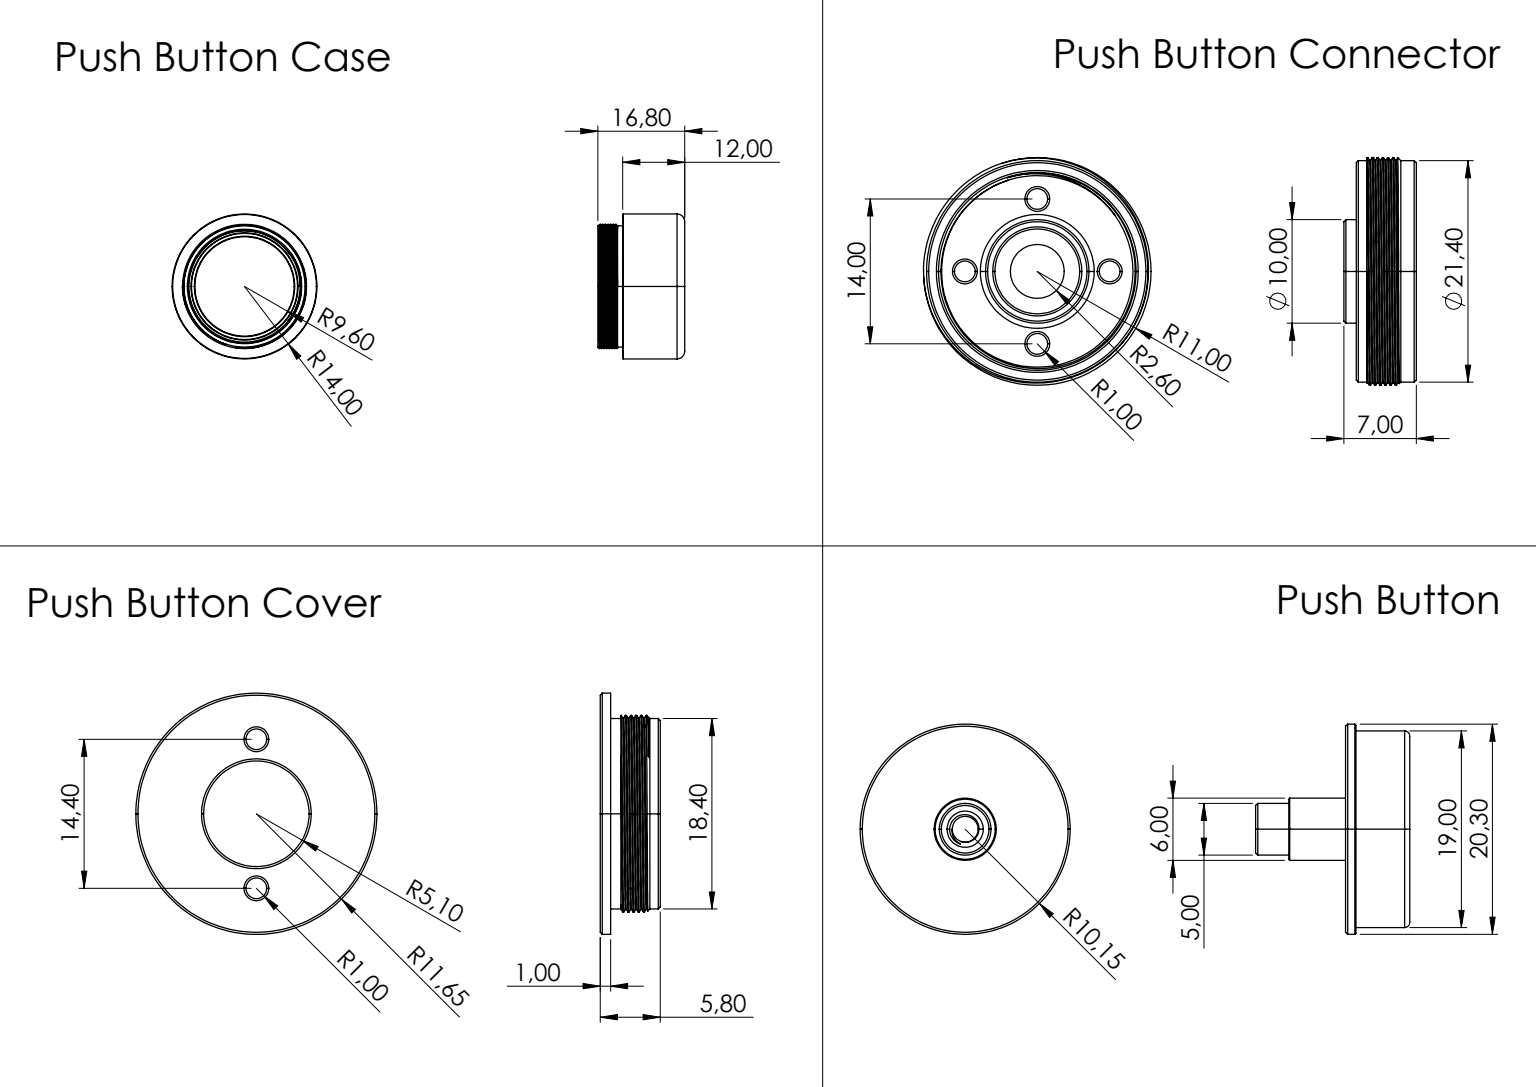
ISO-10303-21;
HEADER;
FILE_DESCRIPTION (('STEP AP214'),
    '1' );
FILE_NAME ('Push Button.step',
    '2026-10-07T19:06:49',
    ( '' ),
    ( '' ),
    'SwSTEP 2.0',
    'SolidWorks 2020',
    '' );
FILE_SCHEMA (( 'AUTOMOTIVE_DESIGN' ));
ENDSEC;

DATA;
#4=CARTESIAN_POINT ( 'NONE',  ( 1.472546342128999930, -80.60010221862999913, -0.7790162248558000213 ) ) ;
#18=CARTESIAN_POINT ( 'NONE',  ( -1.435687946562000272, -77.69186995290999675, 0.2750228405014999988 ) ) ;
#21=CARTESIAN_POINT ( 'NONE',  ( 0.06046471609518229429, -80.22932665438294464, -1.248482646815343600 ) ) ;
#44=CARTESIAN_POINT ( 'NONE',  ( -0.9806565569677715422, -83.04738115356282435, 0.7753017405169410070 ) ) ;
#48=CARTESIAN_POINT ( 'NONE',  ( 1.362316189135000188, -81.60059162671998934, -0.8114345006153000917 ) ) ;
#49=CARTESIAN_POINT ( 'NONE',  ( -1.300896064473999969, -80.54177512065000144, -0.3655689422679000433 ) ) ;
#54=CARTESIAN_POINT ( 'NONE',  ( -1.508789225394999933, -82.23555239048998544, 0.7062677124845000431 ) ) ;
#73=CARTESIAN_POINT ( 'NONE',  ( 0.8787695232493443198, -79.91340179010917666, 0.8885763300944270471 ) ) ;
#78=CARTESIAN_POINT ( 'NONE',  ( -0.5731630996927263855, -81.51327970983244597, 1.110821756836525287 ) ) ;
#88=CARTESIAN_POINT ( 'NONE',  ( -1.250000000000000000, -80.00000000000000000, 0.000000000000000000 ) ) ;
#115=CARTESIAN_POINT ( 'NONE',  ( -1.249999999999999778, -78.01041666666664298, -0.1636246173744686228 ) ) ;
#146=CARTESIAN_POINT ( 'NONE',  ( 0.000000000000000000, -86.20000000000000284, 0.000000000000000000 ) ) ;
#149=B_SPLINE_CURVE_WITH_KNOTS ( 'NONE', 3,
 ( #55404, #38266, #46279, #42423, #24107, #37685, #55701, #15248, #52939, #7198, #42935, #33761, #52652, #47672, #2489, #16927, #57077, #43805 ),
 .UNSPECIFIED., .F., .F.,
 ( 4, 2, 2, 2, 2, 2, 2, 2, 4 ),
 ( 0.000000000000000000, 0.1250000000000000833, 0.2500000000000001110, 0.3750000000000000000, 0.4999999999999999445, 0.6249999999999998890, 0.7499999999999997780, 0.8749999999999998890, 1.000000000000000000 ),
 .UNSPECIFIED. ) ;
#152=CARTESIAN_POINT ( 'NONE',  ( -0.8033051684372000123, -80.29613481679999154, -1.459438184619000101 ) ) ;
#153=CARTESIAN_POINT ( 'NONE',  ( -1.297701781740999927, -78.99170572834999859, -0.6115961818822999163 ) ) ;
#157=DIRECTION ( 'NONE',  ( 0.000000000000000000, -1.000000000000000000, 0.000000000000000000 ) ) ;
#176=CARTESIAN_POINT ( 'NONE',  ( 1.250000000000000000, -78.75000000000000000, 0.000000000000000000 ) ) ;
#186=ORIENTED_EDGE ( 'NONE', *, *, #27821, .T. ) ;
#194=B_SPLINE_CURVE_WITH_KNOTS ( 'NONE', 3,
 ( #52120, #52408, #39679, #34947 ),
 .UNSPECIFIED., .F., .F.,
 ( 4, 4 ),
 ( 0.000000000000000000, 1.000000000000000000 ),
 .UNSPECIFIED. ) ;
#195=CARTESIAN_POINT ( 'NONE',  ( -0.6515920321739999688, -80.16498426945000233, -1.183807013712999900 ) ) ;
#201=LINE ( 'NONE', #48879, #40279 ) ;
#232=DIRECTION ( 'NONE',  ( 0.000000000000000000, -1.000000000000000000, 0.000000000000000000 ) ) ;
#248=CARTESIAN_POINT ( 'NONE',  ( 0.000000000000000000, -80.69999999999998863, -2.899999999999999911 ) ) ;
#273=CARTESIAN_POINT ( 'NONE',  ( 0.1201880509156493942, -80.71773650514016651, 1.541718551563904693 ) ) ;
#282=CARTESIAN_POINT ( 'NONE',  ( 0.000000000000000000, -86.20000000000000284, 0.000000000000000000 ) ) ;
#290=CARTESIAN_POINT ( 'NONE',  ( 0.000000000000000000, -76.75499999999999545, 0.000000000000000000 ) ) ;
#316=CARTESIAN_POINT ( 'NONE',  ( 1.009608792702000102, -77.94743573086999788, -1.302912760256000224 ) ) ;
#319=CARTESIAN_POINT ( 'NONE',  ( 1.156290009273217123, -80.31913236748124518, -0.4746485085928086600 ) ) ;
#320=CARTESIAN_POINT ( 'NONE',  ( 0.3695519436384570033, -77.84114583351794181, -1.371859334843410050 ) ) ;
#333=LINE ( 'NONE', #13274, #40446 ) ;
#342=CARTESIAN_POINT ( 'NONE',  ( 1.349879140156000190, -82.67445575724998719, -0.5781647238538999423 ) ) ;
#345=CARTESIAN_POINT ( 'NONE',  ( -1.217465845835396188, -78.97916666666668561, 0.3271848554490955907 ) ) ;
#362=CARTESIAN_POINT ( 'NONE',  ( -0.2019459281704069076, -77.99218750000888178, 1.256926119276726483 ) ) ;
#368=CARTESIAN_POINT ( 'NONE',  ( -0.5212558242701900157, -81.50950461384270795, 1.136067814103569606 ) ) ;
#370=CYLINDRICAL_SURFACE ( 'NONE', #8132, 1.250000000000000000 ) ;
#371=CARTESIAN_POINT ( 'NONE',  ( -0.9788204679455345669, -81.78049098935534289, 1.151159408688467778 ) ) ;
#388=LINE ( 'NONE', #31625, #21184 ) ;
#402=CARTESIAN_POINT ( 'NONE',  ( -0.9347040216968000026, -78.69407608247999519, 1.332288049216000081 ) ) ;
#442=CARTESIAN_POINT ( 'NONE',  ( 1.520902128651999918, -80.92772696789998577, -0.6797894616744000196 ) ) ;
#443=CARTESIAN_POINT ( 'NONE',  ( 1.082149117140000172, -79.20679688847999955, 1.108446078784000033 ) ) ;
#445=CARTESIAN_POINT ( 'NONE',  ( 0.01073940206318611812, -82.87549824373742524, -1.509945108508129907 ) ) ;
#450=CARTESIAN_POINT ( 'NONE',  ( 0.8593825103163911239, -81.78595333969393266, -0.9078339653130700349 ) ) ;
#478=CARTESIAN_POINT ( 'NONE',  ( -0.5035993198763999423, -79.23880658815998856, -1.271638408173999979 ) ) ;
#513=CARTESIAN_POINT ( 'NONE',  ( -0.7681833999686477066, -82.42708333333332860, 0.9995835529977223910 ) ) ;
#515=VERTEX_POINT ( 'NONE', #57244 ) ;
#555=DIRECTION ( 'NONE',  ( 0.000000000000000000, -1.000000000000000000, 0.000000000000000000 ) ) ;
#565=CARTESIAN_POINT ( 'NONE',  ( -1.511461402894981321, -79.84725243224966107, 0.03864653979242833881 ) ) ;
#573=CARTESIAN_POINT ( 'NONE',  ( -0.5918520097389999846, -82.86672773667999081, -1.596724312065999962 ) ) ;
#595=ORIENTED_EDGE ( 'NONE', *, *, #38393, .T. ) ;
#607=CARTESIAN_POINT ( 'NONE',  ( -1.485771955761999941, -77.72682433276000324, -0.3846555688014000052 ) ) ;
#611=CARTESIAN_POINT ( 'NONE',  ( 0.8048611780553004413, -80.28119307227865420, -0.9591988868156666737 ) ) ;
#613=LINE ( 'NONE', #54606, #57976 ) ;
#632=CARTESIAN_POINT ( 'NONE',  ( 0.6959559787155999988, -82.23218377781998356, 1.424795421937999906 ) ) ;
#634=CARTESIAN_POINT ( 'NONE',  ( -0.1636246173744726473, -79.38541666666664298, 1.249999999999999112 ) ) ;
#663=DIRECTION ( 'NONE',  ( -2.716802477432000171E-13, 0.000000000000000000, 1.000000000000000000 ) ) ;
#673=CIRCLE ( 'NONE', #41223, 10.14999999999999858 ) ;
#686=ORIENTED_EDGE ( 'NONE', *, *, #25485, .T. ) ;
#693=CARTESIAN_POINT ( 'NONE',  ( -0.9347040216968000026, -78.63485975860999133, 1.332288049216000081 ) ) ;
#715=ORIENTED_EDGE ( 'NONE', *, *, #40383, .T. ) ;
#716=DIRECTION ( 'NONE',  ( -1.000000000000000000, 0.000000000000000000, 0.000000000000000000 ) ) ;
#729=CARTESIAN_POINT ( 'NONE',  ( 0.7545134501129999727, -80.60798800110998741, 1.485250302772000097 ) ) ;
#730=CARTESIAN_POINT ( 'NONE',  ( 1.315513048017999953, -78.77661456821999764, 0.1100150488083000005 ) ) ;
#732=CARTESIAN_POINT ( 'NONE',  ( 1.328728262137743421, -81.53943792409916114, 0.7184295318478360892 ) ) ;
#733=CARTESIAN_POINT ( 'NONE',  ( -1.321725462025712616, -83.30889907083121670, 0.7346322590915946860 ) ) ;
#737=CARTESIAN_POINT ( 'NONE',  ( 1.250000000000000000, -81.84999999999999432, 0.000000000000000000 ) ) ;
#741=CARTESIAN_POINT ( 'NONE',  ( 0.9995835529977264988, -80.19791666666665719, -0.7681833999686417114 ) ) ;
#768=CARTESIAN_POINT ( 'NONE',  ( -1.436931233250000162, -79.65986802222998620, -0.3027821832741999786 ) ) ;
#791=DIRECTION ( 'NONE',  ( 0.000000000000000000, -1.000000000000000000, 0.000000000000000000 ) ) ;
#794=DIRECTION ( 'NONE',  ( 0.000000000000000000, -1.000000000000000000, 0.000000000000000000 ) ) ;
#798=CARTESIAN_POINT ( 'NONE',  ( 0.3271848554490964789, -82.35416666666665719, 1.217465845835395521 ) ) ;
#818=B_SPLINE_SURFACE_WITH_KNOTS ( 'NONE', 3, 3, ( 
 ( #39006, #21856, #17146, #8578, #52308, #11864, #12432, #20715, #44020, #25714, #16866, #29841, #57878, #34561, #43740, #3858, #35133, #7424, #26565, #12713, #26288, #8000, #30425, #3572, #34847, #53164, #52878, #25428, #57304, #38715, #52593, #12143, #30131, #48180, #48457 ),
 ( #25997, #21576, #30706, #39581, #48743, #13881, #36609, #54631, #14168, #5322, #4446, #27154, #41337, #4151, #58171, #36896, #22447, #54909, #54, #17737, #18029, #36021, #25219, #43239, #9841, #26576, #58184, #12725, #44610, #35735, #21870, #22164, #35433, #39306, #30717 ),
 ( #4165, #39878, #26008, #34574, #8299, #3305, #53462, #16880, #30437, #40171, #57891, #17447, #48468, #44034, #34861, #39593, #31005, #47909, #8588, #52607, #7441, #25440, #43458, #21013, #39018, #16589, #12157, #30144, #48193, #7726, #32983, #11453, #2595, #25012, #20022 ),
 ( #15871, #33280, #10282, #55444, #14986, #46316, #32692, #6427, #6135, #51320, #15580, #24442, #10878, #38299, #29432, #11170, #29145, #47485, #47191, #51029, #5841, #56605, #42456, #20593, #33575, #43033, #38006, #42162, #24142, #23847, #51614, #19432, #10578, #2024, #56031 ) ),
 .UNSPECIFIED., .F., .F., .F.,
 ( 4, 4 ),
 ( 4, 1, 1, 1, 1, 1, 1, 1, 1, 1, 1, 1, 1, 1, 1, 1, 1, 1, 1, 1, 1, 1, 1, 1, 1, 1, 1, 1, 1, 1, 1, 1, 4 ),
 ( -0.3882448580381000491, 1.388244858038000018 ),
 ( -0.02000000000000000042, 0.01250000000000000069, 0.04499999999999999833, 0.07749999999999999944, 0.1100000000000000006, 0.1424999999999999878, 0.1749999999999999889, 0.2074999999999999900, 0.2399999999999999911, 0.2725000000000000200, 0.3049999999999999933, 0.3375000000000000222, 0.3699999999999999956, 0.4025000000000000244, 0.4349999999999999978, 0.4675000000000000266, 0.5000000000000000000, 0.5324999999999999734, 0.5649999999999999467, 0.5975000000000000311, 0.6300000000000000044, 0.6624999999999999778, 0.6949999999999999512, 0.7275000000000000355, 0.7600000000000000089, 0.7924999999999999822, 0.8249999999999999556, 0.8575000000000000400, 0.8900000000000000133, 0.9224999999999999867, 0.9549999999999999600, 0.9875000000000000444, 1.020000000000000018 ),
 .UNSPECIFIED. ) ;
#820=CARTESIAN_POINT ( 'NONE',  ( 0.8847132563061232968, -82.78824692404089092, -0.8824945250560863874 ) ) ;
#840=CARTESIAN_POINT ( 'NONE',  ( 0.1762382865323051384, -79.63606589178333195, -1.250387681160788134 ) ) ;
#848=CARTESIAN_POINT ( 'NONE',  ( -0.4056890888208716794, -79.74603335400661308, 1.458054600993641259 ) ) ;
#856=CARTESIAN_POINT ( 'NONE',  ( 1.606311393998999915, -82.99304616690000103, -0.5653197666394998988 ) ) ;
#874=CARTESIAN_POINT ( 'NONE',  ( 1.249565383984963862, -80.84028809121133463, -0.1639645281534745924 ) ) ;
#889=CARTESIAN_POINT ( 'NONE',  ( -1.113811846534999983, -78.14627689099999941, 1.056031667973999832 ) ) ;
#894=CARTESIAN_POINT ( 'NONE',  ( -0.8733059116898821417, -80.16394694085556694, -0.8939094887366128006 ) ) ;
#898=CARTESIAN_POINT ( 'NONE',  ( 0.4567011726104230895, -78.99889090922864909, -1.468873967789304125 ) ) ;
#916=CARTESIAN_POINT ( 'NONE',  ( -0.3643839585117999991, -81.91670264959000747, 1.301227969886000091 ) ) ;
#917=CARTESIAN_POINT ( 'NONE',  ( -1.322249586278000155, -80.03650139976998901, -0.2786171024073000324 ) ) ;
#935=CARTESIAN_POINT ( 'NONE',  ( 0.1759108568145950069, -79.23653620316339641, -1.251611073654840034 ) ) ;
#945=CARTESIAN_POINT ( 'NONE',  ( -1.173001147021014212, -81.57218295784426232, 0.4318201719082435108 ) ) ;
#949=CARTESIAN_POINT ( 'NONE',  ( -0.9491653955992001013, -78.01964351345999660, 0.8999264274451000967 ) ) ;
#950=B_SPLINE_CURVE_WITH_KNOTS ( 'NONE', 3,
 ( #46073, #45780, #6184, #14456, #37471, #23607, #15041, #51080, #28612, #20350, #48379, #16211, #43654, #11783, #39207, #57222, #25631, #7630, #34479, #15919, #48098, #25060, #3214, #20919, #33904, #38920, #7060, #47535, #51946, #16787, #56655, #51666, #56938, #38638, #29756, #11503, #30047, #21202, #38060, #29476, #43084, #11213, #3492, #47813, #25918, #16498, #7917, #43358, #2642, #34770, #52510, #12066, #52794, #12349, #38347, #29191, #56081, #7344, #43941, #30336, #15627, #24778, #33622, #47239, #6769, #20635, #42791, #2354, #56368, #34188, #2919, #52226, #25343, #16064, #11355, #29621, #10475, #10775, #29051, #25203, #37617, #46509, #2778, #51511, #28753, #33474, #15186, #38778, #43222, #42644, #2210, #55634, #42058, #47090, #19919, #42356, #15484, #32884, #1924, #29333, #37909, #20777, #14886, #11643, #6034, #55933, #33176 ),
 .UNSPECIFIED., .F., .F.,
 ( 4, 2, 2, 2, 2, 2, 1, 2, 2, 2, 2, 2, 2, 2, 2, 2, 2, 2, 2, 2, 2, 2, 2, 2, 2, 2, 2, 1, 2, 2, 2, 2, 2, 2, 2, 2, 2, 2, 2, 2, 2, 2, 2, 2, 2, 2, 2, 2, 1, 2, 2, 2, 2, 2, 4 ),
 ( 0.000000000000000000, 0.01562500000000001388, 0.03125000000000003469, 0.04687500000000005551, 0.06250000000000008327, 0.07812500000000009714, 0.09375000000000011102, 0.1093750000000001249, 0.1250000000000001388, 0.1406250000000001110, 0.1562500000000001110, 0.1718750000000000833, 0.1875000000000000833, 0.2031250000000000833, 0.2187500000000001110, 0.2343750000000001110, 0.2500000000000001110, 0.2656250000000001110, 0.2812500000000001110, 0.2968750000000001665, 0.3125000000000001665, 0.3281250000000001665, 0.3437500000000001665, 0.3750000000000001665, 0.4062500000000001110, 0.4375000000000001110, 0.4687500000000000555, 0.5000000000000000000, 0.5312500000000000000, 0.5624999999999998890, 0.5937499999999998890, 0.6249999999999997780, 0.6562499999999997780, 0.6718749999999997780, 0.6874999999999997780, 0.7031249999999998890, 0.7187499999999998890, 0.7343749999999998890, 0.7499999999999998890, 0.7656249999999998890, 0.7812499999999998890, 0.7968749999999998890, 0.8124999999999998890, 0.8281250000000000000, 0.8437500000000000000, 0.8593750000000000000, 0.8750000000000000000, 0.8906250000000000000, 0.9062500000000000000, 0.9218750000000000000, 0.9375000000000000000, 0.9531250000000001110, 0.9687500000000001110, 0.9843750000000001110, 1.000000000000000000 ),
 .UNSPECIFIED. ) ;
#959=ORIENTED_EDGE ( 'NONE', *, *, #25485, .F. ) ;
#978=CARTESIAN_POINT ( 'NONE',  ( 0.4326115402657000342, -78.91680236158998696, -1.568920109259999807 ) ) ;
#1016=ADVANCED_FACE ( 'NONE', ( #23425 ), #43407, .T. ) ;
#1018=CARTESIAN_POINT ( 'NONE',  ( -0.8981901762082999952, -79.79086109591999332, -1.403037214508999986 ) ) ;
#1019=CARTESIAN_POINT ( 'NONE',  ( 0.06763567127574998672, -79.64895916143998988, -1.247532485737999908 ) ) ;
#1021=CARTESIAN_POINT ( 'NONE',  ( 0.6046126565052558632, -81.40785622595326743, -1.385375599882785025 ) ) ;
#1026=CARTESIAN_POINT ( 'NONE',  ( -0.8193159871064622513, -81.66856760969551488, -0.9439107478074511004 ) ) ;
#1027=( NAMED_UNIT ( * ) SI_UNIT ( $, .STERADIAN. ) SOLID_ANGLE_UNIT ( ) );
#1048=AXIS2_PLACEMENT_3D ( 'NONE', #52317, #57594, #33995 ) ;
#1053=CARTESIAN_POINT ( 'NONE',  ( 0.6229729438976999711, -81.04952822830999537, 1.458184003450999855 ) ) ;
#1064=CARTESIAN_POINT ( 'NONE',  ( -1.250000000000000000, -79.00000000000000000, 0.000000000000000000 ) ) ;
#1087=CARTESIAN_POINT ( 'NONE',  ( -1.092232985442822102, -82.54166666666664298, -0.6295237254636245616 ) ) ;
#1093=ORIENTED_EDGE ( 'NONE', *, *, #15590, .T. ) ;
#1107=CARTESIAN_POINT ( 'NONE',  ( 1.228744581380641687, -82.83562427784806914, -0.2287525698557267839 ) ) ;
#1126=CARTESIAN_POINT ( 'NONE',  ( -0.4851089960429650905, -83.00678479282305489, 1.152015161174709146 ) ) ;
#1133=CARTESIAN_POINT ( 'NONE',  ( 0.1624548541070857943, -79.48286375057362818, -1.504788102669172734 ) ) ;
#1180=CARTESIAN_POINT ( 'NONE',  ( -1.190204951956445267, -80.12538959866201083, -0.3913796594779095916 ) ) ;
#1184=CARTESIAN_POINT ( 'NONE',  ( -0.7887420553019258707, -78.26716755245251989, 1.320791577295096442 ) ) ;
#1194=DIRECTION ( 'NONE',  ( -1.000000000000000000, 0.000000000000000000, 0.000000000000000000 ) ) ;
#1199=CARTESIAN_POINT ( 'NONE',  ( 0.4274279416557000277, -83.36936459712099179, 1.281884980902999960 ) ) ;
#1209=CARTESIAN_POINT ( 'NONE',  ( -1.288646058034000008, -83.05573296103600001, 0.4058063692239000098 ) ) ;
#1212=CARTESIAN_POINT ( 'NONE',  ( 1.343749999883000035, -77.90625000011999646, 3.156563468101999814E-09 ) ) ;
#1220=CARTESIAN_POINT ( 'NONE',  ( 1.062167859419960614, -79.30478719906479057, -0.6841706396682687430 ) ) ;
#1225=CARTESIAN_POINT ( 'NONE',  ( -2.299999999264999762, -77.49999999927000260, -2.080610052828999912E-10 ) ) ;
#1229=CARTESIAN_POINT ( 'NONE',  ( -1.143190144809757669, -81.56692634864619151, 0.5063306831769307514 ) ) ;
#1234=CARTESIAN_POINT ( 'NONE',  ( -1.280405559996000031, -78.59639078104000021, -0.2671032044805999872 ) ) ;
#1263=CARTESIAN_POINT ( 'NONE',  ( 1.341343219651000229, -78.97248393136999312, -0.9216622887798999741 ) ) ;
#1271=CARTESIAN_POINT ( 'NONE',  ( -0.9334586162929999764, -81.40447863951000329, -1.282259494539000011 ) ) ;
#1298=CARTESIAN_POINT ( 'NONE',  ( 1.640574411872000038, -79.59349766811000393, 0.2893137654249999802 ) ) ;
#1301=CARTESIAN_POINT ( 'NONE',  ( -0.1061383120418225301, -81.63053294589249731, 1.507463295298500761 ) ) ;
#1309=CARTESIAN_POINT ( 'NONE',  ( -0.5392730711932351984, -81.68971611294774959, -1.130938875651418929 ) ) ;
#1319=CARTESIAN_POINT ( 'NONE',  ( -1.447950951198242908, -77.76302083339091098, -0.3900009942188623069 ) ) ;
#1335=CARTESIAN_POINT ( 'NONE',  ( -1.125831293927000099, -79.53339211834999389, 0.7473110439769999891 ) ) ;
#1390=CARTESIAN_POINT ( 'NONE',  ( 1.179782483562120010, -82.82318035081991070, -0.4135125750267664158 ) ) ;
#1410=DIRECTION ( 'NONE',  ( 0.000000000000000000, -1.000000000000000000, 0.000000000000000000 ) ) ;
#1415=CARTESIAN_POINT ( 'NONE',  ( 1.136635571591867233, -82.88416972722252751, 0.5202534302794125098 ) ) ;
#1417=DIRECTION ( 'NONE',  ( -1.000000000000000000, 0.000000000000000000, 0.000000000000000000 ) ) ;
#1421=CONICAL_SURFACE ( 'NONE', #16485, 1.546875000130000011, 0.7853981633972997312 ) ;
#1450=CARTESIAN_POINT ( 'NONE',  ( -0.2327570447753271599, -80.71078059628793255, -1.249194938801351462 ) ) ;
#1469=CARTESIAN_POINT ( 'NONE',  ( -0.4548846362379543873, -80.19556477582571574, -1.164187075856578879 ) ) ;
#1473=CARTESIAN_POINT ( 'NONE',  ( 0.7757320150892573762, -78.51702430842580327, -1.327015570253983867 ) ) ;
#1475=VERTEX_POINT ( 'NONE', #10794 ) ;
#1491=CARTESIAN_POINT ( 'NONE',  ( -0.3271848554491046945, -78.89583333333328596, 1.217465845835393301 ) ) ;
#1515=CARTESIAN_POINT ( 'NONE',  ( 1.137232763453390971, -81.38436038258944905, 0.5186267222472648042 ) ) ;
#1547=CARTESIAN_POINT ( 'NONE',  ( -0.6580604922749000441, -79.48068756757000131, -1.488334326434000099 ) ) ;
#1555=CARTESIAN_POINT ( 'NONE',  ( -1.478021081765000133, -80.28866583923000633, 0.8457367421919999018 ) ) ;
#1586=CARTESIAN_POINT ( 'NONE',  ( 1.520902128651999918, -81.04615961563999349, -0.6797894616744000196 ) ) ;
#1587=CARTESIAN_POINT ( 'NONE',  ( -0.7899273271878000102, -77.87807433275999358, 1.197381041534999913 ) ) ;
#1592=CARTESIAN_POINT ( 'NONE',  ( 1.008924559857650838, -79.79982627189708921, -0.7395781483535016632 ) ) ;
#1595=CARTESIAN_POINT ( 'NONE',  ( -0.6881529071261847097, -81.67893781361996730, -1.045368128735210345 ) ) ;
#1598=EDGE_LOOP ( 'NONE', ( #30301, #26182, #32852, #20081 ) ) ;
#1605=DIRECTION ( 'NONE',  ( 0.000000000000000000, 1.000000000000000000, 0.000000000000000000 ) ) ;
#1625=CARTESIAN_POINT ( 'NONE',  ( -0.4634070002434999558, -79.17548989939000137, -1.170148800580000037 ) ) ;
#1646=CARTESIAN_POINT ( 'NONE',  ( 0.1128515190273495367, -78.46792679642489077, 1.249931857778512345 ) ) ;
#1651=ADVANCED_FACE ( 'NONE', ( #6935 ), #57395, .F. ) ;
#1668=CARTESIAN_POINT ( 'NONE',  ( 0.7677661701836960839, -78.27713689064573543, -0.9989898656190768778 ) ) ;
#1669=CARTESIAN_POINT ( 'NONE',  ( 0.000000000000000000, -87.15000000002500258, 0.000000000000000000 ) ) ;
#1683=ORIENTED_EDGE ( 'NONE', *, *, #42399, .F. ) ;
#1684=CARTESIAN_POINT ( 'NONE',  ( -1.249681228189473803, -79.59559394467255800, 0.07758196913156252539 ) ) ;
#1685=CARTESIAN_POINT ( 'NONE',  ( -0.6712347860653230525, -78.16172226271685020, 1.350201467282728274 ) ) ;
#1703=CARTESIAN_POINT ( 'NONE',  ( 0.4639973262319513347, -82.94477574862143854, 1.160677889351085623 ) ) ;
#1715=CARTESIAN_POINT ( 'NONE',  ( 1.092232985442823212, -80.70833333333331439, -0.6295237254636224522 ) ) ;
#1745=CARTESIAN_POINT ( 'NONE',  ( -1.009397235748368260, -81.20718188826208461, -0.8706472256294847112 ) ) ;
#1760=CARTESIAN_POINT ( 'NONE',  ( -0.5573453952815472512, -80.18842898730592594, -1.122125656035228625 ) ) ;
#1764=CARTESIAN_POINT ( 'NONE',  ( 1.505383061368419151, -79.10597237606836529, 0.1212336400873940262 ) ) ;
#1779=CARTESIAN_POINT ( 'NONE',  ( -0.6142531002814000107, -83.43252381223099690, 1.203711489715000305 ) ) ;
#1789=CARTESIAN_POINT ( 'NONE',  ( -0.5525270872808000222, -82.17150394948998837, -1.233160589678000019 ) ) ;
#1791=ADVANCED_FACE ( 'NONE', ( #35516 ), #44242, .T. ) ;
#1808=CARTESIAN_POINT ( 'NONE',  ( 0.9748194815771379362, -81.40464457030101642, 0.7859197306878139555 ) ) ;
#1813=CARTESIAN_POINT ( 'NONE',  ( 0.05227849266716000365, -79.20809242846999609, -1.244609249457999889 ) ) ;
#1843=CARTESIAN_POINT ( 'NONE',  ( -0.06603165175717734536, -81.62109302337999850, -1.273657571949194489 ) ) ;
#1844=CARTESIAN_POINT ( 'NONE',  ( 0.1660104325307999729, -78.25569303241999819, 1.618982269915999916 ) ) ;
#1852=FACE_OUTER_BOUND ( 'NONE', #12679, .T. ) ;
#1864=ORIENTED_EDGE ( 'NONE', *, *, #30051, .T. ) ;
#1877=CARTESIAN_POINT ( 'NONE',  ( -0.4900037880837543325, -80.00730615406503432, 1.149793150307434342 ) ) ;
#1881=EDGE_CURVE ( 'NONE', #7116, #37205, #34789, .T. ) ;
#1883=CARTESIAN_POINT ( 'NONE',  ( 1.417725061834000044, -79.97639585000999318, -0.8748226493128999914 ) ) ;
#1884=CARTESIAN_POINT ( 'NONE',  ( -1.375650254229000113, -77.93375590253999974, 0.4072090767667999600 ) ) ;
#1886=CARTESIAN_POINT ( 'NONE',  ( 1.076979181859827106, -81.43822123321770334, -1.059161443897362664 ) ) ;
#1888=LINE ( 'NONE', #10740, #54428 ) ;
#1893=CARTESIAN_POINT ( 'NONE',  ( -0.4068589336182526495, -81.69886620421327450, -1.181800740598763166 ) ) ;
#1896=CARTESIAN_POINT ( 'NONE',  ( -1.249999999999999778, -80.01041666666664298, -0.1636246173744686228 ) ) ;
#1903=CARTESIAN_POINT ( 'NONE',  ( 1.250000000000000000, -80.74999999999998579, 0.000000000000000000 ) ) ;
#1908=CARTESIAN_POINT ( 'NONE',  ( 1.343749999883000035, -77.90625000011999646, 3.156563468101999814E-09 ) ) ;
#1920=CARTESIAN_POINT ( 'NONE',  ( 1.676986109946000170, -79.53386453932999700, 0.2957349343760000138 ) ) ;
#1924=CARTESIAN_POINT ( 'NONE',  ( 1.434073767539737476, -79.47461743011145074, -0.4734074842604066302 ) ) ;
#1940=CARTESIAN_POINT ( 'NONE',  ( 0.7924526256690966886, -78.42054099154100300, 0.9668092435737775103 ) ) ;
#1966=DIRECTION ( 'NONE',  ( 1.040437577282999923E-11, 1.000000000000000000, -2.038011343141999906E-09 ) ) ;
#1978=CARTESIAN_POINT ( 'NONE',  ( -0.6292794791536331367, -82.68371027185608568, -1.092639821175960479 ) ) ;
#1979=ORIENTED_EDGE ( 'NONE', *, *, #58164, .T. ) ;
#1983=CARTESIAN_POINT ( 'NONE',  ( 0.7149329466314869874, -78.08609980630498626, 1.354438294650810892 ) ) ;
#2002=CARTESIAN_POINT ( 'NONE',  ( 0.9590251478797268136, -82.90587166377093808, 0.8014916951292889724 ) ) ;
#2024=CARTESIAN_POINT ( 'NONE',  ( -1.374853770045000090, -81.42764988327999731, -0.7192078502473999713 ) ) ;
#2041=CARTESIAN_POINT ( 'NONE',  ( -0.04600636030614828342, -80.47847291610720788, 1.248880407862982711 ) ) ;
#2058=CARTESIAN_POINT ( 'NONE',  ( -1.279096942007310611, -78.80257488668075894, 0.8515545081673395744 ) ) ;
#2071=CARTESIAN_POINT ( 'NONE',  ( -0.6329778402533998705, -82.10618029491999437, -1.193863583722999833 ) ) ;
#2099=CARTESIAN_POINT ( 'NONE',  ( -0.003982218678106667215, -81.47577399763491712, 1.249684034757714279 ) ) ;
#2101=CARTESIAN_POINT ( 'NONE',  ( 1.093387357835452933, -82.30899171049304641, -0.6298603018139183884 ) ) ;
#2103=CARTESIAN_POINT ( 'NONE',  ( 0.0004826309679763999953, -77.70505409477999592, -1.307959744758000031 ) ) ;
#2107=ORIENTED_EDGE ( 'NONE', *, *, #50023, .T. ) ;
#2108=ORIENTED_EDGE ( 'NONE', *, *, #13353, .T. ) ;
#2130=CARTESIAN_POINT ( 'NONE',  ( 0.08338359222296000406, -79.51780861409000067, -1.538001148114999994 ) ) ;
#2139=CARTESIAN_POINT ( 'NONE',  ( 1.653747448240000084, -80.09918819389999101, 0.4061235413877000155 ) ) ;
#2166=CARTESIAN_POINT ( 'NONE',  ( -0.9620943986040956242, -80.04521171774420907, 0.7983770923343646020 ) ) ;
#2172=FACE_OUTER_BOUND ( 'NONE', #45792, .T. ) ;
#2174=CARTESIAN_POINT ( 'NONE',  ( 1.052209778380920779, -83.03560755957414585, -1.084595603600321256 ) ) ;
#2175=CARTESIAN_POINT ( 'NONE',  ( -1.249989095222701962, -79.61143095040115725, -0.1792705600110044706 ) ) ;
#2178=CARTESIAN_POINT ( 'NONE',  ( -0.7575910999740240737, -81.67355912156841669, -0.9946733871216205669 ) ) ;
#2180=( LENGTH_UNIT ( ) NAMED_UNIT ( * ) SI_UNIT ( .MILLI., .METRE. ) );
#2195=DIRECTION ( 'NONE',  ( 0.7071067811865474617, 0.7071067811865474617, -7.240421654463485624E-10 ) ) ;
#2198=ORIENTED_EDGE ( 'NONE', *, *, #38015, .F. ) ;
#2204=CARTESIAN_POINT ( 'NONE',  ( 1.217465845835393967, -79.77083333333330017, 0.3271848554491025851 ) ) ;
#2206=CARTESIAN_POINT ( 'NONE',  ( 0.8102226603197999477, -80.03898078654999892, 1.363061245571999924 ) ) ;
#2210=CARTESIAN_POINT ( 'NONE',  ( 0.1655257079421880717, -79.61632079734550871, 1.501053824981346763 ) ) ;
#2214=LINE ( 'NONE', #38204, #7077 ) ;
#2224=CARTESIAN_POINT ( 'NONE',  ( 0.8397211166896187962, -78.41649201275657788, 0.9258721447709178376 ) ) ;
#2245=CARTESIAN_POINT ( 'NONE',  ( 0.000000000000000000, -77.69999999999998863, 0.000000000000000000 ) ) ;
#2259=CARTESIAN_POINT ( 'NONE',  ( 0.4467594448287516284, -82.75414052523781550, -1.167571400202662035 ) ) ;
#2264=CARTESIAN_POINT ( 'NONE',  ( 0.6359740846337066378, -79.43277818229616116, 1.079437290100915048 ) ) ;
#2265=CARTESIAN_POINT ( 'NONE',  ( -1.002309790681787716, -78.81711688494529255, -1.125562765835532497 ) ) ;
#2274=CARTESIAN_POINT ( 'NONE',  ( 0.9062719787061290777, -81.17322235724128632, 1.209793186763744366 ) ) ;
#2285=CARTESIAN_POINT ( 'NONE',  ( 0.2266372662724759901, -82.96071876721104843, 1.229146615866300696 ) ) ;
#2293=DIRECTION ( 'NONE',  ( 0.000000000000000000, 1.000000000000000000, 0.000000000000000000 ) ) ;
#2319=FACE_OUTER_BOUND ( 'NONE', #35834, .T. ) ;
#2325=CARTESIAN_POINT ( 'NONE',  ( -0.02507988100666198525, -80.47717407346517859, 1.249410415426445153 ) ) ;
#2328=CIRCLE ( 'NONE', #34322, 9.500000000000000000 ) ;
#2332=ORIENTED_EDGE ( 'NONE', *, *, #19355, .T. ) ;
#2341=CARTESIAN_POINT ( 'NONE',  ( -1.478853428237032475, -77.86561205178121270, -0.3007429780463568014 ) ) ;
#2342=ADVANCED_FACE ( 'NONE', ( #58194 ), #8600, .F. ) ;
#2354=CARTESIAN_POINT ( 'NONE',  ( 1.329440977735876661, -79.96045754634249647, -0.7203538468090995295 ) ) ;
#2384=CARTESIAN_POINT ( 'NONE',  ( 1.146081193082048033, -81.38292660934976652, 0.4986479518160068514 ) ) ;
#2392=ORIENTED_EDGE ( 'NONE', *, *, #3092, .T. ) ;
#2406=ORIENTED_EDGE ( 'NONE', *, *, #22775, .F. ) ;
#2415=CARTESIAN_POINT ( 'NONE',  ( 0.1742577344548000007, -77.75455890439999962, 1.489843697164999980 ) ) ;
#2422=CARTESIAN_POINT ( 'NONE',  ( -1.586699731716999962, -82.80045924015399805, 0.6182239771991999699 ) ) ;
#2423=CARTESIAN_POINT ( 'NONE',  ( -1.639384890095999969, -80.35182505433999722, -0.4606887641594999971 ) ) ;
#2431=CARTESIAN_POINT ( 'NONE',  ( -0.8302729325563608098, -81.16825566421603355, -0.9509483969845207163 ) ) ;
#2458=CARTESIAN_POINT ( 'NONE',  ( -0.1835247799291997717, -82.96475420480349783, -1.500792295550013478 ) ) ;
#2488=CARTESIAN_POINT ( 'NONE',  ( -0.9334586162929999764, -81.34442870581999330, -1.282259494539000011 ) ) ;
#2489=CARTESIAN_POINT ( 'NONE',  ( -1.092232985442822102, -81.04166666666664298, -0.6295237254636245616 ) ) ;
#2528=FACE_BOUND ( 'NONE', #24499, .T. ) ;
#2530=CARTESIAN_POINT ( 'NONE',  ( -0.3271848554491046945, -81.89583333333330017, 1.217465845835393301 ) ) ;
#2544=CARTESIAN_POINT ( 'NONE',  ( 0.7945685312060931649, -82.78032265392057809, -0.9647621081858361869 ) ) ;
#2548=CARTESIAN_POINT ( 'NONE',  ( 0.8360307752442982521, -79.41690561761365075, 0.9295092197899607056 ) ) ;
#2549=CARTESIAN_POINT ( 'NONE',  ( -0.9591330678447479441, -78.32136967069745026, -1.194087134926961946 ) ) ;
#2558=CARTESIAN_POINT ( 'NONE',  ( -1.480668258985768482, -81.36553860590423426, -0.3070248522480592546 ) ) ;
#2595=CARTESIAN_POINT ( 'NONE',  ( -0.8762103189736000219, -81.41053970282000307, -1.416501064863000092 ) ) ;
#2607=ORIENTED_EDGE ( 'NONE', *, *, #55721, .F. ) ;
#2611=EDGE_LOOP ( 'NONE', ( #45072, #3068, #21608, #2789, #31112, #29819 ) ) ;
#2612=CARTESIAN_POINT ( 'NONE',  ( -0.06320921880059908460, -80.47953876087936465, 1.248225759446036864 ) ) ;
#2629=CARTESIAN_POINT ( 'NONE',  ( -1.250000000000000000, -83.09999999999999432, 0.000000000000000000 ) ) ;
#2642=CARTESIAN_POINT ( 'NONE',  ( 1.545086291967713299, -80.49690600801427820, -0.05127199417640600221 ) ) ;
#2652=CARTESIAN_POINT ( 'NONE',  ( 0.6735630312197999903, -82.86657026302199824, -1.435516540950999786 ) ) ;
#2670=CARTESIAN_POINT ( 'NONE',  ( 0.6793202165550557003, -81.42948271688828754, 1.050371840538202539 ) ) ;
#2673=CARTESIAN_POINT ( 'NONE',  ( 0.000000000000000000, -87.15000000002500258, 0.000000000000000000 ) ) ;
#2706=DIRECTION ( 'NONE',  ( -1.000000000000000000, 0.000000000000000000, 0.000000000000000000 ) ) ;
#2707=CARTESIAN_POINT ( 'NONE',  ( -1.566959183383000109, -78.36705617198001050, 0.4396611996733000294 ) ) ;
#2713=CARTESIAN_POINT ( 'NONE',  ( 0.4046438523804999909, -81.47411572283999703, -1.654233492563000008 ) ) ;
#2714=CARTESIAN_POINT ( 'NONE',  ( -0.7407245532275998912, -81.59442870581999330, -1.017507444502999903 ) ) ;
#2733=CARTESIAN_POINT ( 'NONE',  ( -1.440962122118119471, -79.37367604318139058, -0.4505052090234867301 ) ) ;
#2739=CARTESIAN_POINT ( 'NONE',  ( -1.250000000000000000, -80.09999999999999432, 0.000000000000000000 ) ) ;
#2745=CARTESIAN_POINT ( 'NONE',  ( 0.4264742922811849413, -82.70158460137095346, 1.451405935591948637 ) ) ;
#2746=CARTESIAN_POINT ( 'NONE',  ( -0.9383909286133819139, -79.65811737660978054, -0.8288992896692728429 ) ) ;
#2754=ORIENTED_EDGE ( 'NONE', *, *, #48627, .T. ) ;
#2755=VERTEX_POINT ( 'NONE', #44119 ) ;
#2776=CARTESIAN_POINT ( 'NONE',  ( -1.526555281555000088, -80.22845843187998582, -0.4289821568622999570 ) ) ;
#2778=CARTESIAN_POINT ( 'NONE',  ( -1.492020074518721318, -79.73778082640328080, 0.2322189972777134459 ) ) ;
#2789=ORIENTED_EDGE ( 'NONE', *, *, #23705, .F. ) ;
#2798=AXIS2_PLACEMENT_3D ( 'NONE', #33784, #43246, #16954 ) ;
#2810=CARTESIAN_POINT ( 'NONE',  ( 1.357547920874000003, -78.53098293213999170, -0.9615626969474000418 ) ) ;
#2818=CARTESIAN_POINT ( 'NONE',  ( 0.9995835529977233902, -81.80208333333332860, 0.7681833999686461523 ) ) ;
#2834=CARTESIAN_POINT ( 'NONE',  ( -0.2254326743809463296, -78.13651477724624783, 1.514863696781568736 ) ) ;
#2891=CARTESIAN_POINT ( 'NONE',  ( -0.01891664938484899361, -80.47679111333721380, 1.249509389969930773 ) ) ;
#2911=VECTOR ( 'NONE', #51281, 1000.000000000000000 ) ;
#2919=CARTESIAN_POINT ( 'NONE',  ( 0.8074256036998892494, -79.91997086998991051, -1.276157013251583150 ) ) ;
#2928=CARTESIAN_POINT ( 'NONE',  ( 1.420454834158999979, -81.41375084182999444, 0.3724989704330000095 ) ) ;
#2947=CARTESIAN_POINT ( 'NONE',  ( -0.8033051684372000123, -80.41456746453999926, -1.459438184619000101 ) ) ;
#2951=CARTESIAN_POINT ( 'NONE',  ( -0.6299849389810197042, -82.18398283962009998, -1.093434970869878287 ) ) ;
#2988=DIRECTION ( 'NONE',  ( 1.000000000000000000, 0.000000000000000000, 2.719057617949999588E-13 ) ) ;
#2991=CARTESIAN_POINT ( 'NONE',  ( 9.500000000000000000, -91.89999999999999147, 0.000000000000000000 ) ) ;
#2997=CARTESIAN_POINT ( 'NONE',  ( -1.544355253863999966, -83.34783910444198796, -0.3612495668209000366 ) ) ;
#2999=CARTESIAN_POINT ( 'NONE',  ( 1.446151133417000079, -79.72054785055999560, 0.2550274018384999786 ) ) ;
#3008=CARTESIAN_POINT ( 'NONE',  ( -0.2863152943028942077, -81.20653045236295497, -1.221378511987871951 ) ) ;
#3013=DIRECTION ( 'NONE',  ( 0.000000000000000000, -1.000000000000000000, 0.000000000000000000 ) ) ;
#3025=CARTESIAN_POINT ( 'NONE',  ( -1.190683053189752982, -80.07578141901581148, 0.3803500925840294089 ) ) ;
#3033=CARTESIAN_POINT ( 'NONE',  ( 1.270967135966797112, -82.05378250061171741, -0.8204115018237847501 ) ) ;
#3034=CARTESIAN_POINT ( 'NONE',  ( 0.4820167300484242690, -79.75682355617291819, -1.153123235814610181 ) ) ;
#3050=SHAPE_DEFINITION_REPRESENTATION ( #24909, #33899 ) ;
#3065=CARTESIAN_POINT ( 'NONE',  ( 1.291435174072999903, -79.40738863544999049, -0.9202965842325999679 ) ) ;
#3068=ORIENTED_EDGE ( 'NONE', *, *, #54755, .F. ) ;
#3092=EDGE_CURVE ( 'NONE', #26509, #39544, #52050, .T. ) ;
#3100=CARTESIAN_POINT ( 'NONE',  ( 1.249653476780883121, -81.85243642884611859, 0.02917368571513033818 ) ) ;
#3127=CARTESIAN_POINT ( 'NONE',  ( 0.3860122406418020624, -82.75015049869273298, -1.188808172101050165 ) ) ;
#3138=CARTESIAN_POINT ( 'NONE',  ( -1.260603054430202263, -81.39590432937541209, -0.8352852932649793560 ) ) ;
#3148=CARTESIAN_POINT ( 'NONE',  ( 1.251003419626117052, -82.85390030615222656, 0.05208032629560303828 ) ) ;
#3154=DIRECTION ( 'NONE',  ( 0.000000000000000000, 1.000000000000000000, 0.000000000000000000 ) ) ;
#3188=CARTESIAN_POINT ( 'NONE',  ( 0.3239878837106308085, -80.45445633517968531, 1.207198879959141102 ) ) ;
#3207=CARTESIAN_POINT ( 'NONE',  ( -1.092232985442824100, -83.45833333333328596, 0.6295237254636200097 ) ) ;
#3214=CARTESIAN_POINT ( 'NONE',  ( 1.348353453518538192, -80.96250278606902384, -0.6851815357594489564 ) ) ;
#3224=CARTESIAN_POINT ( 'NONE',  ( -0.6256353049379000941, -82.61393340258099727, 1.457043991488000012 ) ) ;
#3227=CARTESIAN_POINT ( 'NONE',  ( -1.249999999999999778, -82.01041666666662877, -0.1636246173744686228 ) ) ;
#3237=CARTESIAN_POINT ( 'NONE',  ( 0.000000000000000000, -87.20000000000000284, 0.000000000000000000 ) ) ;
#3243=CARTESIAN_POINT ( 'NONE',  ( 0.8512149552595998925, -80.16193060409999305, 1.432023780608000063 ) ) ;
#3274=CARTESIAN_POINT ( 'NONE',  ( 1.092232985442823212, -83.20833333333330017, -0.6295237254636224522 ) ) ;
#3280=CARTESIAN_POINT ( 'NONE',  ( -1.250000000000000000, -79.10000000000000853, 0.000000000000000000 ) ) ;
#3282=CARTESIAN_POINT ( 'NONE',  ( 0.000000000000000000, -91.89999999999999147, 0.000000000000000000 ) ) ;
#3287=CARTESIAN_POINT ( 'NONE',  ( -1.438065998794000100, -83.41115579321099460, -0.3363867981957999742 ) ) ;
#3288=CARTESIAN_POINT ( 'NONE',  ( 0.4542139134408000323, -80.54146017332999463, -1.519238769708999959 ) ) ;
#3305=CARTESIAN_POINT ( 'NONE',  ( 1.496210884224999926, -83.11583851079198837, 0.7325374182646999799 ) ) ;
#3313=CARTESIAN_POINT ( 'NONE',  ( 1.105138191744446718, -79.88914713198865059, 0.5837908578609295462 ) ) ;
#3316=ADVANCED_FACE ( 'NONE', ( #53478 ), #370, .F. ) ;
#3318=CARTESIAN_POINT ( 'NONE',  ( -0.3273215601811345077, -78.99604344152334079, 1.250887209240275633 ) ) ;
#3319=CARTESIAN_POINT ( 'NONE',  ( 1.520202006809699524, -82.11451394755752631, 0.3017852963696689428 ) ) ;
#3320=CARTESIAN_POINT ( 'NONE',  ( 0.01229450786555221289, -79.72617763684984027, -1.249719495759485710 ) ) ;
#3366=DIRECTION ( 'NONE',  ( 0.000000000000000000, 1.000000000000000000, 0.000000000000000000 ) ) ;
#3385=CARTESIAN_POINT ( 'NONE',  ( 1.181146588278086940, -81.87666702745578107, 0.4112698556210559464 ) ) ;
#3409=EDGE_LOOP ( 'NONE', ( #34555, #30308, #2392, #27625 ) ) ;
#3421=CARTESIAN_POINT ( 'NONE',  ( 0.3870708775265000456, -80.22814348455999323, -1.294661097694999929 ) ) ;
#3466=EDGE_LOOP ( 'NONE', ( #43905, #24684, #12476, #4857, #49366, #30018, #49439 ) ) ;
#3490=CARTESIAN_POINT ( 'NONE',  ( 0.7681833999686451531, -78.67708333333332860, -0.9995835529977240563 ) ) ;
#3492=CARTESIAN_POINT ( 'NONE',  ( -0.6245939647354400437, -80.65885271342463625, 1.376621695022554936 ) ) ;
#3502=CARTESIAN_POINT ( 'NONE',  ( 0.3489451476548999787, -81.28743241160998423, -1.426530384489999914 ) ) ;
#3563=CARTESIAN_POINT ( 'NONE',  ( -0.8845133210371012300, -83.03823067849943129, 0.8826922710338861444 ) ) ;
#3567=CARTESIAN_POINT ( 'NONE',  ( -0.5667803598935999831, -82.23202630415998726, 1.605794812195000087 ) ) ;
#3568=CARTESIAN_POINT ( 'NONE',  ( -1.413725673013999984, -80.47845843187998582, -0.3972755495651000279 ) ) ;
#3572=CARTESIAN_POINT ( 'NONE',  ( 0.5021253177900999454, -81.86053999106999868, -1.588436081161999969 ) ) ;
#3589=CARTESIAN_POINT ( 'NONE',  ( 0.0004189892803136687979, -77.98437500001877254, 1.281334813302893005 ) ) ;
#3592=CARTESIAN_POINT ( 'NONE',  ( 1.072822471686033063, -79.89348443873119265, 0.6422160631042705958 ) ) ;
#3610=EDGE_CURVE ( 'NONE', #7212, #44932, #20964, .T. ) ;
#3615=B_SPLINE_CURVE_WITH_KNOTS ( 'NONE', 3,
 ( #7457, #38161, #25167, #16893, #3318, #25455, #34875, #57046, #20173, #56184, #56471, #56763, #11315, #6872 ),
 .UNSPECIFIED., .F., .F.,
 ( 4, 2, 2, 2, 2, 2, 4 ),
 ( 0.000000000000000000, 0.2500000000000000000, 0.5000000000000000000, 0.6250000000000000000, 0.7500000000000000000, 0.8750000000000000000, 1.000000000000000000 ),
 .UNSPECIFIED. ) ;
#3626=CARTESIAN_POINT ( 'NONE',  ( 0.4326115402657000342, -78.85758603771999731, -1.568920109259999807 ) ) ;
#3666=CARTESIAN_POINT ( 'NONE',  ( 1.036471533130701506, -81.89769297308482976, 0.7000341817469545314 ) ) ;
#3667=CARTESIAN_POINT ( 'NONE',  ( 1.541711259781999743, -79.15111531869999340, 0.1510856428486999914 ) ) ;
#3675=CARTESIAN_POINT ( 'NONE',  ( -1.250000000000001332, -81.98958333333334281, 0.1636246173744632659 ) ) ;
#3682=VERTEX_POINT ( 'NONE', #6800 ) ;
#3691=ORIENTED_EDGE ( 'NONE', *, *, #16360, .F. ) ;
#3695=DIRECTION ( 'NONE',  ( 1.000000000000000000, 0.000000000000000000, 0.000000000000000000 ) ) ;
#3726=ORIENTED_EDGE ( 'NONE', *, *, #52233, .F. ) ;
#3748=EDGE_LOOP ( 'NONE', ( #37219, #7609 ) ) ;
#3769=CARTESIAN_POINT ( 'NONE',  ( 0.9995835529977233902, -83.30208333333332860, 0.7681833999686461523 ) ) ;
#3774=CARTESIAN_POINT ( 'NONE',  ( 1.082313248930284022, -80.53554216430265456, -1.106039928096046898 ) ) ;
#3787=CARTESIAN_POINT ( 'NONE',  ( 1.392666586335999934, -81.91902456270999267, 0.4657552147452999614 ) ) ;
#3801=DIRECTION ( 'NONE',  ( 0.000000000000000000, 0.000000000000000000, -1.000000000000000000 ) ) ;
#3806=CARTESIAN_POINT ( 'NONE',  ( -1.445929428138999828, -80.34746535818999291, 0.8273736140038000508 ) ) ;
#3811=PLANE ( 'NONE',  #19518 ) ;
#3812=B_SPLINE_CURVE_WITH_KNOTS ( 'NONE', 3,
 ( #14647, #1684, #50694, #19674, #37674, #55692, #38255, #57926, #24688, #11699, #4201, #49075, #7547, #52140, #53498, #25547, #56278, #31039, #21903, #17483, #16411, #34100, #56561, #29675, #47148, #16122, #43565, #47725, #52426, #2264, #29963, #58220, #11985, #2548, #35470, #17783, #48013, #3899, #22199, #13041, #44647, #40210, #38837, #8625, #35773, #39912, #53801, #26611, #20551 ),
 .UNSPECIFIED., .F., .F.,
 ( 4, 2, 2, 2, 2, 2, 2, 2, 2, 2, 2, 2, 1, 2, 2, 2, 2, 1, 2, 2, 2, 2, 1, 2, 2, 4 ),
 ( 0.000000000000000000, 0.06250000000000033307, 0.09375000000000018041, 0.1093750000000004441, 0.1250000000000006939, 0.1875000000000002498, 0.2499999999999998057, 0.3124999999999993894, 0.3749999999999989453, 0.4374999999999985012, 0.4999999999999981126, 0.5624999999999976685, 0.5937499999999973355, 0.6093749999999968914, 0.6249999999999964473, 0.6874999999999957812, 0.7187499999999953371, 0.7343749999999952260, 0.7421874999999952260, 0.7499999999999951150, 0.8124999999999962252, 0.8437499999999966693, 0.8593749999999966693, 0.8671874999999966693, 0.8749999999999965583, 1.000000000000000000 ),
 .UNSPECIFIED. ) ;
#3848=CARTESIAN_POINT ( 'NONE',  ( -0.8853410819279036170, -83.03830652476008822, 0.8818642663556593986 ) ) ;
#3852=CARTESIAN_POINT ( 'NONE',  ( -1.388458563311000038, -81.85322848715999555, 0.7658850185041000680 ) ) ;
#3853=CARTESIAN_POINT ( 'NONE',  ( -0.7917463127232000630, -80.03634392611000692, -1.236764296276999797 ) ) ;
#3856=EDGE_CURVE ( 'NONE', #55505, #22441, #47773, .T. ) ;
#3858=CARTESIAN_POINT ( 'NONE',  ( 0.6062141276560999437, -82.36581371194999690, -1.551696954864999922 ) ) ;
#3870=AXIS2_PLACEMENT_3D ( 'NONE', #39423, #57710, #3695 ) ;
#3874=CARTESIAN_POINT ( 'NONE',  ( -0.1834469635243000107, -79.61327907013999550, -1.236465612773999911 ) ) ;
#3889=ORIENTED_EDGE ( 'NONE', *, *, #43305, .T. ) ;
#3899=CARTESIAN_POINT ( 'NONE',  ( 0.9450683339454785115, -79.40746036129796437, 0.8222713226707200063 ) ) ;
#3946=CARTESIAN_POINT ( 'NONE',  ( 0.8682910081118865309, -81.91446363364094907, 0.8987380763722911947 ) ) ;
#3947=CARTESIAN_POINT ( 'NONE',  ( 0.07350186345039000368, -79.58564247267000269, -1.355733752427000116 ) ) ;
#3949=CARTESIAN_POINT ( 'NONE',  ( 0.6752050339386822531, -83.08805329458888878, 1.352705552778453502 ) ) ;
#3978=ORIENTED_EDGE ( 'NONE', *, *, #53175, .F. ) ;
#4037=ORIENTED_EDGE ( 'NONE', *, *, #20942, .F. ) ;
#4055=CARTESIAN_POINT ( 'NONE',  ( -1.250000000000000000, -83.49999999999998579, 0.000000000000000000 ) ) ;
#4062=CARTESIAN_POINT ( 'NONE',  ( 1.330394425097165323, -80.05981249656014143, -0.7208325465702845047 ) ) ;
#4063=CARTESIAN_POINT ( 'NONE',  ( -0.9441204537501906024, -78.54342336913121869, 0.8192162103976715626 ) ) ;
#4073=CARTESIAN_POINT ( 'NONE',  ( 1.614964347157999747, -82.04565794024999548, 0.5400991692461000193 ) ) ;
#4075=ORIENTED_EDGE ( 'NONE', *, *, #32990, .T. ) ;
#4077=CARTESIAN_POINT ( 'NONE',  ( -1.092232985442822102, -82.04166666666664298, -0.6295237254636245616 ) ) ;
#4090=ORIENTED_EDGE ( 'NONE', *, *, #42289, .T. ) ;
#4112=CARTESIAN_POINT ( 'NONE',  ( 0.3277382951148000156, -78.62904613799999254, 1.615386606358000243 ) ) ;
#4117=CARTESIAN_POINT ( 'NONE',  ( 1.249621755023126113, -80.34836072372822002, -0.03568039317074558903 ) ) ;
#4131=B_SPLINE_CURVE_WITH_KNOTS ( 'NONE', 3,
 ( #47897, #47029, #25140, #56159, #7429, #6559, #34565, #47615, #11581, #7139, #25432, #56740, #12148, #20434, #43166, #7717, #43447, #24567, #3008, #21004, #20719, #2431, #15420 ),
 .UNSPECIFIED., .F., .F.,
 ( 4, 2, 2, 2, 1, 1, 1, 2, 2, 2, 2, 2, 4 ),
 ( 0.000000000000000000, 0.2499999999999713007, 0.3749999999999568678, 0.4374999999999500955, 0.4687499999999468758, 0.4843749999999452105, 0.4921874999999448219, 0.4960937499999449884, 0.4999999999999451550, 0.6249999999999588107, 0.7499999999999724665, 0.8749999999999862332, 1.000000000000000000 ),
 .UNSPECIFIED. ) ;
#4146=CARTESIAN_POINT ( 'NONE',  ( 1.420454834158999979, -81.72706753059999585, 0.3724989704330000095 ) ) ;
#4147=CARTESIAN_POINT ( 'NONE',  ( 0.9992737233374668904, -78.79819669903726265, -0.7680393074100418938 ) ) ;
#4151=CARTESIAN_POINT ( 'NONE',  ( 1.541440768196999933, -82.55134846604198628, 0.6318380856084999664 ) ) ;
#4158=ORIENTED_EDGE ( 'NONE', *, *, #55225, .T. ) ;
#4165=CARTESIAN_POINT ( 'NONE',  ( -1.324613189995999862, -83.36847537123300356, -0.7038465009425000085 ) ) ;
#4175=CARTESIAN_POINT ( 'NONE',  ( 0.8822134339024870764, -79.91310085715470279, 0.8851451072459763925 ) ) ;
#4178=VECTOR ( 'NONE', #50468, 1000.000000000000000 ) ;
#4181=CARTESIAN_POINT ( 'NONE',  ( -0.1062458101858989590, -81.72988145023380469, 1.508520553443295942 ) ) ;
#4201=CARTESIAN_POINT ( 'NONE',  ( -1.086186157952083509, -79.55861393801417591, 0.6243850812737060663 ) ) ;
#4202=AXIS2_PLACEMENT_3D ( 'NONE', #17965, #9105, #35955 ) ;
#4250=CARTESIAN_POINT ( 'NONE',  ( 0.07675521435781498814, -81.97078358942633258, 1.247900519352959092 ) ) ;
#4251=CARTESIAN_POINT ( 'NONE',  ( 0.1580158025359000018, -78.26021020222999880, 1.541016301036999936 ) ) ;
#4253=CARTESIAN_POINT ( 'NONE',  ( 0.3159905065672543589, -83.10829663276524570, 1.478797643683121166 ) ) ;
#4258=CARTESIAN_POINT ( 'NONE',  ( 0.4912582738047306941, -81.75727386977339961, -1.149340960687430968 ) ) ;
#4264=ORIENTED_EDGE ( 'NONE', *, *, #10969, .T. ) ;
#4287=CARTESIAN_POINT ( 'NONE',  ( -1.240843214692000096, -81.11237249610999811, -0.5344114414419000036 ) ) ;
#4290=CARTESIAN_POINT ( 'NONE',  ( 0.000000000000000000, -86.39999999999999147, 0.000000000000000000 ) ) ;
#4318=B_SPLINE_CURVE_WITH_KNOTS ( 'NONE', 3,
 ( #12250, #1745, #47999, #52696 ),
 .UNSPECIFIED., .F., .F.,
 ( 4, 4 ),
 ( 0.000000000000000000, 1.000000000000000000 ),
 .UNSPECIFIED. ) ;
#4327=COLOUR_RGB ( '', 0.72549020, 0.75294118, 0.79215686) ;
#4329=ORIENTED_EDGE ( 'NONE', *, *, #45187, .T. ) ;
#4359=FACE_OUTER_BOUND ( 'NONE', #8727, .T. ) ;
#4366=CARTESIAN_POINT ( 'NONE',  ( 1.448902839066656512, -81.12261281811970548, 0.4373190867481531185 ) ) ;
#4377=CARTESIAN_POINT ( 'NONE',  ( -0.6718767921597000869, -82.67725009134899494, 1.564735933714000105 ) ) ;
#4381=FACE_OUTER_BOUND ( 'NONE', #53864, .T. ) ;
#4403=ORIENTED_EDGE ( 'NONE', *, *, #1881, .F. ) ;
#4410=CARTESIAN_POINT ( 'NONE',  ( -0.1834469635243000107, -79.21327907014000402, -1.236465612773999911 ) ) ;
#4411=CARTESIAN_POINT ( 'NONE',  ( -1.069737409789999871, -78.83877241711999773, -1.254012819428000247 ) ) ;
#4412=ORIENTED_EDGE ( 'NONE', *, *, #54106, .F. ) ;
#4416=CARTESIAN_POINT ( 'NONE',  ( 0.9762155229984909033, -80.29668698289697204, -0.7812602609263914477 ) ) ;
#4440=CARTESIAN_POINT ( 'NONE',  ( -0.5511181765943999888, -82.99009435914298649, -1.486830790314999984 ) ) ;
#4442=CARTESIAN_POINT ( 'NONE',  ( -0.7285569484545000307, -80.09966061487999411, -1.138057995564000002 ) ) ;
#4446=CARTESIAN_POINT ( 'NONE',  ( -1.552248384014999871, -82.74082611137200161, 0.6048007385293000526 ) ) ;
#4454=ORIENTED_EDGE ( 'NONE', *, *, #25310, .T. ) ;
#4546=CARTESIAN_POINT ( 'NONE',  ( 1.520902128651999918, -80.98694329177000384, -0.6797894616744000196 ) ) ;
#4547=CARTESIAN_POINT ( 'NONE',  ( 1.182381611807000077, -79.15875043768998864, -0.8124367623325000620 ) ) ;
#4549=CARTESIAN_POINT ( 'NONE',  ( 0.6083220426053820296, -82.59209150926855614, 1.384507690863692408 ) ) ;
#4556=CARTESIAN_POINT ( 'NONE',  ( 1.155696476636351555, -81.81899358315281745, -0.4761507332103875889 ) ) ;
#4560=DIRECTION ( 'NONE',  ( -1.000000000000000000, 0.000000000000000000, 0.000000000000000000 ) ) ;
#4561=ORIENTED_EDGE ( 'NONE', *, *, #44622, .F. ) ;
#4563=FACE_OUTER_BOUND ( 'NONE', #9355, .T. ) ;
#4586=CARTESIAN_POINT ( 'NONE',  ( 1.288070761429999989, -80.35446191477998923, 0.4084665662698999666 ) ) ;
#4590=CARTESIAN_POINT ( 'NONE',  ( -0.8333782921101757779, -79.16723044587702418, -0.9320641449025461878 ) ) ;
#4627=ORIENTED_EDGE ( 'NONE', *, *, #21672, .T. ) ;
#4643=B_SPLINE_CURVE_WITH_KNOTS ( 'NONE', 3,
 ( #58141, #35695, #320, #18297, #14432, #18877, #23878, #55178, #19170, #50769 ),
 .UNSPECIFIED., .F., .F.,
 ( 4, 2, 2, 2, 4 ),
 ( 0.5000000007922399403, 0.6250000005941799275, 0.7500000003961200257, 0.8750000001980600128, 1.000000000000000000 ),
 .UNSPECIFIED. ) ;
#4662=CARTESIAN_POINT ( 'NONE',  ( 0.6809358820633165665, -79.67024612424833663, -1.063416950850958331 ) ) ;
#4670=CARTESIAN_POINT ( 'NONE',  ( 1.385745491928287665, -80.63676124254567412, 0.6939760826984652242 ) ) ;
#4671=CARTESIAN_POINT ( 'NONE',  ( -0.9326541099288512271, -78.54231991824191539, 0.8322237885996108808 ) ) ;
#4713=CARTESIAN_POINT ( 'NONE',  ( 0.3051819181680999749, -78.56572944923000534, 1.504208664230000103 ) ) ;
#4716=CARTESIAN_POINT ( 'NONE',  ( 0.08493805541549671878, -80.23085499046800351, -1.247011083204105919 ) ) ;
#4731=FACE_OUTER_BOUND ( 'NONE', #55790, .T. ) ;
#4738=CARTESIAN_POINT ( 'NONE',  ( -0.7208041749482999583, -83.30589043469399257, 1.412512638229999951 ) ) ;
#4739=CARTESIAN_POINT ( 'NONE',  ( 0.3269278782881216983, -78.74609622332656045, -1.249941949099096172 ) ) ;
#4741=CARTESIAN_POINT ( 'NONE',  ( -1.250000000000000000, -79.00000000000000000, 0.000000000000000000 ) ) ;
#4743=CARTESIAN_POINT ( 'NONE',  ( 0.000000000000000000, -87.20000000000000284, -10.05000000000000071 ) ) ;
#4749=FACE_OUTER_BOUND ( 'NONE', #15583, .T. ) ;
#4764=CARTESIAN_POINT ( 'NONE',  ( -1.156132896548696776, -81.56914977956330404, 0.4749676188561988144 ) ) ;
#4768=CARTESIAN_POINT ( 'NONE',  ( 1.077757070171020848, -81.53756520157187992, -1.059880615153325989 ) ) ;
#4778=ORIENTED_EDGE ( 'NONE', *, *, #43702, .T. ) ;
#4779=DIRECTION ( 'NONE',  ( 0.000000000000000000, 1.000000000000000000, 0.000000000000000000 ) ) ;
#4789=ORIENTED_EDGE ( 'NONE', *, *, #26674, .T. ) ;
#4800=CARTESIAN_POINT ( 'NONE',  ( 0.1429208184976999974, -78.63839451269998904, 1.621183732314999792 ) ) ;
#4841=CARTESIAN_POINT ( 'NONE',  ( 0.3704480504712000521, -79.85402031102998421, -1.624200486671999899 ) ) ;
#4842=CARTESIAN_POINT ( 'NONE',  ( -0.6865653500940999132, -77.98180235332999644, -1.388644167491000170 ) ) ;
#4844=CARTESIAN_POINT ( 'NONE',  ( 1.475387890451711925, -83.01720161097178163, 0.3238678118364496927 ) ) ;
#4851=B_SPLINE_CURVE_WITH_KNOTS ( 'NONE', 3,
 ( #4741, #22740, #345, #36316, #55495, #33037, #10632, #1491, #19481, #41335, #33336, #24200, #19777, #37474, #23900, #15045, #28315, #46953 ),
 .UNSPECIFIED., .F., .F.,
 ( 4, 2, 2, 2, 2, 2, 2, 2, 4 ),
 ( 0.000000000000000000, 0.1249999999999999722, 0.2500000000000000000, 0.3750000000000000000, 0.5000000000000001110, 0.6250000000000001110, 0.7500000000000000000, 0.8750000000000000000, 1.000000000000000000 ),
 .UNSPECIFIED. ) ;
#4857=ORIENTED_EDGE ( 'NONE', *, *, #33179, .T. ) ;
#4862=CARTESIAN_POINT ( 'NONE',  ( 1.151665787602303759, -80.38188276058083659, 0.4857789717937905372 ) ) ;
#4873=LINE ( 'NONE', #18451, #19696 ) ;
#4880=CARTESIAN_POINT ( 'NONE',  ( -1.348464306027999937, -81.17568918487999952, -0.5807621341562000383 ) ) ;
#4895=DIRECTION ( 'NONE',  ( 0.000000000000000000, -1.000000000000000000, 0.000000000000000000 ) ) ;
#4904=ORIENTED_EDGE ( 'NONE', *, *, #32931, .T. ) ;
#4954=B_SPLINE_CURVE_WITH_KNOTS ( 'NONE', 3,
 ( #46086, #56096, #11227, #24501 ),
 .UNSPECIFIED., .F., .F.,
 ( 4, 4 ),
 ( 0.000000000000000000, 1.000000000000000000 ),
 .UNSPECIFIED. ) ;
#4992=CARTESIAN_POINT ( 'NONE',  ( -1.207620444084886113, -80.57949090611919019, 0.3245627370427532354 ) ) ;
#4999=CARTESIAN_POINT ( 'NONE',  ( -1.312001604499999807, -77.67439276297999129, 0.5631709907292000716 ) ) ;
#5001=EDGE_CURVE ( 'NONE', #50285, #32332, #39206, .T. ) ;
#5004=CARTESIAN_POINT ( 'NONE',  ( 1.154865739624113985, -80.31888759917194420, -0.4781106390998191014 ) ) ;
#5017=DIRECTION ( 'NONE',  ( -1.000000000000000000, 0.000000000000000000, 0.000000000000000000 ) ) ;
#5026=CARTESIAN_POINT ( 'NONE',  ( 1.392666586335999934, -82.23234125147999407, 0.4657552147452999614 ) ) ;
#5041=B_SPLINE_CURVE_WITH_KNOTS ( 'NONE', 3,
 ( #14025, #14895, #9610, #32307, #46519, #32893, #10195, #27597, #45932, #10485, #5178, #54194, #5465, #45639, #23184, #13732, #23468, #1064 ),
 .UNSPECIFIED., .F., .F.,
 ( 4, 2, 2, 2, 2, 2, 2, 2, 4 ),
 ( 0.000000000000000000, 0.1250000000000000833, 0.2500000000000001110, 0.3750000000000000000, 0.4999999999999999445, 0.6249999999999998890, 0.7499999999999997780, 0.8749999999999998890, 1.000000000000000000 ),
 .UNSPECIFIED. ) ;
#5092=CARTESIAN_POINT ( 'NONE',  ( -1.481905647302000029, -78.24508877014999086, -0.6727694308694001091 ) ) ;
#5132=CARTESIAN_POINT ( 'NONE',  ( 0.5818457612699999837, -80.92378407665999873, -1.560998038830999857 ) ) ;
#5133=CARTESIAN_POINT ( 'NONE',  ( -1.275974813924000140, -78.99934084733999384, 0.3384762398118000282 ) ) ;
#5135=CARTESIAN_POINT ( 'NONE',  ( 0.1237032920003742348, -83.11841830185345259, 1.505458275059794460 ) ) ;
#5140=CARTESIAN_POINT ( 'NONE',  ( 1.184538586134731508, -81.82436935641939613, -0.3988734786993729520 ) ) ;
#5146=DIRECTION ( 'NONE',  ( 0.000000000000000000, 0.000000000000000000, -1.000000000000000000 ) ) ;
#5167=CARTESIAN_POINT ( 'NONE',  ( 0.5128916439544000117, -80.79673389420999285, -1.376005298375999830 ) ) ;
#5178=CARTESIAN_POINT ( 'NONE',  ( -0.3271848554490991434, -79.10416666666665719, -1.217465845835395299 ) ) ;
#5192=VECTOR ( 'NONE', #25207, 1000.000000000000000 ) ;
#5220=ORIENTED_EDGE ( 'NONE', *, *, #39281, .F. ) ;
#5221=CARTESIAN_POINT ( 'NONE',  ( 0.8840402821807384903, -82.78818478153729643, -0.8831652403929096673 ) ) ;
#5222=ORIENTED_EDGE ( 'NONE', *, *, #6014, .T. ) ;
#5231=CARTESIAN_POINT ( 'NONE',  ( 0.000000000000000000, -77.50000000000000000, 0.000000000000000000 ) ) ;
#5243=CARTESIAN_POINT ( 'NONE',  ( -9.500000000000000000, -91.89999999999999147, 0.000000000000000000 ) ) ;
#5246=CARTESIAN_POINT ( 'NONE',  ( 1.250000000000000000, -80.74999999999998579, 0.000000000000000000 ) ) ;
#5249=CARTESIAN_POINT ( 'NONE',  ( 0.5327588397318764324, -79.50310756622292274, -1.415177852321873209 ) ) ;
#5256=CARTESIAN_POINT ( 'NONE',  ( -1.623947472758999977, -83.24568302734098779, 0.5113958356693000251 ) ) ;
#5282=CARTESIAN_POINT ( 'NONE',  ( -1.189861610678828008, -80.57546913605862926, 0.3832792502281296421 ) ) ;
#5287=LINE ( 'NONE', #23295, #4178 ) ;
#5288=CARTESIAN_POINT ( 'NONE',  ( -0.6796159160043999670, -78.61816101900998888, 1.376191089724000172 ) ) ;
#5306=ADVANCED_FACE ( 'NONE', ( #14288 ), #10280, .T. ) ;
#5307=DIRECTION ( 'NONE',  ( 0.000000000000000000, -1.000000000000000000, 0.000000000000000000 ) ) ;
#5310=CIRCLE ( 'NONE', #27966, 2.299999999999999822 ) ;
#5317=CARTESIAN_POINT ( 'NONE',  ( -0.5331523304941999664, -82.92725009134899494, 1.241660107034999960 ) ) ;
#5318=CARTESIAN_POINT ( 'NONE',  ( -1.091933803201964315, -78.64189527190625029, -0.6291797731469532806 ) ) ;
#5320=CARTESIAN_POINT ( 'NONE',  ( 1.092232985442820992, -82.79166666666665719, 0.6295237254636267821 ) ) ;
#5322=CARTESIAN_POINT ( 'NONE',  ( -1.519662023741000123, -82.80398532648199250, -0.6825586799200999977 ) ) ;
#5342=CARTESIAN_POINT ( 'NONE',  ( -0.5388325380043634816, -81.51077761135140065, 1.127735728752304656 ) ) ;
#5348=CARTESIAN_POINT ( 'NONE',  ( -9.000000000000000000, -91.89999999999999147, -2.445120494964999949E-12 ) ) ;
#5349=AXIS2_PLACEMENT_3D ( 'NONE', #5818, #32664, #50717 ) ;
#5354=ORIENTED_EDGE ( 'NONE', *, *, #9210, .T. ) ;
#5362=DIRECTION ( 'NONE',  ( 0.000000000000000000, 1.000000000000000000, 0.000000000000000000 ) ) ;
#5369=ORIENTED_EDGE ( 'NONE', *, *, #6783, .T. ) ;
#5376=CARTESIAN_POINT ( 'NONE',  ( 0.4102083068199999794, -78.35645190970998897, -1.574926093281000083 ) ) ;
#5399=FACE_OUTER_BOUND ( 'NONE', #18724, .T. ) ;
#5412=CARTESIAN_POINT ( 'NONE',  ( 1.551146335801999898, -80.99088618300999087, 0.6076261867840000441 ) ) ;
#5413=CARTESIAN_POINT ( 'NONE',  ( -0.7268831363637999754, -77.94139102152999499, 1.101817922911999981 ) ) ;
#5415=CARTESIAN_POINT ( 'NONE',  ( -1.549803789708370738, -82.27831976753381582, -0.5760661418227226438 ) ) ;
#5421=CARTESIAN_POINT ( 'NONE',  ( -1.249786646214342989, -81.60930685382331262, -0.1405899892054735811 ) ) ;
#5428=DIRECTION ( 'NONE',  ( 0.000000000000000000, -1.000000000000000000, 0.000000000000000000 ) ) ;
#5436=DIRECTION ( 'NONE',  ( 0.000000000000000000, -1.000000000000000000, 0.000000000000000000 ) ) ;
#5443=CARTESIAN_POINT ( 'NONE',  ( -0.1636246173744726473, -81.38541666666664298, 1.249999999999999112 ) ) ;
#5444=VECTOR ( 'NONE', #10860, 1000.000000000000000 ) ;
#5452=CARTESIAN_POINT ( 'NONE',  ( -0.2789364955927000067, -79.53354959200999019, 1.441751320050999929 ) ) ;
#5465=CARTESIAN_POINT ( 'NONE',  ( -0.7681833999686432657, -79.07291666666668561, -0.9995835529977258327 ) ) ;
#5485=EDGE_CURVE ( 'NONE', #7824, #41164, #27858, .T. ) ;
#5513=EDGE_CURVE ( 'NONE', #40202, #31102, #11338, .T. ) ;
#5518=FACE_OUTER_BOUND ( 'NONE', #22852, .T. ) ;
#5523=CARTESIAN_POINT ( 'NONE',  ( -1.156432516341094896, -83.06912217221712069, 0.4743574928646153710 ) ) ;
#5528=CARTESIAN_POINT ( 'NONE',  ( 1.510215997576003222, -79.60432664446625495, 0.09564393186081109055 ) ) ;
#5566=CARTESIAN_POINT ( 'NONE',  ( -1.242201279478839959, -80.59188204877600015, 0.1373445331278350945 ) ) ;
#5575=CARTESIAN_POINT ( 'NONE',  ( -0.7905733931407377124, -80.17088946056077248, -0.9685879666675529798 ) ) ;
#5579=CARTESIAN_POINT ( 'NONE',  ( 1.343421608112092658, -78.06192807433161818, -0.6881263894564929595 ) ) ;
#5594=CARTESIAN_POINT ( 'NONE',  ( 0.4072933538588000002, -82.16933951002999947, -1.288442219433000080 ) ) ;
#5620=VERTEX_POINT ( 'NONE', #48717 ) ;
#5630=CARTESIAN_POINT ( 'NONE',  ( -1.266141431829999942, -77.60019095522000043, -0.3277948212408000050 ) ) ;
#5660=CARTESIAN_POINT ( 'NONE',  ( -1.560595261880000084, -77.68827307234998614, 0.4619550309703999713 ) ) ;
#5699=CARTESIAN_POINT ( 'NONE',  ( -1.529754383668999962, -81.24352304346000153, -0.6588408878327000062 ) ) ;
#5700=CARTESIAN_POINT ( 'NONE',  ( -0.5850755440913000260, -78.10843573086999925, -1.183371315974999893 ) ) ;
#5702=CARTESIAN_POINT ( 'NONE',  ( 1.518408311387865917, -81.48882957865839671, -0.2150362242269064084 ) ) ;
#5703=CARTESIAN_POINT ( 'NONE',  ( 0.1237567301189053115, -83.21780190041201308, 1.506540253472085755 ) ) ;
#5706=CARTESIAN_POINT ( 'NONE',  ( -1.218468010184407202, -81.07986474255089604, 0.3279021448883003842 ) ) ;
#5739=CARTESIAN_POINT ( 'NONE',  ( 0.7658660592953000501, -79.40707368812999789, 1.113292320107999833 ) ) ;
#5777=CONICAL_SURFACE ( 'NONE', #38770, 10.09999999997999964, 0.7853981633972997312 ) ;
#5784=DIRECTION ( 'NONE',  ( 0.000000000000000000, 1.000000000000000000, 0.000000000000000000 ) ) ;
#5809=CYLINDRICAL_SURFACE ( 'NONE', #31753, 1.250000000000000000 ) ;
#5816=CARTESIAN_POINT ( 'NONE',  ( 1.115776411654021860, -82.88725312741937046, 0.5639269211292178285 ) ) ;
#5818=CARTESIAN_POINT ( 'NONE',  ( 0.000000000000000000, -87.09999999999999432, 0.000000000000000000 ) ) ;
#5841=CARTESIAN_POINT ( 'NONE',  ( 0.7311670807272000472, -82.22766660800999716, 1.496881327486000002 ) ) ;
#5844=EDGE_LOOP ( 'NONE', ( #47249, #20049, #54096, #24145 ) ) ;
#5856=AXIS2_PLACEMENT_3D ( 'NONE', #50630, #41171, #9887 ) ;
#5873=CARTESIAN_POINT ( 'NONE',  ( 1.210448961617198282, -79.15058965391948220, 0.9017437205617973017 ) ) ;
#5878=CARTESIAN_POINT ( 'NONE',  ( 0.000000000000000000, -76.75499999999999545, 0.000000000000000000 ) ) ;
#5906=CARTESIAN_POINT ( 'NONE',  ( -0.3070260000256299082, -79.20550685558696102, -1.218020810600508153 ) ) ;
#5919=CARTESIAN_POINT ( 'NONE',  ( -0.8842298993840882471, -81.53809034327093741, 0.8830699700463247037 ) ) ;
#5952=CARTESIAN_POINT ( 'NONE',  ( 2.500000000000000000, -80.69999999999998863, 0.000000000000000000 ) ) ;
#5954=CARTESIAN_POINT ( 'NONE',  ( -0.1732310466989999687, -77.59547045605000903, 1.530487294790999986 ) ) ;
#5957=( GEOMETRIC_REPRESENTATION_CONTEXT ( 3 ) GLOBAL_UNCERTAINTY_ASSIGNED_CONTEXT ( ( #37827 ) ) GLOBAL_UNIT_ASSIGNED_CONTEXT ( ( #56019, #10567, #24720 ) ) REPRESENTATION_CONTEXT ( 'NONE', 'WORKASPACE' ) );
#5964=CARTESIAN_POINT ( 'NONE',  ( -1.494795747725999879, -80.92041546398999685, -0.5291335979940999801 ) ) ;
#5992=CARTESIAN_POINT ( 'NONE',  ( -1.542698325316999908, -81.29879647607999971, 0.6290719308543000210 ) ) ;
#5993=CARTESIAN_POINT ( 'NONE',  ( 1.031014977102000074, -78.26784532121999405, 0.9975409193212999570 ) ) ;
#5996=CARTESIAN_POINT ( 'NONE',  ( -1.500000000000000000, -83.34999999999999432, 0.000000000000000000 ) ) ;
#5997=EDGE_LOOP ( 'NONE', ( #1864, #4904, #21685, #10220, #28201, #44556, #40343, #37595, #14059, #25029, #29160 ) ) ;
#5998=CARTESIAN_POINT ( 'NONE',  ( 1.249651984936067439, -79.84628556922963583, -0.06748478051193507188 ) ) ;
#6003=CARTESIAN_POINT ( 'NONE',  ( 0.3134647746052411921, -81.74538725804720229, -1.211105577459558269 ) ) ;
#6014=EDGE_CURVE ( 'NONE', #16529, #515, #54870, .T. ) ;
#6018=CARTESIAN_POINT ( 'NONE',  ( 0.000000000000000000, -86.29999999996098836, 0.000000000000000000 ) ) ;
#6030=CARTESIAN_POINT ( 'NONE',  ( -0.3737996561424999920, -80.03882331289000263, 1.420113360969999849 ) ) ;
#6034=CARTESIAN_POINT ( 'NONE',  ( 0.1623090455760520801, -79.38352240831720508, -1.503739187786481191 ) ) ;
#6043=CARTESIAN_POINT ( 'NONE',  ( -1.135826688880000157, -81.30663953507000485, -0.9797437077257000748 ) ) ;
#6075=CARTESIAN_POINT ( 'NONE',  ( 1.249471583050132839, -78.32919795546139596, -0.3269302217491961149 ) ) ;
#6086=CARTESIAN_POINT ( 'NONE',  ( 1.186068794074434996, -82.82441975421146196, -0.3952336422712977027 ) ) ;
#6090=CARTESIAN_POINT ( 'NONE',  ( -1.521427883520144686, -78.25414970944238746, -0.07951690128473563879 ) ) ;
#6110=CARTESIAN_POINT ( 'NONE',  ( 0.8734639515568026757, -82.91404585606140643, 0.8936271339499843869 ) ) ;
#6119=CARTESIAN_POINT ( 'NONE',  ( -1.493074398910679834, -79.83713052442533353, 0.2323495900538211922 ) ) ;
#6135=CARTESIAN_POINT ( 'NONE',  ( -0.5790013745696001024, -82.98557718933099636, -1.562055304842999925 ) ) ;
#6147=CARTESIAN_POINT ( 'NONE',  ( 0.6294848425788325263, -80.76745373571634445, -1.093351163505755341 ) ) ;
#6148=ORIENTED_EDGE ( 'NONE', *, *, #38393, .F. ) ;
#6155=CARTESIAN_POINT ( 'NONE',  ( -1.055666910258088231, -80.55513841626326155, 0.6698640694703560383 ) ) ;
#6159=EDGE_LOOP ( 'NONE', ( #19027, #42909, #14269, #13943, #41729, #1093, #49408, #56851, #13957, #46261, #3889, #27054 ) ) ;
#6165=CARTESIAN_POINT ( 'NONE',  ( -0.3490198212478526907, -80.20286839885675079, -1.200175596027631908 ) ) ;
#6170=CARTESIAN_POINT ( 'NONE',  ( 0.5445062389433608097, -78.69549341983497470, 1.437445382695913487 ) ) ;
#6184=CARTESIAN_POINT ( 'NONE',  ( -1.357301787716079788, -81.28639619689411688, -0.6673137404722703225 ) ) ;
#6187=CARTESIAN_POINT ( 'NONE',  ( 0.000000000000000000, -77.69999999999998863, 0.000000000000000000 ) ) ;
#6193=CARTESIAN_POINT ( 'NONE',  ( -0.5331523304941999664, -82.48730002504399295, 1.241660107034999960 ) ) ;
#6210=CARTESIAN_POINT ( 'NONE',  ( 0.9272193457273129047, -81.40918307165384249, 0.8400180975224862401 ) ) ;
#6215=CARTESIAN_POINT ( 'NONE',  ( -1.140778876102999995, -79.12070647882998742, -0.6399209788899999918 ) ) ;
#6243=CARTESIAN_POINT ( 'NONE',  ( 0.4326115402657000342, -78.97601868546000503, -1.568920109259999807 ) ) ;
#6244=CARTESIAN_POINT ( 'NONE',  ( -0.9428654619097610601, -79.15721871088541661, -0.8204702594945776362 ) ) ;
#6278=CARTESIAN_POINT ( 'NONE',  ( -0.6492849177312852715, -80.01898409060812867, 1.068617496498147856 ) ) ;
#6286=CARTESIAN_POINT ( 'NONE',  ( 0.2617232932829000047, -79.40796291402000406, -1.644907507304999905 ) ) ;
#6287=CARTESIAN_POINT ( 'NONE',  ( -0.7581747471680000405, -78.94365927756000190, 1.080670598843999963 ) ) ;
#6289=CARTESIAN_POINT ( 'NONE',  ( 1.205168758126570427, -81.44834290230591023, -0.9133787470919593199 ) ) ;
#6295=CARTESIAN_POINT ( 'NONE',  ( 0.9994933351473022087, -80.90274815551298104, 0.7676091254557989574 ) ) ;
#6296=ORIENTED_EDGE ( 'NONE', *, *, #38342, .T. ) ;
#6298=CARTESIAN_POINT ( 'NONE',  ( 0.1446683541241534920, -81.73463977978825312, -1.242005837416781056 ) ) ;
#6317=CARTESIAN_POINT ( 'NONE',  ( 1.217465845835393967, -81.27083333333332860, 0.3271848554491025851 ) ) ;
#6322=CARTESIAN_POINT ( 'NONE',  ( -0.6295237254636286695, -79.91666666666665719, 1.092232985442819881 ) ) ;
#6325=CARTESIAN_POINT ( 'NONE',  ( -1.321122997307999869, -79.66002549588999671, 0.8769429413327000100 ) ) ;
#6344=CARTESIAN_POINT ( 'NONE',  ( -0.004472651058881748666, -78.47550862917535142, 1.249857563130390981 ) ) ;
#6380=ORIENTED_EDGE ( 'NONE', *, *, #48957, .F. ) ;
#6385=CARTESIAN_POINT ( 'NONE',  ( 0.9916361112363957231, -78.06929481599125609, 1.169919221591249503 ) ) ;
#6402=CARTESIAN_POINT ( 'NONE',  ( 0.9188661267636154539, -82.90988150905879195, 0.8478900103341754368 ) ) ;
#6404=DIRECTION ( 'NONE',  ( 0.000000000000000000, -1.000000000000000000, 0.000000000000000000 ) ) ;
#6405=CARTESIAN_POINT ( 'NONE',  ( 0.6295237254636211199, -80.33333333333334281, 1.092232985442824322 ) ) ;
#6416=SURFACE_STYLE_FILL_AREA ( #10867 ) ;
#6423=DIRECTION ( 'NONE',  ( 0.000000000000000000, -1.000000000000000000, 0.000000000000000000 ) ) ;
#6427=CARTESIAN_POINT ( 'NONE',  ( 0.7076411874954000591, -83.04873640444098726, -1.508144869335000138 ) ) ;
#6435=ADVANCED_FACE ( 'NONE', ( #25413 ), #48164, .F. ) ;
#6444=CARTESIAN_POINT ( 'NONE',  ( -0.6282371225189693487, -80.51721610571219401, 1.080583994657213998 ) ) ;
#6461=CARTESIAN_POINT ( 'NONE',  ( 0.7804427332109117321, -79.01673782036979787, -1.323298261115681385 ) ) ;
#6476=CARTESIAN_POINT ( 'NONE',  ( 0.5739952604901000788, -83.17988695178998171, -1.223314898041000021 ) ) ;
#6479=DIRECTION ( 'NONE',  ( 0.000000000000000000, 1.000000000000000000, 0.000000000000000000 ) ) ;
#6489=CARTESIAN_POINT ( 'NONE',  ( 1.250000000000000222, -82.23958333333330017, -0.1636246173744659582 ) ) ;
#6505=EDGE_CURVE ( 'NONE', #45641, #50158, #44530, .T. ) ;
#6506=CARTESIAN_POINT ( 'NONE',  ( 1.250000000000000000, -81.34999999999999432, 0.000000000000000000 ) ) ;
#6507=EDGE_CURVE ( 'NONE', #31243, #50285, #34448, .T. ) ;
#6509=CARTESIAN_POINT ( 'NONE',  ( 0.6295189948058200757, -82.26732208686871672, -1.093239786954644410 ) ) ;
#6525=CARTESIAN_POINT ( 'NONE',  ( 0.000000000000000000, -91.89999999999999147, 0.000000000000000000 ) ) ;
#6541=CARTESIAN_POINT ( 'NONE',  ( 0.4102083068199999794, -78.53410088132000055, -1.574926093281000083 ) ) ;
#6550=CARTESIAN_POINT ( 'NONE',  ( 0.9651418585498000580, -79.65707368812999789, 1.402967275931999769 ) ) ;
#6559=CARTESIAN_POINT ( 'NONE',  ( 0.7369231997792153877, -81.27577443587277628, -1.011343237770755632 ) ) ;
#6583=CARTESIAN_POINT ( 'NONE',  ( -1.192863218486718724, -81.80260132039094856, -0.9258880463762395596 ) ) ;
#6585=CARTESIAN_POINT ( 'NONE',  ( -0.02827822798232390578, -81.97280723801726765, -1.511008595699627532 ) ) ;
#6586=CARTESIAN_POINT ( 'NONE',  ( -0.8768947901867296668, -79.66348982473350304, -0.8905431139892215908 ) ) ;
#6590=CARTESIAN_POINT ( 'NONE',  ( -1.151942055393958553, -81.63187234693144489, -0.4850639606811199545 ) ) ;
#6617=CARTESIAN_POINT ( 'NONE',  ( 0.4877854313978999268, -80.41809355086999744, -1.631527605715999973 ) ) ;
#6628=CARTESIAN_POINT ( 'NONE',  ( -1.250000000000000000, -80.99999999999998579, 0.000000000000000000 ) ) ;
#6639=CARTESIAN_POINT ( 'NONE',  ( 0.3401359493934584810, -78.45311654837766469, 1.203085218402039525 ) ) ;
#6648=CARTESIAN_POINT ( 'NONE',  ( -1.249549403371825740, -82.09031365513524747, 0.1639824843638148233 ) ) ;
#6680=CARTESIAN_POINT ( 'NONE',  ( -1.499313493251033913, -78.74149442853628500, 0.1614851097358912524 ) ) ;
#6688=CARTESIAN_POINT ( 'NONE',  ( 0.3918244861196526485, -81.20358808071422629, 1.461319962763056868 ) ) ;
#6699=CARTESIAN_POINT ( 'NONE',  ( 0.8515782275871298657, -82.91596154203972446, 0.9145198330317436675 ) ) ;
#6701=CARTESIAN_POINT ( 'NONE',  ( -1.217465845835396188, -80.47916666666668561, 0.3271848554490955907 ) ) ;
#6726=ORIENTED_EDGE ( 'NONE', *, *, #50366, .T. ) ;
#6739=CARTESIAN_POINT ( 'NONE',  ( 0.6898300185143996233, -80.42861775785651446, 1.042310243182293483 ) ) ;
#6745=EDGE_LOOP ( 'NONE', ( #49802, #49662, #36189, #42813, #40102 ) ) ;
#6766=CARTESIAN_POINT ( 'NONE',  ( 0.1636246173744697330, -78.63541666666665719, -1.249999999999999778 ) ) ;
#6769=CARTESIAN_POINT ( 'NONE',  ( 1.497208609717835648, -80.01106589178321826, 0.2087373732156078132 ) ) ;
#6779=CARTESIAN_POINT ( 'NONE',  ( 1.250322495222000008, -82.36098159482000369, 0.5125084194436000384 ) ) ;
#6783=EDGE_CURVE ( 'NONE', #24608, #29213, #47398, .T. ) ;
#6798=CARTESIAN_POINT ( 'NONE',  ( -0.2725461282999930845, -81.49265652800838211, 1.220870497201928639 ) ) ;
#6800=CARTESIAN_POINT ( 'NONE',  ( -1.250000000000000000, -80.99999999999998579, 0.000000000000000000 ) ) ;
#6803=CARTESIAN_POINT ( 'NONE',  ( -1.118058248199999882, -77.54775938543998848, 0.4799216473306999742 ) ) ;
#6829=CARTESIAN_POINT ( 'NONE',  ( -1.491326706514000122, -77.92160361373998967, -0.6515838025032999470 ) ) ;
#6838=CARTESIAN_POINT ( 'NONE',  ( 1.529418508686999800, -83.11625531570498993, 0.7487957062819000642 ) ) ;
#6839=CARTESIAN_POINT ( 'NONE',  ( -0.6027184710183000060, -81.29937075464998486, 1.466649853462000053 ) ) ;
#6867=CARTESIAN_POINT ( 'NONE',  ( -0.8943305861287761394, -80.03894847689588232, 0.8728967361965981331 ) ) ;
#6870=CARTESIAN_POINT ( 'NONE',  ( 0.000000000000000000, -77.69999999999998863, -2.500000000003963496 ) ) ;
#6872=CARTESIAN_POINT ( 'NONE',  ( 1.250000000000000000, -78.85000000000000853, 0.000000000000000000 ) ) ;
#6874=CARTESIAN_POINT ( 'NONE',  ( 0.8231928634769288822, -82.51939026053260307, -1.312852273108907397 ) ) ;
#6875=CARTESIAN_POINT ( 'NONE',  ( -1.211605918170402196, -79.62183856433064477, -0.3412175572405004020 ) ) ;
#6907=CARTESIAN_POINT ( 'NONE',  ( 1.505228744355000092, -80.48125276597998834, -0.7963060858757999849 ) ) ;
#6927=CARTESIAN_POINT ( 'NONE',  ( 0.3711240750354344864, -78.45108290871590384, 1.193600970463786881 ) ) ;
#6935=FACE_OUTER_BOUND ( 'NONE', #35276, .T. ) ;
#6936=VECTOR ( 'NONE', #15509, 1000.000000000000000 ) ;
#6950=CARTESIAN_POINT ( 'NONE',  ( -1.250013176831791695, -78.10006463709670754, 4.053087819277079897E-06 ) ) ;
#6951=DIRECTION ( 'NONE',  ( 0.000000000000000000, 0.000000000000000000, -1.000000000000000000 ) ) ;
#6956=EDGE_CURVE ( 'NONE', #22441, #17800, #49325, .T. ) ;
#6968=CARTESIAN_POINT ( 'NONE',  ( 1.520089283902537947, -78.48941957383496515, -0.1979304151590696170 ) ) ;
#6986=CARTESIAN_POINT ( 'NONE',  ( 0.6995068289773208603, -82.92824216472010335, 1.038481775461846057 ) ) ;
#6988=CARTESIAN_POINT ( 'NONE',  ( 0.1636246173744642929, -80.36458333333335702, 1.250000000000000888 ) ) ;
#6996=EDGE_CURVE ( 'NONE', #12208, #22441, #26713, .T. ) ;
#7021=CARTESIAN_POINT ( 'NONE',  ( -0.9211504236885831309, -80.66021725436883116, -0.8591334638782682775 ) ) ;
#7029=CARTESIAN_POINT ( 'NONE',  ( -0.2496591548053319620, -80.49116606994940071, 1.224717197152575654 ) ) ;
#7048=CARTESIAN_POINT ( 'NONE',  ( -0.7748888817652298533, -77.76745404050591048, 1.296322661737231874 ) ) ;
#7060=CARTESIAN_POINT ( 'NONE',  ( 0.5006249160878237792, -80.90177277154016622, -1.427178972532155088 ) ) ;
#7069=CARTESIAN_POINT ( 'NONE',  ( 1.495758047513000122, -82.92972947813200335, -0.5264119980271999566 ) ) ;
#7077=VECTOR ( 'NONE', #32887, 1000.000000000000000 ) ;
#7089=CARTESIAN_POINT ( 'NONE',  ( 0.3808713525295242541, -81.45074787893075552, 1.190513909683055926 ) ) ;
#7090=EDGE_CURVE ( 'NONE', #42991, #2755, #15447, .T. ) ;
#7095=CARTESIAN_POINT ( 'NONE',  ( 0.1636246173744642929, -78.36458333333330017, 1.250000000000000888 ) ) ;
#7116=VERTEX_POINT ( 'NONE', #10254 ) ;
#7124=CARTESIAN_POINT ( 'NONE',  ( -1.472167250137000005, -78.86465554589999272, -0.6938203229310999642 ) ) ;
#7131=CARTESIAN_POINT ( 'NONE',  ( 0.8322913257134999521, -79.78370706566998649, 1.209850638715999960 ) ) ;
#7139=CARTESIAN_POINT ( 'NONE',  ( 0.4919046592935741868, -81.25746093831025973, -1.149158243204877472 ) ) ;
#7164=CARTESIAN_POINT ( 'NONE',  ( -1.506971685459099097, -82.84329131091146792, 0.1165168607353958691 ) ) ;
#7165=CARTESIAN_POINT ( 'NONE',  ( -0.2710612067321039320, -79.70821832930488426, -1.220449725728272705 ) ) ;
#7198=CARTESIAN_POINT ( 'NONE',  ( -0.1636246173744673738, -81.11458333333331439, -1.249999999999999778 ) ) ;
#7212=VERTEX_POINT ( 'NONE', #47742 ) ;
#7216=CARTESIAN_POINT ( 'NONE',  ( 1.228871970593624852, -78.36477678297961802, 0.2288398227139316898 ) ) ;
#7230=CARTESIAN_POINT ( 'NONE',  ( -1.607979213109999916, -78.80939078103999407, 0.4265466307092000142 ) ) ;
#7260=CARTESIAN_POINT ( 'NONE',  ( -1.215794352730352079, -78.80031189463259977, -0.8913456688967522634 ) ) ;
#7261=CIRCLE ( 'NONE', #42119, 2.500000000000000000 ) ;
#7291=ORIENTED_EDGE ( 'NONE', *, *, #48227, .F. ) ;
#7306=B_SPLINE_CURVE_WITH_KNOTS ( 'NONE', 3,
 ( #45237, #26607, #44644, #54386, #13923, #53798, #31918, #13332, #57922, #31326, #8919, #26041, #22494, #32494, #24247, #10681, #49963 ),
 .UNSPECIFIED., .F., .F.,
 ( 4, 2, 2, 2, 2, 2, 1, 2, 4 ),
 ( 0.000000000000000000, 0.1250000000000000555, 0.2500000000000001110, 0.3750000000000001665, 0.5000000000000002220, 0.6250000000000002220, 0.7500000000000003331, 0.8750000000000001110, 1.000000000000000000 ),
 .UNSPECIFIED. ) ;
#7314=CARTESIAN_POINT ( 'NONE',  ( 0.4619589256644854869, -80.44498959896617407, 1.161429065943083039 ) ) ;
#7328=CYLINDRICAL_SURFACE ( 'NONE', #47812, 9.500000000000000000 ) ;
#7342=CARTESIAN_POINT ( 'NONE',  ( 0.9995835529977264988, -78.69791666666664298, -0.7681833999686417114 ) ) ;
#7343=B_SPLINE_CURVE_WITH_KNOTS ( 'NONE', 3,
 ( #46269, #41523, #32640, #18512, #50692, #37670, #32067, #19385, #1107, #9361, #23799, #41815, #6086, #1390, #46562, #54532, #37376, #45389, #55689, #55391, #24095, #14937, #36506, #14069, #50978, #28512, #50107, #49815, #45681, #5221, #23226, #41230, #820, #25543, #42987, #2544, #37959, #42408, #47433, #20259, #42695, #11695, #11406, #19973, #2259, #20827, #43561, #3127, #11980, #46851, #56273, #55983, #39124, #15533, #51564, #51274, #48009, #52137, #52423, #21117, #24967, #15235, #29385, #33228, #20547, #24394, #38251, #1978, #43276, #10828, #15824, #7544, #34391, #29671 ),
 .UNSPECIFIED., .F., .F.,
 ( 4, 2, 2, 1, 2, 2, 2, 2, 1, 1, 1, 2, 2, 2, 2, 2, 1, 1, 2, 2, 2, 2, 2, 2, 2, 2, 1, 2, 2, 2, 2, 1, 2, 2, 2, 2, 2, 2, 2, 2, 4 ),
 ( 0.000000000000000000, 0.03125000000000469763, 0.04687500000000669603, 0.05468750000000768829, 0.05859375000000816708, 0.06250000000000864586, 0.09375000000000832667, 0.1093750000000081740, 0.1171875000000081185, 0.1210937500000085210, 0.1230468750000082712, 0.1240234375000081324, 0.1250000000000079936, 0.1875000000000035805, 0.2187500000000010270, 0.2343749999999996669, 0.2421874999999990286, 0.2460937499999984734, 0.2480468749999981681, 0.2499999999999978906, 0.2812499999999959477, 0.2968749999999949485, 0.3046874999999941158, 0.3124999999999932832, 0.3749999999999866218, 0.3906249999999853451, 0.3984374999999846789, 0.4023437499999846234, 0.4062499999999845124, 0.4218749999999843459, 0.4296874999999840128, 0.4335937499999837907, 0.4355468749999836797, 0.4374999999999836242, 0.4687499999999834577, 0.4843749999999837352, 0.4999999999999839573, 0.6249999999999878986, 0.7499999999999918954, 0.8749999999999960032, 1.000000000000000000 ),
 .UNSPECIFIED. ) ;
#7344=CARTESIAN_POINT ( 'NONE',  ( -1.177014466106575785, -80.19325593536987640, 1.006209693435321739 ) ) ;
#7346=CARTESIAN_POINT ( 'NONE',  ( 1.250000000000000000, -79.25000000000000000, 0.000000000000000000 ) ) ;
#7354=CARTESIAN_POINT ( 'NONE',  ( -0.6878774159238000285, -81.72954691737999156, -1.297410027194999982 ) ) ;
#7373=CARTESIAN_POINT ( 'NONE',  ( -1.570423240223999928, -80.91589829417999624, -0.5559045111934000083 ) ) ;
#7379=CARTESIAN_POINT ( 'NONE',  ( -1.250000000000001332, -78.48958333333332860, 0.1636246173744632659 ) ) ;
#7403=CARTESIAN_POINT ( 'NONE',  ( -1.217465845835394411, -83.02083333333330017, -0.3271848554491003647 ) ) ;
#7407=CIRCLE ( 'NONE', #56429, 9.500000000000000000 ) ;
#7410=CARTESIAN_POINT ( 'NONE',  ( -0.7213013439201000354, -77.91806885964999196, -1.458901041394999876 ) ) ;
#7411=DIRECTION ( 'NONE',  ( 0.000000000000000000, 1.000000000000000000, 0.000000000000000000 ) ) ;
#7420=CARTESIAN_POINT ( 'NONE',  ( -0.2789364955927000067, -79.84686628078000581, 1.441751320050999929 ) ) ;
#7424=CARTESIAN_POINT ( 'NONE',  ( -1.561527218546999940, -82.23949528173000090, -0.5804237711334999661 ) ) ;
#7429=CARTESIAN_POINT ( 'NONE',  ( 0.8922764163254073289, -81.28868091437070120, -0.8857686078441138200 ) ) ;
#7441=CARTESIAN_POINT ( 'NONE',  ( 0.7311670807272000472, -82.16845028413999330, 1.496881327486000002 ) ) ;
#7450=CARTESIAN_POINT ( 'NONE',  ( -1.226019641078067490, -80.08489572786606914, 0.2445129742201496981 ) ) ;
#7457=CARTESIAN_POINT ( 'NONE',  ( -1.250000000000000000, -79.10000000000000853, 0.000000000000000000 ) ) ;
#7458=CARTESIAN_POINT ( 'NONE',  ( 0.6087236336976633577, -82.69146269354659751, 1.385507257417856186 ) ) ;
#7459=CARTESIAN_POINT ( 'NONE',  ( -0.4678443571040080129, -79.69481927908104524, -1.158927088315063969 ) ) ;
#7477=VERTEX_POINT ( 'NONE', #40458 ) ;
#7486=CARTESIAN_POINT ( 'NONE',  ( -1.250000000000000000, -80.00000000000000000, 0.000000000000000000 ) ) ;
#7488=CARTESIAN_POINT ( 'NONE',  ( 1.561568621681000080, -79.47054785055999560, 0.2753811681071999806 ) ) ;
#7508=CARTESIAN_POINT ( 'NONE',  ( 1.240145984052934303, -78.36013412040074400, 0.1580125328906592519 ) ) ;
#7520=B_SPLINE_CURVE_WITH_KNOTS ( 'NONE', 3,
 ( #10438, #5998, #18715, #19582, #55600, #14561, #28129, #36710, #23426, #32555, #23716, #41727, #15147, #33142, #1592, #51186, #29017, #16029, #7744, #52623, #33441, #34595, #29298, #42900, #38458, #25744, #11894, #20747, #51477, #12175, #3034, #52053, #38745, #21314, #21032, #38163, #39037, #57048, #16326, #3320, #11611, #29585, #16608, #7165, #30162, #48211, #43770, #39326, #24884, #7459, #56187, #15735, #56765, #57333, #33731, #11035, #47056, #56473, #34307, #6586, #2746, #52339, #24597, #29873, #47641, #51766, #25458, #43477, #42611, #6875, #2175, #11318 ),
 .UNSPECIFIED., .F., .F.,
 ( 4, 2, 2, 1, 1, 2, 2, 2, 2, 1, 1, 2, 2, 2, 2, 1, 1, 2, 2, 2, 2, 1, 1, 2, 2, 2, 2, 1, 1, 2, 2, 2, 2, 1, 2, 2, 2, 2, 1, 2, 2, 4 ),
 ( 0.000000000000000000, 0.06249999999999798772, 0.09374999999999730771, 0.1093749999999972800, 0.1171874999999975714, 0.1210937499999977102, 0.1249999999999978628, 0.1875000000000006661, 0.2187500000000024425, 0.2343750000000035805, 0.2421875000000041911, 0.2460937500000048017, 0.2500000000000053846, 0.3125000000000109357, 0.3437500000000133782, 0.3593750000000145994, 0.3671875000000155431, 0.3710937500000163203, 0.3750000000000170419, 0.4375000000000226485, 0.4687500000000254241, 0.4843750000000268119, 0.4921875000000275335, 0.4960937500000278666, 0.5000000000000281997, 0.5625000000000229816, 0.5937500000000199840, 0.6093750000000184297, 0.6171875000000176525, 0.6210937500000173195, 0.6250000000000169864, 0.6875000000000148770, 0.7187500000000138778, 0.7343750000000133227, 0.7421875000000127676, 0.7500000000000121014, 0.8125000000000074385, 0.8437500000000047740, 0.8593750000000034417, 0.8671875000000031086, 0.8750000000000026645, 1.000000000000000000 ),
 .UNSPECIFIED. ) ;
#7523=CARTESIAN_POINT ( 'NONE',  ( 0.1585695142483192488, -81.96550636862359340, 1.239693765617767340 ) ) ;
#7528=LINE ( 'NONE', #29368, #47622 ) ;
#7544=CARTESIAN_POINT ( 'NONE',  ( -1.217816995976848338, -82.62131526224676747, -0.3277238727207466007 ) ) ;
#7547=CARTESIAN_POINT ( 'NONE',  ( -0.9418125538657827756, -79.54291035859898784, 0.8257868174826785701 ) ) ;
#7574=EDGE_CURVE ( 'NONE', #16529, #20818, #12606, .T. ) ;
#7603=CARTESIAN_POINT ( 'NONE',  ( 0.6623344797569685749, -80.43065007664468169, 1.060132421565134431 ) ) ;
#7609=ORIENTED_EDGE ( 'NONE', *, *, #55721, .T. ) ;
#7618=CARTESIAN_POINT ( 'NONE',  ( -0.5337295926248202260, -77.94592315191539456, -1.412633301426811760 ) ) ;
#7630=CARTESIAN_POINT ( 'NONE',  ( 1.292068742513557078, -81.04347613877415313, 0.7843776082647708758 ) ) ;
#7640=CARTESIAN_POINT ( 'NONE',  ( -0.7723712723579999606, -81.22427319649999333, -1.248632555533999877 ) ) ;
#7656=FACE_OUTER_BOUND ( 'NONE', #36559, .T. ) ;
#7659=CARTESIAN_POINT ( 'NONE',  ( 1.587978134902999994, -80.60404510987000037, 0.5035716945827000135 ) ) ;
#7663=CARTESIAN_POINT ( 'NONE',  ( -1.218691819105022001, -82.12147840418360545, -0.3276751685990938467 ) ) ;
#7670=VERTEX_POINT ( 'NONE', #46075 ) ;
#7695=CARTESIAN_POINT ( 'NONE',  ( 1.250000000000000888, -81.73388662792250159, -0.2531082567149807172 ) ) ;
#7706=CARTESIAN_POINT ( 'NONE',  ( -1.542276019614999827, -82.29518551926999237, 0.7219429580085000575 ) ) ;
#7708=CARTESIAN_POINT ( 'NONE',  ( 0.7503380909894999951, -80.28898078654999892, 1.262315685543000221 ) ) ;
#7717=CARTESIAN_POINT ( 'NONE',  ( 0.2796250015563770397, -81.24281920464285633, -1.222472053442152484 ) ) ;
#7726=CARTESIAN_POINT ( 'NONE',  ( 1.611423453808999984, -81.60001734814998997, 0.4225784326546000447 ) ) ;
#7743=CARTESIAN_POINT ( 'NONE',  ( 1.348211372310171408, -82.64085315442503088, 0.7644857786683515455 ) ) ;
#7744=CARTESIAN_POINT ( 'NONE',  ( 0.9013968416950485230, -79.78949536163368350, -0.8657002453825515254 ) ) ;
#7809=CARTESIAN_POINT ( 'NONE',  ( 1.199399675185978564, -81.87278530070058480, 0.3527059046770779083 ) ) ;
#7817=EDGE_CURVE ( 'NONE', #12936, #8817, #35053, .T. ) ;
#7820=CARTESIAN_POINT ( 'NONE',  ( -1.250000000000000000, -81.99999999999998579, 0.000000000000000000 ) ) ;
#7824=VERTEX_POINT ( 'NONE', #47815 ) ;
#7852=CARTESIAN_POINT ( 'NONE',  ( 1.214377479881415978, -82.87154625297898747, 0.3342415832218785243 ) ) ;
#7859=CARTESIAN_POINT ( 'NONE',  ( 0.000000000000000000, -83.49999999999998579, 0.000000000000000000 ) ) ;
#7917=CARTESIAN_POINT ( 'NONE',  ( 1.151817246788077176, -80.55763602254313582, 1.030585181417483565 ) ) ;
#7920=DIRECTION ( 'NONE',  ( 1.000000000000000000, 0.000000000000000000, 0.000000000000000000 ) ) ;
#7927=CARTESIAN_POINT ( 'NONE',  ( 0.5770204343780001022, -82.36129654213999629, -1.476971271490000071 ) ) ;
#7941=DIRECTION ( 'NONE',  ( 0.000000000000000000, 1.000000000000000000, 0.000000000000000000 ) ) ;
#7945=CARTESIAN_POINT ( 'NONE',  ( -0.7048934085577001074, -80.91984118541999749, -1.509431780672999990 ) ) ;
#7962=CARTESIAN_POINT ( 'NONE',  ( -0.8698315184489000540, -77.71593921376999958, -1.124239518549000172 ) ) ;
#7976=ORIENTED_EDGE ( 'NONE', *, *, #13476, .F. ) ;
#7984=DIRECTION ( 'NONE',  ( 2.719057617950000092E-13, 0.000000000000000000, -1.000000000000000000 ) ) ;
#7987=DIRECTION ( 'NONE',  ( -0.9999873237594404385, 0.000000000000000000, -0.005035108780571202237 ) ) ;
#7988=CARTESIAN_POINT ( 'NONE',  ( -0.8854615841765430817, -83.03831763565791846, 0.8817396644130072181 ) ) ;
#7995=CARTESIAN_POINT ( 'NONE',  ( -1.274573384913999963, -80.41529921676999493, 0.7293221697183999153 ) ) ;
#8000=CARTESIAN_POINT ( 'NONE',  ( 1.579899301681999990, -81.98685842128999468, 0.5283722218587000308 ) ) ;
#8015=DIRECTION ( 'NONE',  ( -1.000000000000000000, 0.000000000000000000, 0.000000000000000000 ) ) ;
#8020=CARTESIAN_POINT ( 'NONE',  ( 0.2548808781567560300, -79.95924185380276583, 1.223919185308683266 ) ) ;
#8025=PLANE ( 'NONE',  #47314 ) ;
#8026=CARTESIAN_POINT ( 'NONE',  ( 0.4639995417680284895, -81.69951572676090734, 1.438848120810740872 ) ) ;
#8052=ADVANCED_FACE ( 'NONE', ( #4359 ), #17945, .F. ) ;
#8057=CARTESIAN_POINT ( 'NONE',  ( -1.578837173282999995, -79.19167545639999162, 0.3948290484592000271 ) ) ;
#8060=CARTESIAN_POINT ( 'NONE',  ( -1.217465845835394411, -78.02083333333332860, -0.3271848554491003647 ) ) ;
#8096=CARTESIAN_POINT ( 'NONE',  ( 1.129777590424469569, -81.88536348647744489, 0.5350541287706942484 ) ) ;
#8132=AXIS2_PLACEMENT_3D ( 'NONE', #18351, #13906, #8900 ) ;
#8200=CARTESIAN_POINT ( 'NONE',  ( -0.1636246173744726473, -83.38541666666664298, 1.249999999999999112 ) ) ;
#8207=CARTESIAN_POINT ( 'NONE',  ( -0.8298952231115165334, -79.92822769484411083, -1.265560781775035171 ) ) ;
#8216=CARTESIAN_POINT ( 'NONE',  ( -0.4887637738901999818, -82.04534299292998867, 1.384759226041999858 ) ) ;
#8220=CARTESIAN_POINT ( 'NONE',  ( 0.3271848554491016414, -82.14583333333331439, -1.217465845835393967 ) ) ;
#8230=CARTESIAN_POINT ( 'NONE',  ( 0.000000000000000000, -77.50000000000000000, 0.000000000000000000 ) ) ;
#8241=ORIENTED_EDGE ( 'NONE', *, *, #6996, .T. ) ;
#8250=CARTESIAN_POINT ( 'NONE',  ( 0.06134695251390999415, -79.33472580599999446, -1.460504705271000070 ) ) ;
#8257=CARTESIAN_POINT ( 'NONE',  ( 0.8515566320460936645, -80.28524471423844489, -0.9156626745943138301 ) ) ;
#8272=DIRECTION ( 'NONE',  ( 1.000000000000000000, 0.000000000000000000, 0.000000000000000000 ) ) ;
#8276=CARTESIAN_POINT ( 'NONE',  ( -1.155509423026611415, -83.06897101105678871, 0.4765901429544092682 ) ) ;
#8281=CARTESIAN_POINT ( 'NONE',  ( -1.400413196275999805, -83.43236633857299012, 0.4410028580390000230 ) ) ;
#8282=CARTESIAN_POINT ( 'NONE',  ( 0.5769282351073999893, -81.29952822830999537, 1.350407801515999928 ) ) ;
#8293=CARTESIAN_POINT ( 'NONE',  ( -0.7528178228308939346, -79.57551938009331138, -1.041016560679725478 ) ) ;
#8299=CARTESIAN_POINT ( 'NONE',  ( 0.5269479332349999989, -83.17899772590298824, 1.580352090963000000 ) ) ;
#8304=CARTESIAN_POINT ( 'NONE',  ( -0.2078146149822125144, -79.51265551170533286, -1.400962704543201154 ) ) ;
#8308=CARTESIAN_POINT ( 'NONE',  ( 1.249963906870020347, -79.86378459473635871, 0.2155801268755469513 ) ) ;
#8320=VERTEX_POINT ( 'NONE', #49699 ) ;
#8346=CARTESIAN_POINT ( 'NONE',  ( 1.250000000000000000, -78.25000000000000000, 0.000000000000000000 ) ) ;
#8363=CARTESIAN_POINT ( 'NONE',  ( 0.000000000000000000, -80.74999999950000529, 0.000000000000000000 ) ) ;
#8377=CARTESIAN_POINT ( 'NONE',  ( 0.4690275182270805532, -81.94447212118758728, 1.158641618440934051 ) ) ;
#8378=CARTESIAN_POINT ( 'NONE',  ( 1.195585824879000114, -78.14121194367999124, 1.156768630296999945 ) ) ;
#8391=CARTESIAN_POINT ( 'NONE',  ( 0.1636246173744697330, -80.13541666666665719, -1.249999999999999778 ) ) ;
#8462=ORIENTED_EDGE ( 'NONE', *, *, #11446, .T. ) ;
#8491=CARTESIAN_POINT ( 'NONE',  ( 0.3271848554490964789, -80.85416666666665719, 1.217465845835395521 ) ) ;
#8492=CARTESIAN_POINT ( 'NONE',  ( 0.9540091777473798107, -80.17115348262751695, 1.221456096381576151 ) ) ;
#8503=CARTESIAN_POINT ( 'NONE',  ( -0.6962927961685000389, -82.36145401580000680, -1.554024870232999955 ) ) ;
#8517=DIRECTION ( 'NONE',  ( 0.000000000000000000, 1.000000000000000000, 0.000000000000000000 ) ) ;
#8522=B_SPLINE_CURVE_WITH_KNOTS ( 'NONE', 3,
 ( #40925, #36197, #54215, #31156, #53621, #513, #17906, #49194, #50087, #8746, #798, #58343, #14332, #31750, #40030, #9341, #36772, #27330 ),
 .UNSPECIFIED., .F., .F.,
 ( 4, 2, 2, 2, 2, 2, 2, 2, 4 ),
 ( 0.000000000000000000, 0.1249999999999999722, 0.2500000000000000000, 0.3750000000000000000, 0.5000000000000001110, 0.6250000000000001110, 0.7500000000000000000, 0.8750000000000000000, 1.000000000000000000 ),
 .UNSPECIFIED. ) ;
#8539=CARTESIAN_POINT ( 'NONE',  ( 0.8664330213526999502, -79.10093026602000066, 1.402205237644999825 ) ) ;
#8543=CARTESIAN_POINT ( 'NONE',  ( -1.407266007596761570, -79.27925411857121674, -0.5431331937064914905 ) ) ;
#8544=CARTESIAN_POINT ( 'NONE',  ( -0.04676854649727409108, -80.22264845957727175, -1.249623885083431807 ) ) ;
#8548=EDGE_CURVE ( 'NONE', #30955, #32917, #4131, .T. ) ;
#8561=CYLINDRICAL_SURFACE ( 'NONE', #35708, 1.250000000000000000 ) ;
#8573=CARTESIAN_POINT ( 'NONE',  ( -0.6675286376147999690, -83.36920712346199025, 1.308112063971999861 ) ) ;
#8578=CARTESIAN_POINT ( 'NONE',  ( -0.7572724432162000197, -83.12372429327399459, 1.483977110291999857 ) ) ;
#8588=CARTESIAN_POINT ( 'NONE',  ( -1.508789225394999933, -82.29476871435998930, 0.7062677124845000431 ) ) ;
#8595=CARTESIAN_POINT ( 'NONE',  ( 1.277523036634464537, -77.92187500009777068, 0.4181665473888493412 ) ) ;
#8596=ORIENTED_EDGE ( 'NONE', *, *, #30941, .F. ) ;
#8599=CARTESIAN_POINT ( 'NONE',  ( 0.7287571107289755323, -79.92570316464997404, 1.016895782456411323 ) ) ;
#8600=CYLINDRICAL_SURFACE ( 'NONE', #22591, 1.250000000000000000 ) ;
#8625=CARTESIAN_POINT ( 'NONE',  ( 1.139330238168773324, -79.38420227355845782, 0.5135602714818040537 ) ) ;
#8673=CARTESIAN_POINT ( 'NONE',  ( 0.4455676568320503517, -81.94613279277081119, 1.167930216820072920 ) ) ;
#8674=CARTESIAN_POINT ( 'NONE',  ( -0.1648886907344999930, -77.77763659747000702, 1.456783013396000248 ) ) ;
#8686=CYLINDRICAL_SURFACE ( 'NONE', #33710, 2.500000000000000000 ) ;
#8727=EDGE_LOOP ( 'NONE', ( #26003, #36730, #31571, #43402 ) ) ;
#8746=CARTESIAN_POINT ( 'NONE',  ( 0.1636246173744642929, -82.36458333333334281, 1.250000000000000888 ) ) ;
#8755=FACE_OUTER_BOUND ( 'NONE', #52488, .T. ) ;
#8785=CARTESIAN_POINT ( 'NONE',  ( -1.217465845835396188, -83.47916666666668561, 0.3271848554490955907 ) ) ;
#8792=CARTESIAN_POINT ( 'NONE',  ( -0.1058354079650530299, -79.96871532614137834, -1.507746398707539681 ) ) ;
#8802=CARTESIAN_POINT ( 'NONE',  ( -1.631971144587999856, -81.79302107981000347, -0.4862994432698999892 ) ) ;
#8803=ORIENTED_EDGE ( 'NONE', *, *, #34070, .T. ) ;
#8817=VERTEX_POINT ( 'NONE', #28181 ) ;
#8826=CARTESIAN_POINT ( 'NONE',  ( -0.3164372427141999844, -79.77903242220000379, 1.635583079321000000 ) ) ;
#8836=ORIENTED_EDGE ( 'NONE', *, *, #22873, .F. ) ;
#8840=CARTESIAN_POINT ( 'NONE',  ( -0.9392528719664000603, -77.77925590253998678, -1.213965203811000038 ) ) ;
#8844=CARTESIAN_POINT ( 'NONE',  ( 1.165063941761719013, -80.32067678519440790, -0.4527090129185701306 ) ) ;
#8868=CARTESIAN_POINT ( 'NONE',  ( -0.5103843434498001042, -83.05341104791099838, -1.376937268564000005 ) ) ;
#8869=CARTESIAN_POINT ( 'NONE',  ( 1.330733645151999989, -79.78386453932999700, 0.2346736355698000043 ) ) ;
#8876=EDGE_CURVE ( 'NONE', #25256, #10113, #7407, .T. ) ;
#8894=CARTESIAN_POINT ( 'NONE',  ( 0.5875992245590921925, -79.93626096961999394, 1.106550443725125232 ) ) ;
#8900=DIRECTION ( 'NONE',  ( -1.000000000000000000, 0.000000000000000000, 0.000000000000000000 ) ) ;
#8909=LINE ( 'NONE', #88, #12954 ) ;
#8919=CARTESIAN_POINT ( 'NONE',  ( 0.3278620359192580547, -82.45482759320131549, 1.218429155783411044 ) ) ;
#8936=VECTOR ( 'NONE', #52119, 1000.000000000000000 ) ;
#8958=DIRECTION ( 'NONE',  ( 0.000000000000000000, 1.000000000000000000, -1.561587422443000175E-14 ) ) ;
#8974=CARTESIAN_POINT ( 'NONE',  ( 0.6544915521845998674, -81.11326172198998563, 1.531959166345999934 ) ) ;
#8975=CARTESIAN_POINT ( 'NONE',  ( -1.497311080048000065, -78.87270746980999547, 0.3971898337434000004 ) ) ;
#8978=CARTESIAN_POINT ( 'NONE',  ( 1.501514506084554723, -82.48075314929823776, -0.3793901851540854020 ) ) ;
#8983=CARTESIAN_POINT ( 'NONE',  ( 1.079681942422447305, -81.80797850944155414, -0.6305161809801804740 ) ) ;
#8992=CARTESIAN_POINT ( 'NONE',  ( -1.391457981517000064, -78.65970746980998740, -0.2902696593763000044 ) ) ;
#9014=CARTESIAN_POINT ( 'NONE',  ( -1.273831304311999979, -80.60709877522999989, -0.4509157470602000450 ) ) ;
#9051=CARTESIAN_POINT ( 'NONE',  ( 0.000000000000000000, -76.75499999999999545, 0.000000000000000000 ) ) ;
#9091=CARTESIAN_POINT ( 'NONE',  ( 0.5010153433495700970, -81.00114992422807347, -1.428186821674153117 ) ) ;
#9092=CARTESIAN_POINT ( 'NONE',  ( -1.249848728141158993, -78.59781426991139597, 0.03830777415639201322 ) ) ;
#9101=CARTESIAN_POINT ( 'NONE',  ( -0.5277720668919000380, -82.10865968170000428, 1.495277019118000039 ) ) ;
#9105=DIRECTION ( 'NONE',  ( 0.000000000000000000, -1.000000000000000000, 0.000000000000000000 ) ) ;
#9124=CARTESIAN_POINT ( 'NONE',  ( 0.8512149552595998925, -80.22114692796999691, 1.432023780608000063 ) ) ;
#9138=CARTESIAN_POINT ( 'NONE',  ( -1.062134069330999964, -79.14247671680999474, 1.107996173502999948 ) ) ;
#9143=CARTESIAN_POINT ( 'NONE',  ( 1.174637156278667494, -80.32243980880512879, -0.4274726629302632586 ) ) ;
#9167=CARTESIAN_POINT ( 'NONE',  ( 1.467208996055999748, -82.67429828359199462, 0.6014104092625999209 ) ) ;
#9168=CARTESIAN_POINT ( 'NONE',  ( 0.3004848064042999756, -80.16281982998998501, -1.317452118262000038 ) ) ;
#9202=ORIENTED_EDGE ( 'NONE', *, *, #6956, .F. ) ;
#9210=EDGE_CURVE ( 'NONE', #48909, #20818, #41364, .T. ) ;
#9227=CARTESIAN_POINT ( 'NONE',  ( -0.8961266428360998848, -77.69180782643999805, 1.358359200922999888 ) ) ;
#9264=B_SPLINE_SURFACE_WITH_KNOTS ( 'NONE', 3, 3, ( 
 ( #57936, #30484, #31049, #48510, #8057, #35781, #12767, #44077, #49084, #53810, #3626, #30763, #39922, #40810, #693, #31639, #28379, #14224, #46425, #5376, #27213, #5092, #45251, #46137, #13644, #18675, #50847, #37245, #54966, #13937, #32222, #5660, #27506, #5954, #36666 ),
 ( #54682, #50264, #23088, #9812, #23384, #23956, #23670, #22801, #41683, #1263, #978, #41976, #27797, #32799, #402, #4800, #36083, #19250, #18380, #55257, #18090, #10393, #41395, #41101, #45841, #14806, #18961, #36955, #54102, #49682, #14517, #31932, #9227, #32509, #36373 ),
 ( #54399, #49976, #10106, #9519, #50554, #28086, #45547, #56143, #56431, #15690, #6243, #47011, #7124, #11849, #29828, #56721, #33098, #42564, #24260, #25414, #42276, #37831, #37534, #34258, #38411, #38700, #47879, #11276, #16278, #7410, #33972, #52290, #47597, #51434, #47303 ),
 ( #55551, #2130, #1547, #20702, #15982, #55851, #33686, #25124, #10988, #19539, #20131, #15403, #28673, #43148, #38119, #33396, #15101, #52010, #51142, #6541, #19836, #29542, #2707, #28969, #1844, #10696, #51724, #46727, #29254, #24550, #6829, #24841, #42855, #11564, #2415 ) ),
 .UNSPECIFIED., .F., .F., .F.,
 ( 4, 4 ),
 ( 4, 1, 1, 1, 1, 1, 1, 1, 1, 1, 1, 1, 1, 1, 1, 1, 1, 1, 1, 1, 1, 1, 1, 1, 1, 1, 1, 1, 1, 1, 1, 1, 4 ),
 ( -0.3882448580381000491, 1.388244858038000018 ),
 ( -0.01763212848115999765, 0.01102008030072000079, 0.03967228908261000164, 0.06832449786448999141, 0.09697670664638000093, 0.1256289154283000142, 0.1542811242101000124, 0.1829333329919999862, 0.2115855417738999877, 0.2402377505557999893, 0.2688899593376999908, 0.2975421681195999923, 0.3261943769014999939, 0.3548465856833000198, 0.3834987944651999658, 0.4121510032471000229, 0.4408032120290000244, 0.4694554208109000260, 0.4981076295927999720, 0.5267598383746000534, 0.5554120471565000550, 0.5840642559384000565, 0.6127164647203000580, 0.6413686735021999485, 0.6700208822840999501, 0.6986730910659999516, 0.7273252998478000331, 0.7559775086296999236, 0.7846297174115999251, 0.8132819261935000377, 0.8419341349753999282, 0.8705863437573000407, 0.8992385525391000112 ),
 .UNSPECIFIED. ) ;
#9266=CARTESIAN_POINT ( 'NONE',  ( -0.5298108134926000634, -80.67114721621999252, 1.579417458585999912 ) ) ;
#9267=CARTESIAN_POINT ( 'NONE',  ( -1.391730330000000126, -79.43715828658999101, 0.3480381455443000149 ) ) ;
#9269=CARTESIAN_POINT ( 'NONE',  ( 0.8225791642732954712, -82.42002313476852748, -1.311939220806510153 ) ) ;
#9275=CARTESIAN_POINT ( 'NONE',  ( 1.001278227489189598, -81.79905685887599986, -0.7511161502827685688 ) ) ;
#9285=CARTESIAN_POINT ( 'NONE',  ( 1.249765501161204995, -80.36036749726001460, 0.1566955736949024458 ) ) ;
#9304=CARTESIAN_POINT ( 'NONE',  ( 1.367321113498000118, -80.92305232442998886, 0.5356168500207999505 ) ) ;
#9306=CARTESIAN_POINT ( 'NONE',  ( -0.8944171124340070111, -79.16181922138737548, -0.8730969871168202667 ) ) ;
#9341=CARTESIAN_POINT ( 'NONE',  ( 1.217465845835393967, -82.27083333333331439, 0.3271848554491025851 ) ) ;
#9355=EDGE_LOOP ( 'NONE', ( #44774, #40275, #17545, #42761 ) ) ;
#9361=CARTESIAN_POINT ( 'NONE',  ( 1.227045062450840884, -82.83502415505597583, -0.2377312851286680906 ) ) ;
#9364=AXIS2_PLACEMENT_3D ( 'NONE', #146, #44690, #31081 ) ;
#9378=CARTESIAN_POINT ( 'NONE',  ( 0.000000000000000000, -86.20000000000000284, 0.000000000000000000 ) ) ;
#9386=CARTESIAN_POINT ( 'NONE',  ( -0.7681833999686477066, -80.92708333333332860, 0.9995835529977223910 ) ) ;
#9388=CYLINDRICAL_SURFACE ( 'NONE', #9534, 1.250000000000000000 ) ;
#9389=CARTESIAN_POINT ( 'NONE',  ( -1.546786622596739047, -80.35334782346511417, -0.08660658759117148553 ) ) ;
#9390=CARTESIAN_POINT ( 'NONE',  ( -0.1873428942460613755, -78.48719004869164451, 1.238278019793636942 ) ) ;
#9433=CARTESIAN_POINT ( 'NONE',  ( 1.409966096066999963, -77.98898218165999197, 0.6064444106313999772 ) ) ;
#9435=CARTESIAN_POINT ( 'NONE',  ( 0.8901331092129259881, -80.28864483123025764, -0.8771058481484877989 ) ) ;
#9460=CARTESIAN_POINT ( 'NONE',  ( -0.6256353049379000941, -82.80061671381200483, 1.457043991488000012 ) ) ;
#9462=CARTESIAN_POINT ( 'NONE',  ( -0.9995835529977281642, -79.44791666666662877, 0.7681833999686391579 ) ) ;
#9478=CARTESIAN_POINT ( 'NONE',  ( 1.209853131585020947, -79.32753753103162353, -0.3581602740580526190 ) ) ;
#9490=EDGE_CURVE ( 'NONE', #48229, #45641, #48883, .T. ) ;
#9511=EDGE_LOOP ( 'NONE', ( #57928, #47001, #26601, #18869 ) ) ;
#9512=EDGE_CURVE ( 'NONE', #10113, #25387, #43245, .T. ) ;
#9519=CARTESIAN_POINT ( 'NONE',  ( -1.462188802161999979, -79.36578967391999129, -0.7147474581103999691 ) ) ;
#9534=AXIS2_PLACEMENT_3D ( 'NONE', #46295, #32668, #23536 ) ;
#9559=CARTESIAN_POINT ( 'NONE',  ( 0.8512149552595998925, -80.04349795635999953, 1.432023780608000063 ) ) ;
#9560=CARTESIAN_POINT ( 'NONE',  ( -0.8715281638271999975, -78.31589177200999075, 1.280679076496999969 ) ) ;
#9562=CARTESIAN_POINT ( 'NONE',  ( -1.499047393880830858, -83.23987833091183575, 0.1907839512157355755 ) ) ;
#9563=DIRECTION ( 'NONE',  ( 0.000000000000000000, 1.000000000000000000, 0.000000000000000000 ) ) ;
#9566=EDGE_CURVE ( 'NONE', #16901, #45372, #14946, .T. ) ;
#9574=VERTEX_POINT ( 'NONE', #49014 ) ;
#9591=CARTESIAN_POINT ( 'NONE',  ( 1.092232985442820992, -81.29166666666665719, 0.6295237254636267821 ) ) ;
#9597=CARTESIAN_POINT ( 'NONE',  ( -1.322249586278000155, -79.59655133345999900, -0.2786171024073000324 ) ) ;
#9606=CARTESIAN_POINT ( 'NONE',  ( 1.250000000000000000, -79.25000000000000000, 0.000000000000000000 ) ) ;
#9610=CARTESIAN_POINT ( 'NONE',  ( 1.217465845835394855, -79.22916666666665719, -0.3271848554490981997 ) ) ;
#9645=ORIENTED_EDGE ( 'NONE', *, *, #38085, .F. ) ;
#9674=CARTESIAN_POINT ( 'NONE',  ( -0.3862712429687000237, -78.00000000000000000, 1.188820645369000006 ) ) ;
#9679=CARTESIAN_POINT ( 'NONE',  ( -1.474633671607979091, -79.86749624789827351, -0.3407938052334066326 ) ) ;
#9688=CARTESIAN_POINT ( 'NONE',  ( 0.3767945000176999848, -81.35074910037999985, -1.540381938526000027 ) ) ;
#9721=CARTESIAN_POINT ( 'NONE',  ( -1.250000000000000000, -78.50000000000000000, 0.000000000000000000 ) ) ;
#9722=CARTESIAN_POINT ( 'NONE',  ( 1.162219475002999935, -78.51329787945999783, 1.002509651144999792 ) ) ;
#9726=CARTESIAN_POINT ( 'NONE',  ( -1.154538933705213211, -80.13146567447462587, -0.4788082789554529706 ) ) ;
#9750=CARTESIAN_POINT ( 'NONE',  ( 0.6120151737828000149, -80.85757119619998434, 1.204744225600999918 ) ) ;
#9751=CARTESIAN_POINT ( 'NONE',  ( 0.3271848554490964789, -79.35416666666667140, 1.217465845835395521 ) ) ;
#9752=CARTESIAN_POINT ( 'NONE',  ( -0.6295237254636286695, -82.91666666666667140, 1.092232985442819881 ) ) ;
#9761=AXIS2_PLACEMENT_3D ( 'NONE', #8230, #30071, #22089 ) ;
#9775=EDGE_CURVE ( 'NONE', #32332, #13850, #333, .T. ) ;
#9776=CARTESIAN_POINT ( 'NONE',  ( -0.9682055199207542096, -81.54584953990853080, 0.7910361119925342077 ) ) ;
#9788=ADVANCED_FACE ( 'NONE', ( #4731 ), #8561, .F. ) ;
#9792=B_SPLINE_CURVE_WITH_KNOTS ( 'NONE', 3,
 ( #52262, #7379, #43395, #56972, #43695, #16824, #39243, #12101, #42538, #7095, #34807, #38382, #20104, #52831, #12387, #33658, #11247, #51699 ),
 .UNSPECIFIED., .F., .F.,
 ( 4, 2, 2, 2, 2, 2, 2, 2, 4 ),
 ( 0.000000000000000000, 0.1249999999999999722, 0.2500000000000000000, 0.3750000000000000000, 0.5000000000000001110, 0.6250000000000001110, 0.7500000000000000000, 0.8750000000000000000, 1.000000000000000000 ),
 .UNSPECIFIED. ) ;
#9794=DIRECTION ( 'NONE',  ( -1.000000000000000000, 0.000000000000000000, 0.000000000000000000 ) ) ;
#9812=CARTESIAN_POINT ( 'NONE',  ( -1.462188802161999979, -79.30657335004998743, -0.7147474581103999691 ) ) ;
#9841=CARTESIAN_POINT ( 'NONE',  ( -0.7803569495551999635, -81.85659709982999743, -1.471836271561000054 ) ) ;
#9847=CARTESIAN_POINT ( 'NONE',  ( -1.249474801850635419, -81.11011701208103375, -0.1486004900664459893 ) ) ;
#9853=CARTESIAN_POINT ( 'NONE',  ( -1.570423240223999928, -80.73824932256999887, -0.5559045111934000083 ) ) ;
#9854=CARTESIAN_POINT ( 'NONE',  ( -1.209673032756999778, -78.05275416108999309, -0.5285249375785000536 ) ) ;
#9856=CARTESIAN_POINT ( 'NONE',  ( -1.527490045409469532, -82.23783309118122986, 0.2444902829799560084 ) ) ;
#9857=CARTESIAN_POINT ( 'NONE',  ( 1.476436775452767192, -83.11658282216879456, 0.3241340806173243494 ) ) ;
#9861=CARTESIAN_POINT ( 'NONE',  ( -0.3392593397791182075, -81.70348311923245888, -1.202985507264590304 ) ) ;
#9864=LINE ( 'NONE', #19306, #35587 ) ;
#9883=CARTESIAN_POINT ( 'NONE',  ( -1.092232985442824100, -81.45833333333328596, 0.6295237254636200097 ) ) ;
#9887=DIRECTION ( 'NONE',  ( -1.000000000000000000, 0.000000000000000000, 2.817678007057000277E-14 ) ) ;
#9890=CARTESIAN_POINT ( 'NONE',  ( -1.359874270581000077, -81.11252996976000418, 0.5545210745837000355 ) ) ;
#9916=CYLINDRICAL_SURFACE ( 'NONE', #39135, 1.250000000000000000 ) ;
#9919=FACE_OUTER_BOUND ( 'NONE', #41966, .T. ) ;
#9926=ORIENTED_EDGE ( 'NONE', *, *, #23548, .F. ) ;
#9965=DIRECTION ( 'NONE',  ( -1.000000000000000000, 0.000000000000000000, 0.000000000000000000 ) ) ;
#9966=CARTESIAN_POINT ( 'NONE',  ( 0.5200116074403198230, -79.65885271342665419, -1.150702922115795612 ) ) ;
#9967=CARTESIAN_POINT ( 'NONE',  ( -1.053645312779857068, -83.05505849742939972, 0.6765476259604800147 ) ) ;
#9971=CARTESIAN_POINT ( 'NONE',  ( -1.164523129836848581, -78.06680908019323795, 0.5225932405203995712 ) ) ;
#9976=CARTESIAN_POINT ( 'NONE',  ( 1.363667439983781371, -79.56383901316905849, -0.6545495444765823123 ) ) ;
#9999=ORIENTED_EDGE ( 'NONE', *, *, #3856, .F. ) ;
#10013=VERTEX_POINT ( 'NONE', #38703 ) ;
#10024=CARTESIAN_POINT ( 'NONE',  ( -0.9677429597868729694, -80.15535212655082375, -0.7945947339589979341 ) ) ;
#10027=CARTESIAN_POINT ( 'NONE',  ( 1.495278353479605249, -78.08869844104306424, -0.2055598165236604546 ) ) ;
#10047=CARTESIAN_POINT ( 'NONE',  ( 1.160935205181999885, -81.72722500425999215, -0.6914862246935000734 ) ) ;
#10050=CARTESIAN_POINT ( 'NONE',  ( -0.9995835529977281642, -82.94791666666661456, 0.7681833999686391579 ) ) ;
#10074=CARTESIAN_POINT ( 'NONE',  ( -0.8938566341920096692, -81.53894037312349496, 0.8733612504233605467 ) ) ;
#10079=CARTESIAN_POINT ( 'NONE',  ( 1.306140625255000076, -78.33423293213999727, 0.06913166271809000063 ) ) ;
#10081=CIRCLE ( 'NONE', #5349, 10.14999999999999858 ) ;
#10106=CARTESIAN_POINT ( 'NONE',  ( -0.6580604922749000441, -79.42147124369999744, -1.488334326434000099 ) ) ;
#10113=VERTEX_POINT ( 'NONE', #2991 ) ;
#10131=CYLINDRICAL_SURFACE ( 'NONE', #13634, 3.000000000000000000 ) ;
#10146=CARTESIAN_POINT ( 'NONE',  ( -0.5432945554243000519, -81.36589858243000606, -1.398152719143000100 ) ) ;
#10147=CARTESIAN_POINT ( 'NONE',  ( 0.3509080281557999670, -79.16638555667999810, -1.272612056386999813 ) ) ;
#10149=CARTESIAN_POINT ( 'NONE',  ( -0.6588690626962807606, -81.66089795315696165, 1.359795660138139350 ) ) ;
#10156=DIRECTION ( 'NONE',  ( 0.000000000000000000, 0.000000000000000000, 1.000000000000000000 ) ) ;
#10183=CARTESIAN_POINT ( 'NONE',  ( 1.476447168807000221, -80.98636901320000447, 0.5783644924166000401 ) ) ;
#10195=CARTESIAN_POINT ( 'NONE',  ( 0.6295237254636258939, -79.16666666666665719, -1.092232985442821658 ) ) ;
#10213=CARTESIAN_POINT ( 'NONE',  ( -0.6295237254636235624, -82.58333333333332860, -1.092232985442822990 ) ) ;
#10219=ORIENTED_EDGE ( 'NONE', *, *, #51188, .F. ) ;
#10220=ORIENTED_EDGE ( 'NONE', *, *, #37768, .T. ) ;
#10228=ADVANCED_FACE ( 'NONE', ( #48446 ), #17828, .T. ) ;
#10234=ORIENTED_EDGE ( 'NONE', *, *, #40514, .T. ) ;
#10254=CARTESIAN_POINT ( 'NONE',  ( 0.000000000000000000, -86.20000000000000284, -9.950000000000001066 ) ) ;
#10256=CARTESIAN_POINT ( 'NONE',  ( 0.1216125091987902140, -82.96767066915866451, 1.244084642679034625 ) ) ;
#10273=ORIENTED_EDGE ( 'NONE', *, *, #25310, .F. ) ;
#10277=CYLINDRICAL_SURFACE ( 'NONE', #46942, 1.250000000000000000 ) ;
#10280=CONICAL_SURFACE ( 'NONE', #17820, 10.04999999996000071, 0.7853981633972997312 ) ;
#10282=CARTESIAN_POINT ( 'NONE',  ( -1.588687380433000174, -83.36453247999199334, 0.5002921117598999601 ) ) ;
#10312=CARTESIAN_POINT ( 'NONE',  ( -1.408973282649000014, -77.73770945175000691, 0.6047956624285000249 ) ) ;
#10314=CARTESIAN_POINT ( 'NONE',  ( -0.4716021410008969794, -80.19438574499905314, -1.157506175934070347 ) ) ;
#10318=CARTESIAN_POINT ( 'NONE',  ( 1.258015307303396391, -78.05300461876107931, -0.8356367902642429790 ) ) ;
#10332=CARTESIAN_POINT ( 'NONE',  ( 1.307088170492999968, -81.79038421936999725, 0.3427697847655999941 ) ) ;
#10336=DIRECTION ( 'NONE',  ( -1.000000000000000000, 0.000000000000000000, 0.000000000000000000 ) ) ;
#10353=EDGE_LOOP ( 'NONE', ( #20691, #48047, #2107, #33802, #53937 ) ) ;
#10359=CARTESIAN_POINT ( 'NONE',  ( -1.219338165725585066, -81.58269073872453703, 0.2774308609236747492 ) ) ;
#10363=CARTESIAN_POINT ( 'NONE',  ( -0.1995282058519000090, -77.96721194367999885, 1.292660429007000067 ) ) ;
#10393=CARTESIAN_POINT ( 'NONE',  ( -1.481905647302000029, -78.30430509401999473, -0.6727694308694001091 ) ) ;
#10395=CARTESIAN_POINT ( 'NONE',  ( -0.6813111686677723045, -79.17942873427989525, -1.051713183095109416 ) ) ;
#10403=CARTESIAN_POINT ( 'NONE',  ( 1.449190734180999973, -80.03602897879000011, -0.8942388842271000726 ) ) ;
#10432=CARTESIAN_POINT ( 'NONE',  ( -0.6332123272625999055, -81.23563726096999460, 1.540853336418999797 ) ) ;
#10435=CARTESIAN_POINT ( 'NONE',  ( -0.5897947633678554125, -81.84308799674356294, -1.392029655722818671 ) ) ;
#10438=CARTESIAN_POINT ( 'NONE',  ( 1.250000000000000000, -79.84999999999999432, 0.000000000000000000 ) ) ;
#10440=CARTESIAN_POINT ( 'NONE',  ( 0.1765468244193108827, -81.73664919909492710, -1.237851851414618176 ) ) ;
#10453=DIRECTION ( 'NONE',  ( 0.000000000000000000, -1.000000000000000000, -1.369275063704000118E-14 ) ) ;
#10465=CARTESIAN_POINT ( 'NONE',  ( -1.217465845835396188, -81.47916666666668561, 0.3271848554490955907 ) ) ;
#10471=CARTESIAN_POINT ( 'NONE',  ( 0.3265465218672000125, -79.78618645244999641, -1.431717670164000200 ) ) ;
#10475=CARTESIAN_POINT ( 'NONE',  ( -0.8293389441169838339, -79.82887584819658855, -1.264652115086847939 ) ) ;
#10485=CARTESIAN_POINT ( 'NONE',  ( -0.1636246173744673738, -79.11458333333331439, -1.249999999999999778 ) ) ;
#10498=DIRECTION ( 'NONE',  ( -1.000000000000000000, 0.000000000000000000, 0.000000000000000000 ) ) ;
#10553=CARTESIAN_POINT ( 'NONE',  ( 1.065041349166195195, -82.89404281940629460, 0.6558440019770916951 ) ) ;
#10561=CARTESIAN_POINT ( 'NONE',  ( -0.03126777369098861226, -79.47274184274870379, -1.511873468966818734 ) ) ;
#10567=( NAMED_UNIT ( * ) PLANE_ANGLE_UNIT ( ) SI_UNIT ( $, .RADIAN. ) );
#10578=CARTESIAN_POINT ( 'NONE',  ( -0.8762103189736000219, -81.46975602669000693, -1.416501064863000092 ) ) ;
#10596=CARTESIAN_POINT ( 'NONE',  ( -1.217612721212264049, -80.58218577482048772, 0.2845431953339345177 ) ) ;
#10605=CARTESIAN_POINT ( 'NONE',  ( -1.541801436820000148, -77.75518664167998395, 0.2953501223290999622 ) ) ;
#10612=DIRECTION ( 'NONE',  ( 0.000000000000000000, -0.7071067811866525998, -0.7071067811864425456 ) ) ;
#10614=CARTESIAN_POINT ( 'NONE',  ( 0.6984937801707818972, -79.18628347620142449, 1.337435529320990302 ) ) ;
#10632=CARTESIAN_POINT ( 'NONE',  ( -0.6295237254636286695, -78.91666666666665719, 1.092232985442819881 ) ) ;
#10639=CARTESIAN_POINT ( 'NONE',  ( 0.5739952604901000788, -82.73993688548499392, -1.223314898041000021 ) ) ;
#10642=EDGE_CURVE ( 'NONE', #55505, #22441, #11220, .T. ) ;
#10650=CARTESIAN_POINT ( 'NONE',  ( -0.5870567661726286968, -79.18616477877183968, -1.103542300118057984 ) ) ;
#10668=CARTESIAN_POINT ( 'NONE',  ( 0.7508852574861999418, -78.75368549038000765, -1.070959314402999851 ) ) ;
#10681=CARTESIAN_POINT ( 'NONE',  ( 1.249647686960656756, -82.36107796002586667, 0.1638768531599422151 ) ) ;
#10696=CARTESIAN_POINT ( 'NONE',  ( 1.169626569868999821, -78.20001146263999203, 1.131652196797999999 ) ) ;
#10736=CARTESIAN_POINT ( 'NONE',  ( 0.8512149552595998925, -80.10271428023000340, 1.432023780608000063 ) ) ;
#10737=CARTESIAN_POINT ( 'NONE',  ( 0.9221831299987999220, -79.33343026601998815, 0.9445928090476000127 ) ) ;
#10740=CARTESIAN_POINT ( 'NONE',  ( 1.250000000000000000, -82.74999999999998579, 0.000000000000000000 ) ) ;
#10746=CARTESIAN_POINT ( 'NONE',  ( 0.4716226049498870587, -81.75588184218486276, -1.157571032113124954 ) ) ;
#10764=CARTESIAN_POINT ( 'NONE',  ( 0.3271848554490964789, -81.35416666666667140, 1.217465845835395521 ) ) ;
#10770=CARTESIAN_POINT ( 'NONE',  ( -1.418768848999000021, -79.72334218465999811, 0.9417588900106000915 ) ) ;
#10775=CARTESIAN_POINT ( 'NONE',  ( -1.118026905147402328, -79.80863251002027425, -1.015872027318809101 ) ) ;
#10789=CARTESIAN_POINT ( 'NONE',  ( -0.001976671226007847143, -78.47534806730480739, 1.249865324143346168 ) ) ;
#10794=CARTESIAN_POINT ( 'NONE',  ( 1.250000000000000000, -79.34999999999999432, 0.000000000000000000 ) ) ;
#10804=DIRECTION ( 'NONE',  ( 0.000000000000000000, 1.000000000000000000, 0.000000000000000000 ) ) ;
#10813=CONICAL_SURFACE ( 'NONE', #43804, 2.949999999500999781, 0.7853981633972997312 ) ;
#10828=CARTESIAN_POINT ( 'NONE',  ( -0.9992933932515307704, -82.65243683341363123, -0.7674328717235032737 ) ) ;
#10833=CARTESIAN_POINT ( 'NONE',  ( 0.8523209396086280920, -78.42219961258000183, -1.272697597679407933 ) ) ;
#10853=CARTESIAN_POINT ( 'NONE',  ( 0.4492946238560011629, -82.94576776959728193, 1.166509796814039213 ) ) ;
#10860=DIRECTION ( 'NONE',  ( 1.996950752507999982E-10, 1.000000000000000000, -5.653827411922000189E-11 ) ) ;
#10864=DIRECTION ( 'NONE',  ( 1.000000000000000000, 0.000000000000000000, 0.000000000000000000 ) ) ;
#10867=FILL_AREA_STYLE ('',( #37993 ) ) ;
#10878=CARTESIAN_POINT ( 'NONE',  ( 0.6304340365998000184, -82.73294032889000960, 1.542015542100000136 ) ) ;
#10881=ORIENTED_EDGE ( 'NONE', *, *, #53680, .F. ) ;
#10882=DIRECTION ( 'NONE',  ( 0.000000000000000000, -1.000000000000000000, 0.000000000000000000 ) ) ;
#10896=CARTESIAN_POINT ( 'NONE',  ( 0.8387602819694093270, -80.41695080943928531, 0.9265839650083794732 ) ) ;
#10911=CARTESIAN_POINT ( 'NONE',  ( 0.2177847895985361160, -79.21305384291285634, 1.494441264229401378 ) ) ;
#10928=CARTESIAN_POINT ( 'NONE',  ( -1.250000000000000000, -82.99999999999998579, 0.000000000000000000 ) ) ;
#10934=CARTESIAN_POINT ( 'NONE',  ( 1.281517705925000028, -81.85570787394000547, 0.4285832374949000156 ) ) ;
#10953=CARTESIAN_POINT ( 'NONE',  ( 0.8649096616148368444, -81.41463932042252338, 0.9021248153222395372 ) ) ;
#10958=CARTESIAN_POINT ( 'NONE',  ( -1.108895999262000220, -78.12450665301999209, -0.6936369237491999407 ) ) ;
#10969=EDGE_CURVE ( 'NONE', #29213, #12675, #27247, .T. ) ;
#10981=VERTEX_POINT ( 'NONE', #29633 ) ;
#10988=CARTESIAN_POINT ( 'NONE',  ( 1.619712389308999967, -79.14659814888999279, 0.1587296492880999887 ) ) ;
#10995=CARTESIAN_POINT ( 'NONE',  ( -1.418768848999000021, -79.78339211834999389, 0.9417588900106000915 ) ) ;
#11021=CARTESIAN_POINT ( 'NONE',  ( -1.250000000000000000, -80.09999999999999432, 0.000000000000000000 ) ) ;
#11024=CARTESIAN_POINT ( 'NONE',  ( -0.4796072403373097814, -80.00656463011694086, 1.154180156579423189 ) ) ;
#11030=CARTESIAN_POINT ( 'NONE',  ( -1.194132053304999941, -79.05502241712000000, -0.5627846202731000558 ) ) ;
#11032=CARTESIAN_POINT ( 'NONE',  ( 0.6447284801462368486, -81.59004626953988293, 1.368070997584296844 ) ) ;
#11035=CARTESIAN_POINT ( 'NONE',  ( -0.8005651750373993236, -79.66990695520425447, -0.9602051216220701679 ) ) ;
#11039=CARTESIAN_POINT ( 'NONE',  ( -0.09604542572962751490, -81.71951835724753721, -1.248441681024932803 ) ) ;
#11040=FILL_AREA_STYLE ('',( #51482 ) ) ;
#11056=ORIENTED_EDGE ( 'NONE', *, *, #23435, .F. ) ;
#11067=CARTESIAN_POINT ( 'NONE',  ( -1.639384890095999969, -80.29177512065000144, -0.4606887641594999971 ) ) ;
#11080=CARTESIAN_POINT ( 'NONE',  ( 0.000000000000000000, -86.20000000000000284, 0.000000000000000000 ) ) ;
#11086=CARTESIAN_POINT ( 'NONE',  ( -0.0002385852177439338659, -78.47523597995287048, 1.249867994843831376 ) ) ;
#11101=CARTESIAN_POINT ( 'NONE',  ( 1.250000000000000000, -82.74999999999998579, 0.000000000000000000 ) ) ;
#11111=ORIENTED_EDGE ( 'NONE', *, *, #55225, .F. ) ;
#11124=DIRECTION ( 'NONE',  ( 1.000000000000000000, 0.000000000000000000, 0.000000000000000000 ) ) ;
#11127=CARTESIAN_POINT ( 'NONE',  ( -0.06629182480466444538, -78.37178464163872604, -1.530081213047539634 ) ) ;
#11147=CARTESIAN_POINT ( 'NONE',  ( 0.1634127036930090315, -82.96491418332730916, 1.239110987847197531 ) ) ;
#11150=CARTESIAN_POINT ( 'NONE',  ( -1.250000000000000000, -80.49999999999998579, 0.000000000000000000 ) ) ;
#11166=CARTESIAN_POINT ( 'NONE',  ( 0.000000000000000000, -76.75499999999999545, 0.000000000000000000 ) ) ;
#11170=CARTESIAN_POINT ( 'NONE',  ( 0.6062141276560999437, -82.54346268355999428, -1.551696954864999922 ) ) ;
#11179=CARTESIAN_POINT ( 'NONE',  ( 0.07163746727446854146, -80.73022344930195970, -1.248029480940866520 ) ) ;
#11180=ORIENTED_EDGE ( 'NONE', *, *, #48851, .F. ) ;
#11186=CARTESIAN_POINT ( 'NONE',  ( 0.9073035717151847201, -80.41100119561156134, 0.8599128470893483422 ) ) ;
#11202=CARTESIAN_POINT ( 'NONE',  ( -0.8490343226412601085, -78.42778975272105413, -1.282990012170490690 ) ) ;
#11213=CARTESIAN_POINT ( 'NONE',  ( -0.9485035383083301186, -80.67909605160095055, 1.175018830168555128 ) ) ;
#11220=CIRCLE ( 'NONE', #15962, 1.250000000000000000 ) ;
#11223=CARTESIAN_POINT ( 'NONE',  ( 1.204186364734999959, -81.79254865883000036, -0.6131120777826000179 ) ) ;
#11227=CARTESIAN_POINT ( 'NONE',  ( -0.2199206942898871697, -79.42994573680664416, -1.482330506908097201 ) ) ;
#11235=EDGE_CURVE ( 'NONE', #25256, #28446, #40541, .T. ) ;
#11241=CARTESIAN_POINT ( 'NONE',  ( -0.01395791329646856385, -81.47639348663375358, 1.249632885952940864 ) ) ;
#11245=CARTESIAN_POINT ( 'NONE',  ( -0.5100614604570999910, -79.17313804860999937, -1.204325901401000154 ) ) ;
#11247=CARTESIAN_POINT ( 'NONE',  ( 1.249999999999999778, -78.26041666666665719, 0.1636246173744711763 ) ) ;
#11260=LINE ( 'NONE', #51995, #29604 ) ;
#11265=LINE ( 'NONE', #47292, #42575 ) ;
#11276=CARTESIAN_POINT ( 'NONE',  ( 1.314530797355000225, -78.02943199921000428, -0.9595159925157999981 ) ) ;
#11302=CARTESIAN_POINT ( 'NONE',  ( -0.9813197044111214851, -79.41829332103382910, -1.146063690337610685 ) ) ;
#11309=CARTESIAN_POINT ( 'NONE',  ( -1.249631684896997275, -80.09712312601374151, 0.05486053264030937848 ) ) ;
#11315=CARTESIAN_POINT ( 'NONE',  ( 1.249716928680867145, -78.86070762237109477, 0.1637401775088879741 ) ) ;
#11317=CARTESIAN_POINT ( 'NONE',  ( -0.5178498375169425794, -82.75219414049253430, 1.421764397643496602 ) ) ;
#11318=CARTESIAN_POINT ( 'NONE',  ( -1.250000000000000000, -79.59999999999999432, 0.000000000000000000 ) ) ;
#11338=LINE ( 'NONE', #1908, #23766 ) ;
#11350=CARTESIAN_POINT ( 'NONE',  ( -0.7681833999686477066, -79.92708333333332860, 0.9995835529977223910 ) ) ;
#11352=CARTESIAN_POINT ( 'NONE',  ( -0.8211341099608999716, -80.35493433575999234, -1.491829658087999944 ) ) ;
#11355=CARTESIAN_POINT ( 'NONE',  ( -0.2985019281634834210, -79.85924085546105289, -1.480232390986309321 ) ) ;
#11372=CARTESIAN_POINT ( 'NONE',  ( -0.007261404845503787592, -78.47568757210336798, 1.249841100264606375 ) ) ;
#11396=ORIENTED_EDGE ( 'NONE', *, *, #9775, .F. ) ;
#11406=CARTESIAN_POINT ( 'NONE',  ( 0.5370760595369525880, -82.76026336597686850, -1.130548436120011102 ) ) ;
#11408=DIRECTION ( 'NONE',  ( 0.000000000000000000, 1.000000000000000000, 0.000000000000000000 ) ) ;
#11411=CARTESIAN_POINT ( 'NONE',  ( 1.465732314324990737, -78.97676429292373257, -0.4454333615512816591 ) ) ;
#11416=CARTESIAN_POINT ( 'NONE',  ( -1.250000000000000000, -81.49999999999998579, 0.000000000000000000 ) ) ;
#11429=CARTESIAN_POINT ( 'NONE',  ( -0.5585027192942962904, -83.01198894187744770, 1.119379558410208420 ) ) ;
#11437=VECTOR ( 'NONE', #37382, 1000.000000000000000 ) ;
#11446=EDGE_CURVE ( 'NONE', #38752, #48919, #29647, .T. ) ;
#11453=CARTESIAN_POINT ( 'NONE',  ( 0.3958579896396000608, -81.47369891792999397, -1.618315812554999900 ) ) ;
#11475=CARTESIAN_POINT ( 'NONE',  ( -0.5581268078707392055, -80.51203588205464712, 1.118380629099624546 ) ) ;
#11490=CARTESIAN_POINT ( 'NONE',  ( -1.495765920156680862, -77.83884168506972401, 0.2048668414424503481 ) ) ;
#11500=CARTESIAN_POINT ( 'NONE',  ( 0.6295237254636258939, -78.66666666666665719, -1.092232985442821658 ) ) ;
#11503=CARTESIAN_POINT ( 'NONE',  ( -1.463514287764630550, -80.77019107339425830, -0.3791178640163613833 ) ) ;
#11529=CARTESIAN_POINT ( 'NONE',  ( 0.4168712897526509753, -81.44826334302578630, 1.178261328541365893 ) ) ;
#11537=DIRECTION ( 'NONE',  ( 0.000000000000000000, -0.7071067811866525998, -0.7071067811864425456 ) ) ;
#11550=DIRECTION ( 'NONE',  ( 1.000000000000000000, 0.000000000000000000, 0.000000000000000000 ) ) ;
#11554=CARTESIAN_POINT ( 'NONE',  ( 9.949999999959999286, -86.19999999995999929, 1.488367914068999967E-09 ) ) ;
#11563=CARTESIAN_POINT ( 'NONE',  ( 1.170845731893568331, -81.71777325584498897, -0.5056521153163634485 ) ) ;
#11564=CARTESIAN_POINT ( 'NONE',  ( -0.1732310466989999687, -77.77311942765999220, 1.530487294790999986 ) ) ;
#11570=ORIENTED_EDGE ( 'NONE', *, *, #48227, .T. ) ;
#11572=CARTESIAN_POINT ( 'NONE',  ( -1.456085397364999867, -81.42568918487999952, -0.6271128268704999620 ) ) ;
#11581=CARTESIAN_POINT ( 'NONE',  ( 0.5470778622144214509, -81.26141029258948834, -1.124504696060896425 ) ) ;
#11600=ORIENTED_EDGE ( 'NONE', *, *, #6507, .T. ) ;
#11601=CARTESIAN_POINT ( 'NONE',  ( -0.2126258756077037404, -79.98878773083430360, 1.232946059365898073 ) ) ;
#11609=CARTESIAN_POINT ( 'NONE',  ( -1.036575664049323109, -82.91414466568171804, -1.099456454985895171 ) ) ;
#11611=CARTESIAN_POINT ( 'NONE',  ( 0.004531456056113089548, -79.72569806758036748, -1.249755132514873690 ) ) ;
#11641=CARTESIAN_POINT ( 'NONE',  ( 1.386886761648000066, -79.47070532422000610, -0.9883168548346998872 ) ) ;
#11643=CARTESIAN_POINT ( 'NONE',  ( 0.5323558113646862378, -79.40376574649415886, -1.414199531720756298 ) ) ;
#11659=CARTESIAN_POINT ( 'NONE',  ( 1.242692993603842222, -78.35873442546773049, 0.1364330655704606987 ) ) ;
#11667=CIRCLE ( 'NONE', #9761, 2.299999999999999822 ) ;
#11672=CARTESIAN_POINT ( 'NONE',  ( -0.9331672942107464008, -82.04272704394496429, 0.8318759801249889785 ) ) ;
#11682=CARTESIAN_POINT ( 'NONE',  ( 0.1636246173744642929, -81.86458333333334281, 1.250000000000000888 ) ) ;
#11695=CARTESIAN_POINT ( 'NONE',  ( 0.6122205248558478807, -82.76563067023366216, -1.094235436730285116 ) ) ;
#11699=CARTESIAN_POINT ( 'NONE',  ( -1.124031593430794063, -79.56385312167009261, 0.5524272544800838958 ) ) ;
#11700=CARTESIAN_POINT ( 'NONE',  ( -1.455667963173603141, -78.27095469975617448, -0.3934943062302369565 ) ) ;
#11738=EDGE_CURVE ( 'NONE', #45641, #24608, #4873, .T. ) ;
#11753=CARTESIAN_POINT ( 'NONE',  ( 0.3984351131076449004, -80.44939689437285324, 1.184687104124929613 ) ) ;
#11783=CARTESIAN_POINT ( 'NONE',  ( 0.3915780857578022855, -81.10420615330434657, 1.460265237947602879 ) ) ;
#11792=CARTESIAN_POINT ( 'NONE',  ( -0.7107282322889000303, -81.16095650773000614, -1.148979047684000054 ) ) ;
#11795=CARTESIAN_POINT ( 'NONE',  ( -1.500000000000000000, -83.24999999999998579, 0.000000000000000000 ) ) ;
#11811=CARTESIAN_POINT ( 'NONE',  ( 1.195514927944278050, -81.37427934806251528, 0.3747885264647531356 ) ) ;
#11812=CARTESIAN_POINT ( 'NONE',  ( -0.5432945554243000519, -81.48433123016999957, -1.398152719143000100 ) ) ;
#11831=EDGE_CURVE ( 'NONE', #57912, #44932, #14292, .T. ) ;
#11842=CARTESIAN_POINT ( 'NONE',  ( 0.1636246173744697330, -83.13541666666665719, -1.249999999999999778 ) ) ;
#11845=UNCERTAINTY_MEASURE_WITH_UNIT (LENGTH_MEASURE( 1.000000000000000082E-05 ), #2180, 'distance_accuracy_value', 'NONE');
#11849=CARTESIAN_POINT ( 'NONE',  ( -1.573065832928000063, -78.80897397612000077, 0.4172852021023999991 ) ) ;
#11860=CARTESIAN_POINT ( 'NONE',  ( -1.384313526018999818, -80.98373215275999826, -0.4900246725272000003 ) ) ;
#11864=CARTESIAN_POINT ( 'NONE',  ( 1.496210884224999926, -82.99740586305399859, 0.7325374182646999799 ) ) ;
#11878=CARTESIAN_POINT ( 'NONE',  ( -1.481817198881961950, -79.36475258761093698, -0.2847931209667339814 ) ) ;
#11886=CARTESIAN_POINT ( 'NONE',  ( -1.138858729362214106, -80.06622006278557535, 0.5167690694360175252 ) ) ;
#11893=CARTESIAN_POINT ( 'NONE',  ( -1.274260011682852189, -82.39792736663919470, -0.8801008395726741540 ) ) ;
#11894=CARTESIAN_POINT ( 'NONE',  ( 0.5499219767868982478, -79.76170476781604179, -1.122585114487897773 ) ) ;
#11925=APPLICATION_CONTEXT ( 'automotive_design' ) ;
#11943=CARTESIAN_POINT ( 'NONE',  ( 0.4506131419724269116, -78.44581188727093490, 1.166324524794932982 ) ) ;
#11948=FACE_OUTER_BOUND ( 'NONE', #39406, .T. ) ;
#11955=CARTESIAN_POINT ( 'NONE',  ( 0.4123449529901261346, -81.94846309541368612, 1.180275517497846316 ) ) ;
#11967=CARTESIAN_POINT ( 'NONE',  ( -0.6292628992211932726, -78.18342697397770280, -1.092251993020334044 ) ) ;
#11980=CARTESIAN_POINT ( 'NONE',  ( 0.3746329102212312967, -82.74941308002549079, -1.192428859071045899 ) ) ;
#11985=CARTESIAN_POINT ( 'NONE',  ( 0.8142187701153039692, -79.41871938336271342, 0.9486283461955962171 ) ) ;
#11986=CARTESIAN_POINT ( 'NONE',  ( -1.133755312681792971, -78.69107945759728295, 1.029799983678180819 ) ) ;
#12040=CARTESIAN_POINT ( 'NONE',  ( 0.5488453404877545738, -80.43885426786198423, 1.123841912394225817 ) ) ;
#12053=CARTESIAN_POINT ( 'NONE',  ( -1.105309719138173108, -77.91022932963348069, -1.053953978756914101 ) ) ;
#12060=CARTESIAN_POINT ( 'NONE',  ( 0.7681833999686413783, -83.32291666666667140, 0.9995835529977274980 ) ) ;
#12066=CARTESIAN_POINT ( 'NONE',  ( 0.7537979459027094320, -80.41593265530910628, -1.352198804742777760 ) ) ;
#12076=CARTESIAN_POINT ( 'NONE',  ( 0.6445170026176001432, -81.98218377781998356, 1.319487011787000119 ) ) ;
#12095=CARTESIAN_POINT ( 'NONE',  ( -0.3164372427141999844, -79.71981609832999993, 1.635583079321000000 ) ) ;
#12101=CARTESIAN_POINT ( 'NONE',  ( -0.3271848554491046945, -78.39583333333328596, 1.217465845835393301 ) ) ;
#12107=CARTESIAN_POINT ( 'NONE',  ( 0.8706374436944001038, -77.82080235332999507, -1.123568498160000040 ) ) ;
#12123=CARTESIAN_POINT ( 'NONE',  ( -0.7681833999686432657, -83.07291666666667140, -0.9995835529977258327 ) ) ;
#12128=CARTESIAN_POINT ( 'NONE',  ( 1.250000000000000000, -81.74999999999998579, 0.000000000000000000 ) ) ;
#12130=DIRECTION ( 'NONE',  ( 0.000000000000000000, 1.000000000000000000, 0.000000000000000000 ) ) ;
#12138=CARTESIAN_POINT ( 'NONE',  ( -1.512180334517000180, -83.36904964980398347, 0.4761993468540999808 ) ) ;
#12139=CARTESIAN_POINT ( 'NONE',  ( -1.348464306027999937, -81.48900587363999648, -0.5807621341562000383 ) ) ;
#12142=CARTESIAN_POINT ( 'NONE',  ( 1.250000000000000000, -81.34999999999999432, 0.000000000000000000 ) ) ;
#12143=CARTESIAN_POINT ( 'NONE',  ( 0.3958579896396000608, -81.35526627018998624, -1.618315812554999900 ) ) ;
#12148=CARTESIAN_POINT ( 'NONE',  ( 0.4436071767293376378, -81.25405316505460007, -1.168520871849203946 ) ) ;
#12157=CARTESIAN_POINT ( 'NONE',  ( -1.458706046781999888, -81.78949499347999108, 0.8046341008317999810 ) ) ;
#12174=CARTESIAN_POINT ( 'NONE',  ( -0.5534603023178866765, -82.94451038915471486, -1.408692892589827217 ) ) ;
#12175=CARTESIAN_POINT ( 'NONE',  ( 0.4887196984038748582, -79.75730190472970094, -1.150295180735885658 ) ) ;
#12189=ORIENTED_EDGE ( 'NONE', *, *, #50366, .F. ) ;
#12195=ORIENTED_EDGE ( 'NONE', *, *, #39281, .T. ) ;
#12208=VERTEX_POINT ( 'NONE', #28963 ) ;
#12226=DIRECTION ( 'NONE',  ( 0.000000000000000000, 1.000000000000000000, 0.000000000000000000 ) ) ;
#12238=CARTESIAN_POINT ( 'NONE',  ( 0.3833199769307082949, -81.95046860891231688, 1.189846988800133287 ) ) ;
#12239=CARTESIAN_POINT ( 'NONE',  ( 1.178978867320999990, -78.64234607169998981, 1.173689911365999983 ) ) ;
#12244=CYLINDRICAL_SURFACE ( 'NONE', #25869, 1.250000000000000000 ) ;
#12250=CARTESIAN_POINT ( 'NONE',  ( -0.9465222407332000154, -81.15663953506998496, -0.8164530897714000757 ) ) ;
#12339=CIRCLE ( 'NONE', #3870, 2.899999999999999911 ) ;
#12348=CARTESIAN_POINT ( 'NONE',  ( -0.1636246173744673738, -78.61458333333330017, -1.249999999999999778 ) ) ;
#12349=CARTESIAN_POINT ( 'NONE',  ( -0.7972742194625092038, -80.33495930260389173, -1.448481206412859157 ) ) ;
#12358=CARTESIAN_POINT ( 'NONE',  ( -1.407332420019999919, -81.66638770227000066, -0.4193609517060999936 ) ) ;
#12378=CARTESIAN_POINT ( 'NONE',  ( 0.9441861370063999725, -79.59744055935000517, 1.372505234203999835 ) ) ;
#12387=CARTESIAN_POINT ( 'NONE',  ( 1.092232985442820992, -78.29166666666667140, 0.6295237254636267821 ) ) ;
#12393=CARTESIAN_POINT ( 'NONE',  ( 1.305753739922999923, -77.92566549289000477, 0.5616213463899000224 ) ) ;
#12406=COLOUR_RGB ( '', 0.72549020, 0.75294118, 0.79215686) ;
#12411=CARTESIAN_POINT ( 'NONE',  ( -0.9995835529977249445, -83.05208333333330017, -0.7681833999686439318 ) ) ;
#12418=CARTESIAN_POINT ( 'NONE',  ( 0.000000000000000000, -80.69999999999998863, 0.000000000000000000 ) ) ;
#12423=CARTESIAN_POINT ( 'NONE',  ( -0.8973488778757167106, -83.03941064879536782, 0.8696509586403449177 ) ) ;
#12426=CARTESIAN_POINT ( 'NONE',  ( 1.565347158977999920, -82.54782237971299708, -0.6704515100525999527 ) ) ;
#12427=CARTESIAN_POINT ( 'NONE',  ( 1.399788002916999785, -80.73109529231999204, 0.4438937798904999954 ) ) ;
#12432=CARTESIAN_POINT ( 'NONE',  ( 1.571434226476000173, -82.93424664794399348, -0.5530452149683998675 ) ) ;
#12438=EDGE_LOOP ( 'NONE', ( #39330, #32679, #8462, #22484 ) ) ;
#12453=DIRECTION ( 'NONE',  ( 0.000000000000000000, -1.000000000000000000, 4.329869796038000067E-14 ) ) ;
#12455=CARTESIAN_POINT ( 'NONE',  ( 1.365918550425730738, -82.06390440843598810, -0.6514700801450835632 ) ) ;
#12466=ORIENTED_EDGE ( 'NONE', *, *, #19715, .T. ) ;
#12476=ORIENTED_EDGE ( 'NONE', *, *, #13739, .T. ) ;
#12522=CARTESIAN_POINT ( 'NONE',  ( 1.081160367018396462, -81.89214477630333988, 0.6272441749643766773 ) ) ;
#12530=AXIS2_PLACEMENT_3D ( 'NONE', #23484, #794, #27900 ) ;
#12599=VECTOR ( 'NONE', #24874, 1000.000000000000000 ) ;
#12606=B_SPLINE_CURVE_WITH_KNOTS ( 'NONE', 3,
 ( #30421, #48453, #25993, #12991, #44017, #39861 ),
 .UNSPECIFIED., .F., .F.,
 ( 4, 2, 4 ),
 ( 0.000000000000000000, 0.5000000000000000000, 1.000000000000000000 ),
 .UNSPECIFIED. ) ;
#12621=CARTESIAN_POINT ( 'NONE',  ( -1.158060974166144508, -77.79422440721735654, 0.9671104533053733743 ) ) ;
#12627=CARTESIAN_POINT ( 'NONE',  ( -0.9995835529977281642, -83.44791666666662877, 0.7681833999686391579 ) ) ;
#12637=CARTESIAN_POINT ( 'NONE',  ( 0.9655213319334129407, -80.02944677308721566, -1.162632870702606791 ) ) ;
#12645=CARTESIAN_POINT ( 'NONE',  ( -0.5793938177159999592, -82.55061671381200483, 1.349352049262000142 ) ) ;
#12647=ORIENTED_EDGE ( 'NONE', *, *, #13563, .F. ) ;
#12658=CARTESIAN_POINT ( 'NONE',  ( 0.000000000000000000, -77.74999999981000087, 0.000000000000000000 ) ) ;
#12675=VERTEX_POINT ( 'NONE', #46791 ) ;
#12677=CARTESIAN_POINT ( 'NONE',  ( -0.2201363562291999698, -79.36327907013999550, -1.483758735329000045 ) ) ;
#12678=CARTESIAN_POINT ( 'NONE',  ( 0.3645270829314000149, -79.35220299592999993, -1.380445500850000062 ) ) ;
#12679=EDGE_LOOP ( 'NONE', ( #25171, #48980, #39361, #42980, #22567, #41808, #41449, #10273, #9926, #11180, #48692, #48819 ) ) ;
#12682=CARTESIAN_POINT ( 'NONE',  ( 0.9951994886139982066, -80.29861577946837770, -0.7569065563915547967 ) ) ;
#12702=CARTESIAN_POINT ( 'NONE',  ( -1.249764222956683657, -83.09108160190875481, 0.1462821142628205062 ) ) ;
#12707=CARTESIAN_POINT ( 'NONE',  ( 0.4426188121580000301, -82.10602282125999807, -1.400191678299000042 ) ) ;
#12709=CARTESIAN_POINT ( 'NONE',  ( 1.426111243542000029, -80.22582157143999382, 0.3502211593775000353 ) ) ;
#12713=CARTESIAN_POINT ( 'NONE',  ( -0.5544740949720999845, -82.11317685150999068, 1.570928860995999932 ) ) ;
#12725=CARTESIAN_POINT ( 'NONE',  ( -0.4492251327744000156, -81.66711945450001053, 1.604198796042999753 ) ) ;
#12733=CARTESIAN_POINT ( 'NONE',  ( 0.4768038028798605721, -79.94409901709930466, 1.155327188750691292 ) ) ;
#12767=CARTESIAN_POINT ( 'NONE',  ( 0.1198033158700999995, -79.08031231683999351, 1.623056241665000066 ) ) ;
#12786=VERTEX_POINT ( 'NONE', #2629 ) ;
#12803=CARTESIAN_POINT ( 'NONE',  ( 1.007676913700946697, -81.90086700953483501, 0.7397467089371103643 ) ) ;
#12804=CARTESIAN_POINT ( 'NONE',  ( -1.410540931501999884, -78.42725491157000306, -0.6403706075564999933 ) ) ;
#12806=CARTESIAN_POINT ( 'NONE',  ( -0.7280429309147493644, -82.83501156738459770, -1.324360742052439477 ) ) ;
#12813=CARTESIAN_POINT ( 'NONE',  ( 1.041624132644355161, -81.80353841734945775, -0.6908730350728758962 ) ) ;
#12831=ORIENTED_EDGE ( 'NONE', *, *, #6505, .F. ) ;
#12833=CARTESIAN_POINT ( 'NONE',  ( -1.498805164377271737, -77.75840249518691394, -0.1584492094687433572 ) ) ;
#12853=DIRECTION ( 'NONE',  ( 1.000000000000000000, 0.000000000000000000, 0.000000000000000000 ) ) ;
#12886=ORIENTED_EDGE ( 'NONE', *, *, #26417, .T. ) ;
#12916=CARTESIAN_POINT ( 'NONE',  ( 1.227268718659146218, -80.04969058873581389, -0.8848763678067933514 ) ) ;
#12924=CARTESIAN_POINT ( 'NONE',  ( 1.261625697157999992, -81.35059162671998934, -0.7514603626543999715 ) ) ;
#12936=VERTEX_POINT ( 'NONE', #17638 ) ;
#12947=FACE_OUTER_BOUND ( 'NONE', #45972, .T. ) ;
#12954=VECTOR ( 'NONE', #30740, 1000.000000000000000 ) ;
#12955=VERTEX_POINT ( 'NONE', #51076 ) ;
#12958=CARTESIAN_POINT ( 'NONE',  ( 0.8068013270406000359, -79.03761357724998504, 1.305699365831000103 ) ) ;
#12961=CARTESIAN_POINT ( 'NONE',  ( -0.3767128267918133933, -79.35487657498305225, -1.459930215568542522 ) ) ;
#12962=CARTESIAN_POINT ( 'NONE',  ( 0.0006957917016094362049, -80.22560324140505372, -1.249665624490517768 ) ) ;
#12983=CARTESIAN_POINT ( 'NONE',  ( -0.8902956382338467201, -83.03876140007196227, 0.8768580129426997161 ) ) ;
#12989=CARTESIAN_POINT ( 'NONE',  ( -0.3959877895327999497, -81.85338596081999185, 1.414086365320999850 ) ) ;
#12990=CARTESIAN_POINT ( 'NONE',  ( 1.249711497515000103, -80.16266235632998871, -0.7711480544179000196 ) ) ;
#12991=CARTESIAN_POINT ( 'NONE',  ( -0.9768374075688754932, -77.83333333333224857, 1.065675943311487295 ) ) ;
#13014=CARTESIAN_POINT ( 'NONE',  ( 0.2973127429259597720, -79.95643973076548150, 1.214524578331088733 ) ) ;
#13022=CARTESIAN_POINT ( 'NONE',  ( 2.899999999999999911, -80.69999999999998863, 0.000000000000000000 ) ) ;
#13041=CARTESIAN_POINT ( 'NONE',  ( 1.065724622738618121, -79.39441019242424602, 0.6536201573516686736 ) ) ;
#13084=CARTESIAN_POINT ( 'NONE',  ( 0.000000000000000000, -77.59999999938000315, 0.000000000000000000 ) ) ;
#13089=CARTESIAN_POINT ( 'NONE',  ( 0.5348319831205907704, -81.93981601381945268, 1.130533534708823229 ) ) ;
#13090=CARTESIAN_POINT ( 'NONE',  ( -1.491498510839000202, -78.37157334178999690, 0.4184882615579000320 ) ) ;
#13092=CARTESIAN_POINT ( 'NONE',  ( 1.509093300816331418, -82.99695827279550997, -0.05655753630307266966 ) ) ;
#13098=CARTESIAN_POINT ( 'NONE',  ( 1.140339328391035467, -81.81637019837238256, -0.5133320548427554586 ) ) ;
#13101=CARTESIAN_POINT ( 'NONE',  ( -0.3271848554490991434, -80.10416666666667140, -1.217465845835395299 ) ) ;
#13107=EDGE_LOOP ( 'NONE', ( #57482, #47424, #29167, #2198 ) ) ;
#13108=VERTEX_POINT ( 'NONE', #47426 ) ;
#13207=CARTESIAN_POINT ( 'NONE',  ( -1.057528278039415515, -80.41407927041096571, -1.131349316642257019 ) ) ;
#13218=CARTESIAN_POINT ( 'NONE',  ( 1.575652246471999973, -82.55093166112899894, 0.6458614041720999177 ) ) ;
#13255=CARTESIAN_POINT ( 'NONE',  ( 1.574466862065000194, -78.99606712646000517, -0.4877912776778999815 ) ) ;
#13260=CARTESIAN_POINT ( 'NONE',  ( 0.4850963087208033375, -80.25687247894693144, -1.151929813589695373 ) ) ;
#13269=ORIENTED_EDGE ( 'NONE', *, *, #22775, .T. ) ;
#13274=CARTESIAN_POINT ( 'NONE',  ( -1.250000000000000000, -81.49999999999998579, 0.000000000000000000 ) ) ;
#13275=CARTESIAN_POINT ( 'NONE',  ( 0.000000000000000000, -77.50000000000000000, 0.000000000000000000 ) ) ;
#13280=FACE_OUTER_BOUND ( 'NONE', #9511, .T. ) ;
#13285=CARTESIAN_POINT ( 'NONE',  ( -1.446479059201000172, -82.92693514403299559, -0.6496884318727998986 ) ) ;
#13286=CARTESIAN_POINT ( 'NONE',  ( 1.250000000000000000, -78.85000000000000853, 0.000000000000000000 ) ) ;
#13302=VECTOR ( 'NONE', #55991, 1000.000000000000000 ) ;
#13310=CARTESIAN_POINT ( 'NONE',  ( 0.4375120388952565831, -79.94686972374893230, 1.170817719393832279 ) ) ;
#13332=CARTESIAN_POINT ( 'NONE',  ( -0.3278092779548479330, -82.49649409683389933, 1.218271132180950511 ) ) ;
#13339=CIRCLE ( 'NONE', #33024, 10.14999999999999858 ) ;
#13349=CARTESIAN_POINT ( 'NONE',  ( -0.9995835529977249445, -78.05208333333330017, -0.7681833999686439318 ) ) ;
#13353=EDGE_CURVE ( 'NONE', #10113, #21051, #44716, .T. ) ;
#13384=CARTESIAN_POINT ( 'NONE',  ( 1.002166123569000034, -79.27011357725000096, 1.026519443915999918 ) ) ;
#13396=LINE ( 'NONE', #57987, #47907 ) ;
#13423=CARTESIAN_POINT ( 'NONE',  ( 0.5308835263170998964, -80.92289485077999700, 1.242631599581000001 ) ) ;
#13476=EDGE_CURVE ( 'NONE', #21051, #28446, #49919, .T. ) ;
#13478=CARTESIAN_POINT ( 'NONE',  ( -1.500000000000000000, -83.34999999999999432, 0.000000000000000000 ) ) ;
#13507=CARTESIAN_POINT ( 'NONE',  ( -1.404188869873914003, -80.81895558338473506, 0.5634542928392101135 ) ) ;
#13508=CARTESIAN_POINT ( 'NONE',  ( -1.163246785803522698, -78.56960608111629085, 0.4728783135193991849 ) ) ;
#13517=CARTESIAN_POINT ( 'NONE',  ( -0.8956573524961000121, -81.35090657403999614, -1.447939571232000011 ) ) ;
#13535=EDGE_CURVE ( 'NONE', #15743, #20349, #42336, .T. ) ;
#13540=CARTESIAN_POINT ( 'NONE',  ( -0.8033051684372000123, -80.47378378841000313, -1.459438184619000101 ) ) ;
#13554=CARTESIAN_POINT ( 'NONE',  ( 1.486116868684999925, -77.93655061187999422, -0.3837144090195000468 ) ) ;
#13557=CARTESIAN_POINT ( 'NONE',  ( 0.9273595869657466073, -80.29200840023126773, -0.8380822826822911242 ) ) ;
#13563=EDGE_CURVE ( 'NONE', #15817, #54320, #40553, .T. ) ;
#13580=CARTESIAN_POINT ( 'NONE',  ( 1.503815466746999840, -82.16902456270999267, 0.5029271919957000181 ) ) ;
#13581=CARTESIAN_POINT ( 'NONE',  ( -1.250000000000000000, -82.59999999999999432, 0.000000000000000000 ) ) ;
#13584=CARTESIAN_POINT ( 'NONE',  ( 1.250000000000000000, -81.74999999999998579, 0.000000000000000000 ) ) ;
#13604=DIRECTION ( 'NONE',  ( -0.7071067811865969777, -0.7071067811864980568, 1.359270614438996183E-10 ) ) ;
#13605=DIRECTION ( 'NONE',  ( 0.000000000000000000, -1.000000000000000000, 0.000000000000000000 ) ) ;
#13609=CARTESIAN_POINT ( 'NONE',  ( -0.6943029181025289764, -81.52241017303003900, 1.039652336598162696 ) ) ;
#13618=ORIENTED_EDGE ( 'NONE', *, *, #49087, .F. ) ;
#13626=EDGE_CURVE ( 'NONE', #48919, #26401, #30885, .T. ) ;
#13634=AXIS2_PLACEMENT_3D ( 'NONE', #22824, #31956, #716 ) ;
#13644=CARTESIAN_POINT ( 'NONE',  ( 0.1660104325307999729, -78.07804406081000081, 1.618982269915999916 ) ) ;
#13679=CARTESIAN_POINT ( 'NONE',  ( 0.5818457612699999837, -80.86456775278999487, -1.560998038830999857 ) ) ;
#13680=CARTESIAN_POINT ( 'NONE',  ( -0.8239329289818000390, -78.88034258879000049, 1.174399563024999926 ) ) ;
#13681=CIRCLE ( 'NONE', #46720, 10.14999999999999858 ) ;
#13683=CARTESIAN_POINT ( 'NONE',  ( 1.250300346049109557, -83.04756661823621755, 0.8499747096666684376 ) ) ;
#13695=ORIENTED_EDGE ( 'NONE', *, *, #53545, .T. ) ;
#13699=ORIENTED_EDGE ( 'NONE', *, *, #32827, .F. ) ;
#13702=CARTESIAN_POINT ( 'NONE',  ( 1.132506419232103712, -80.38497993291565535, 0.5291395119344256548 ) ) ;
#13712=VERTEX_POINT ( 'NONE', #13757 ) ;
#13732=CARTESIAN_POINT ( 'NONE',  ( -1.217465845835394411, -79.02083333333330017, -0.3271848554491003647 ) ) ;
#13739=EDGE_CURVE ( 'NONE', #20818, #48919, #41469, .T. ) ;
#13755=EDGE_LOOP ( 'NONE', ( #9999, #12189, #47633, #42178, #18898 ) ) ;
#13757=CARTESIAN_POINT ( 'NONE',  ( 0.000000000000000000, -86.39999999999999147, -10.14999999999897007 ) ) ;
#13761=ADVANCED_FACE ( 'NONE', ( #8755 ), #53629, .T. ) ;
#13796=CARTESIAN_POINT ( 'NONE',  ( -0.9995835529977281642, -80.94791666666662877, 0.7681833999686391579 ) ) ;
#13798=CARTESIAN_POINT ( 'NONE',  ( -1.317248530341201818, -80.39383545476231063, -0.8131718307597066708 ) ) ;
#13809=CARTESIAN_POINT ( 'NONE',  ( -1.354012292646000093, -83.30884224245099290, -0.7194680089321999761 ) ) ;
#13848=CARTESIAN_POINT ( 'NONE',  ( -1.008674225483999987, -77.84257259131000239, -1.303690889073000125 ) ) ;
#13850=VERTEX_POINT ( 'NONE', #13984 ) ;
#13853=CARTESIAN_POINT ( 'NONE',  ( 0.4786272935714176446, -80.25641286416187370, -1.154639604756080073 ) ) ;
#13855=VECTOR ( 'NONE', #26236, 1000.000000000000000 ) ;
#13876=CARTESIAN_POINT ( 'NONE',  ( -1.368292558779000023, -82.92709261769098816, 0.5331262435804999811 ) ) ;
#13881=CARTESIAN_POINT ( 'NONE',  ( 1.496210884224999926, -83.05662218692300769, 0.7325374182646999799 ) ) ;
#13889=EDGE_CURVE ( 'NONE', #36858, #13850, #23171, .T. ) ;
#13906=DIRECTION ( 'NONE',  ( 0.000000000000000000, -1.000000000000000000, 0.000000000000000000 ) ) ;
#13923=CARTESIAN_POINT ( 'NONE',  ( -0.9994182591520053283, -82.54857722637443374, 0.7676657006752972690 ) ) ;
#13937=CARTESIAN_POINT ( 'NONE',  ( -0.7213013439201000354, -77.79963621190999845, -1.458901041394999876 ) ) ;
#13943=ORIENTED_EDGE ( 'NONE', *, *, #38015, .T. ) ;
#13957=ORIENTED_EDGE ( 'NONE', *, *, #34070, .F. ) ;
#13975=FACE_OUTER_BOUND ( 'NONE', #53203, .T. ) ;
#13976=CARTESIAN_POINT ( 'NONE',  ( 1.276747624218999899, -79.09543374892000145, -0.8772774337639999143 ) ) ;
#13978=CARTESIAN_POINT ( 'NONE',  ( 0.5734623601598806131, -82.90586325100210274, -1.399525524612139638 ) ) ;
#13984=CARTESIAN_POINT ( 'NONE',  ( -1.250000000000000000, -81.59999999999999432, 0.000000000000000000 ) ) ;
#13991=ORIENTED_EDGE ( 'NONE', *, *, #37762, .F. ) ;
#13993=CARTESIAN_POINT ( 'NONE',  ( 1.157571443481175466, -80.38088009010486701, 0.4716244123812511901 ) ) ;
#14012=CARTESIAN_POINT ( 'NONE',  ( -0.7850755733694999572, -79.21775351646000729, -1.063938263677999929 ) ) ;
#14025=CARTESIAN_POINT ( 'NONE',  ( 1.250000000000000000, -79.25000000000000000, 0.000000000000000000 ) ) ;
#14026=ORIENTED_EDGE ( 'NONE', *, *, #25276, .F. ) ;
#14059=ORIENTED_EDGE ( 'NONE', *, *, #50912, .F. ) ;
#14068=ORIENTED_EDGE ( 'NONE', *, *, #49087, .T. ) ;
#14069=CARTESIAN_POINT ( 'NONE',  ( 0.9403724367845377463, -82.79329554165276761, -0.8236006839109907274 ) ) ;
#14096=CARTESIAN_POINT ( 'NONE',  ( 0.7681833999686413783, -80.82291666666668561, 0.9995835529977274980 ) ) ;
#14103=CARTESIAN_POINT ( 'NONE',  ( 0.6295237254636258939, -80.66666666666665719, -1.092232985442821658 ) ) ;
#14107=CARTESIAN_POINT ( 'NONE',  ( -1.519651782304000109, -81.72970439103998785, -0.4528301974880000191 ) ) ;
#14115=DIRECTION ( 'NONE',  ( 0.000000000000000000, -1.000000000000000000, 0.000000000000000000 ) ) ;
#14137=CARTESIAN_POINT ( 'NONE',  ( -0.5697605620548999994, -78.36688828910999405, -1.546692981914000065 ) ) ;
#14141=CARTESIAN_POINT ( 'NONE',  ( -0.8629689471358689135, -80.16484394472540487, -0.9039662746332275400 ) ) ;
#14162=CARTESIAN_POINT ( 'NONE',  ( 0.3210957952920999725, -81.66406578914998704, -1.312678830453999801 ) ) ;
#14164=CARTESIAN_POINT ( 'NONE',  ( 0.2122939316688999822, -79.65754610911000100, -1.334248387208000208 ) ) ;
#14168=CARTESIAN_POINT ( 'NONE',  ( -0.5790013745696001024, -82.86714454159299237, -1.562055304842999925 ) ) ;
#14190=CARTESIAN_POINT ( 'NONE',  ( -1.164165648490407268, -81.57056345355888993, 0.4549354940310009754 ) ) ;
#14217=VERTEX_POINT ( 'NONE', #51407 ) ;
#14224=CARTESIAN_POINT ( 'NONE',  ( 1.621809933883000099, -78.46781504927000128, 0.1356303529659999840 ) ) ;
#14237=CIRCLE ( 'NONE', #1048, 9.500000000000000000 ) ;
#14261=CARTESIAN_POINT ( 'NONE',  ( -0.8033051684372000123, -80.35535114066999540, -1.459438184619000101 ) ) ;
#14262=CARTESIAN_POINT ( 'NONE',  ( 0.1346575116716999809, -78.38684357976998740, 1.313219419913000063 ) ) ;
#14264=CARTESIAN_POINT ( 'NONE',  ( 1.501921250453331025, -81.50907291683472522, 0.1730332911310038246 ) ) ;
#14265=CARTESIAN_POINT ( 'NONE',  ( 1.010008291100382483, -83.16719236129050330, 1.155447337432020438 ) ) ;
#14269=ORIENTED_EDGE ( 'NONE', *, *, #22210, .T. ) ;
#14270=CARTESIAN_POINT ( 'NONE',  ( -0.9597372295412756049, -81.65614046397973880, -0.8042208309310099335 ) ) ;
#14272=SURFACE_STYLE_FILL_AREA ( #11040 ) ;
#14282=CARTESIAN_POINT ( 'NONE',  ( 1.048462055999483722, -80.39633018666535236, 0.6817341454441373516 ) ) ;
#14288=FACE_OUTER_BOUND ( 'NONE', #55749, .T. ) ;
#14292=LINE ( 'NONE', #18162, #25369 ) ;
#14299=CARTESIAN_POINT ( 'NONE',  ( 0.7503380909894999951, -79.97566409777999752, 1.262315685543000221 ) ) ;
#14332=CARTESIAN_POINT ( 'NONE',  ( 0.7681833999686413783, -82.32291666666665719, 0.9995835529977274980 ) ) ;
#14333=CARTESIAN_POINT ( 'NONE',  ( 0.9995835529977264988, -82.69791666666664298, -0.7681833999686417114 ) ) ;
#14342=CARTESIAN_POINT ( 'NONE',  ( 0.000000000000000000, -77.50000000000000000, -2.299999999999999822 ) ) ;
#14364=EDGE_CURVE ( 'NONE', #44478, #26509, #9792, .T. ) ;
#14375=CARTESIAN_POINT ( 'NONE',  ( -1.192783596312423589, -83.07577989394255269, 0.3769634839055466813 ) ) ;
#14387=CARTESIAN_POINT ( 'NONE',  ( -0.1636246173744673738, -80.61458333333328596, -1.249999999999999778 ) ) ;
#14431=CARTESIAN_POINT ( 'NONE',  ( -0.7033595694237251283, -80.17773795642190748, -1.034965556745985893 ) ) ;
#14432=CARTESIAN_POINT ( 'NONE',  ( 0.8544064497059326024, -77.86067708349810346, -1.110392862171576622 ) ) ;
#14436=CARTESIAN_POINT ( 'NONE',  ( 0.2063409356571887232, -78.21362681902969882, 1.524325540200904827 ) ) ;
#14444=DIRECTION ( 'NONE',  ( 0.000000000000000000, 1.000000000000000000, 0.000000000000000000 ) ) ;
#14456=CARTESIAN_POINT ( 'NONE',  ( -1.479613214588597625, -81.26615285871807259, -0.3067698822034324313 ) ) ;
#14457=CARTESIAN_POINT ( 'NONE',  ( 1.249910393070341685, -78.83987707960370983, -0.1637800131244415147 ) ) ;
#14468=CONICAL_SURFACE ( 'NONE', #41827, 1.500000000188000060, 0.7853981633972997312 ) ;
#14517=CARTESIAN_POINT ( 'NONE',  ( -1.491326706514000122, -77.80317096599999616, -0.6515838025032999470 ) ) ;
#14555=CARTESIAN_POINT ( 'NONE',  ( 1.617840321509000034, -79.98033874124999443, 0.3973055507782000118 ) ) ;
#14556=CARTESIAN_POINT ( 'NONE',  ( -0.1405144323591999977, -77.90426997500999562, 1.241437707376999988 ) ) ;
#14558=CARTESIAN_POINT ( 'NONE',  ( -1.118453976065381994, -81.69126296042138335, 1.015803637914979740 ) ) ;
#14561=CARTESIAN_POINT ( 'NONE',  ( 1.194177587799142071, -79.82664734801842599, -0.3688301857723336186 ) ) ;
#14563=CARTESIAN_POINT ( 'NONE',  ( -0.8771444964703341007, -81.66363988412527419, -0.8900962782329024936 ) ) ;
#14564=DIRECTION ( 'NONE',  ( 1.000000000000000000, 0.000000000000000000, 0.000000000000000000 ) ) ;
#14581=EDGE_CURVE ( 'NONE', #36091, #19028, #45672, .T. ) ;
#14593=CARTESIAN_POINT ( 'NONE',  ( -0.6709475781581999421, -80.79689136786998915, -1.436741477991000160 ) ) ;
#14630=DIRECTION ( 'NONE',  ( 0.000000000000000000, -1.000000000000000000, 0.000000000000000000 ) ) ;
#14640=VERTEX_POINT ( 'NONE', #176 ) ;
#14644=ORIENTED_EDGE ( 'NONE', *, *, #28325, .T. ) ;
#14647=CARTESIAN_POINT ( 'NONE',  ( -1.250000000000000000, -79.59999999999999432, 0.000000000000000000 ) ) ;
#14665=CARTESIAN_POINT ( 'NONE',  ( 0.9973843665736694675, -82.90183089828425977, 0.7531913344093712492 ) ) ;
#14672=CARTESIAN_POINT ( 'NONE',  ( 0.5372315382144975393, -79.69542381488500382, 1.412885547448977652 ) ) ;
#14709=CARTESIAN_POINT ( 'NONE',  ( -0.9751240804252407912, -80.54658200636069409, 0.7826983233412607710 ) ) ;
#14724=CARTESIAN_POINT ( 'NONE',  ( -1.030512144556630316, -79.28444148747665565, 1.103585378104965375 ) ) ;
#14741=CARTESIAN_POINT ( 'NONE',  ( 1.213634779058999857, -83.30620538201100089, 0.5941895605367999433 ) ) ;
#14775=CARTESIAN_POINT ( 'NONE',  ( -1.239721164836000256, -79.18402316759998882, -0.6954227484140999005 ) ) ;
#14806=CARTESIAN_POINT ( 'NONE',  ( 1.169626569868999821, -78.08157881489999852, 1.131652196797999999 ) ) ;
#14812=ORIENTED_EDGE ( 'NONE', *, *, #11235, .T. ) ;
#14814=CARTESIAN_POINT ( 'NONE',  ( 1.476447168807000221, -81.17305232442998886, 0.5783644924166000401 ) ) ;
#14845=CARTESIAN_POINT ( 'NONE',  ( 1.417725061834000044, -80.03561217387999704, -0.8748226493128999914 ) ) ;
#14846=CARTESIAN_POINT ( 'NONE',  ( -1.381259992031000028, -78.43489003055999831, 0.3875572711764000422 ) ) ;
#14848=CARTESIAN_POINT ( 'NONE',  ( -0.5205927694291033747, -81.34712621142415401, -1.418571885323605786 ) ) ;
#14852=CARTESIAN_POINT ( 'NONE',  ( -0.9057099665792408549, -81.03819025148258959, 0.9057972107843319520 ) ) ;
#14854=CARTESIAN_POINT ( 'NONE',  ( -0.4933197585330857393, -81.69281355437695424, -1.148584473005615170 ) ) ;
#14863=CARTESIAN_POINT ( 'NONE',  ( -1.172866835075395020, -77.78255208343296090, -0.9024179113435036870 ) ) ;
#14883=CARTESIAN_POINT ( 'NONE',  ( 1.298035947816999824, -80.35461938843998553, -0.6866955795318000488 ) ) ;
#14886=CARTESIAN_POINT ( 'NONE',  ( 0.7090065431140329943, -79.41388741558243680, -1.333103239968771447 ) ) ;
#14895=CARTESIAN_POINT ( 'NONE',  ( 1.250000000000000222, -79.23958333333331439, -0.1636246173744659582 ) ) ;
#14898=FACE_OUTER_BOUND ( 'NONE', #32639, .T. ) ;
#14937=CARTESIAN_POINT ( 'NONE',  ( 1.092468167825580094, -82.80859976460473604, -0.6286521223243165535 ) ) ;
#14941=CARTESIAN_POINT ( 'NONE',  ( -0.8122579684721802362, -79.32966908951244989, -1.270466924700469180 ) ) ;
#14943=ADVANCED_FACE ( 'NONE', ( #38001 ), #10277, .F. ) ;
#14946=CIRCLE ( 'NONE', #57347, 2.500000000000000000 ) ;
#14962=CARTESIAN_POINT ( 'NONE',  ( 1.142427346679885547, -82.88327974481559579, 0.5074387660638589592 ) ) ;
#14966=CARTESIAN_POINT ( 'NONE',  ( -0.8579432262127338893, -78.03348889011373046, 0.9468520969737713733 ) ) ;
#14969=FACE_OUTER_BOUND ( 'NONE', #48621, .T. ) ;
#14970=CARTESIAN_POINT ( 'NONE',  ( 1.021972327705173322, -79.53347328969611851, -1.113959016257049628 ) ) ;
#14983=CYLINDRICAL_SURFACE ( 'NONE', #24805, 1.250000000000000000 ) ;
#14986=CARTESIAN_POINT ( 'NONE',  ( 0.5269479332349999989, -83.23821404977199734, 1.580352090963000000 ) ) ;
#14999=CARTESIAN_POINT ( 'NONE',  ( -0.7889670424319170650, -80.67174664738183765, -0.9893556795060300946 ) ) ;
#15005=EDGE_LOOP ( 'NONE', ( #23513, #12195, #33660, #7291 ) ) ;
#15008=CARTESIAN_POINT ( 'NONE',  ( -1.250000000000000000, -80.59999999999999432, 0.000000000000000000 ) ) ;
#15019=CARTESIAN_POINT ( 'NONE',  ( -1.168247351827577551, -80.12911975281166121, -0.4458151081181576658 ) ) ;
#15024=CARTESIAN_POINT ( 'NONE',  ( 1.504596964206185161, -78.10654535218401406, 0.1305286778095537392 ) ) ;
#15041=CARTESIAN_POINT ( 'NONE',  ( -1.441964492907930273, -81.22566618236561453, 0.4560415640900693512 ) ) ;
#15045=CARTESIAN_POINT ( 'NONE',  ( 1.217465845835393967, -78.77083333333330017, 0.3271848554491025851 ) ) ;
#15072=CARTESIAN_POINT ( 'NONE',  ( 0.2600691642747999799, -78.43909607169999276, 1.281852779972999734 ) ) ;
#15101=CARTESIAN_POINT ( 'NONE',  ( 1.153380192234999990, -78.70114559065000037, 1.148206073167999941 ) ) ;
#15135=CIRCLE ( 'NONE', #42491, 0.5000000000000004441 ) ;
#15141=CARTESIAN_POINT ( 'NONE',  ( 0.4771943503223999850, -80.47772667965000437, -1.596102929133000004 ) ) ;
#15142=CARTESIAN_POINT ( 'NONE',  ( 0.3401063316509999601, -79.66751968469999667, -1.168206624324999998 ) ) ;
#15144=CARTESIAN_POINT ( 'NONE',  ( -1.510119349581099168, -81.75199297495029782, -0.03898315715275646465 ) ) ;
#15147=CARTESIAN_POINT ( 'NONE',  ( 1.099580560635592841, -79.81033228112796962, -0.6005170649868118993 ) ) ;
#15151=CARTESIAN_POINT ( 'NONE',  ( 0.009713482255590434947, -81.72619256271893562, -1.249622119345054294 ) ) ;
#15181=CARTESIAN_POINT ( 'NONE',  ( -1.320073427535999988, -80.60725624888000596, 0.6433150820290999272 ) ) ;
#15186=CARTESIAN_POINT ( 'NONE',  ( -0.9178039125309811475, -79.67705081187436633, 1.199110755174137788 ) ) ;
#15200=CARTESIAN_POINT ( 'NONE',  ( 0.3875071078916553224, -78.45000632268018137, 1.188430056412658642 ) ) ;
#15209=CARTESIAN_POINT ( 'NONE',  ( -0.7507646060929270559, -82.02611842029168088, 1.015794618571693064 ) ) ;
#15225=CARTESIAN_POINT ( 'NONE',  ( 0.3273202981720256255, -78.24590025175641017, -1.217754575872296741 ) ) ;
#15235=CARTESIAN_POINT ( 'NONE',  ( 0.09617818635378815040, -82.73177828884955431, -1.246062951507001415 ) ) ;
#15242=CARTESIAN_POINT ( 'NONE',  ( 1.445648592326100879, -79.02717926386495151, 0.5087904774525755514 ) ) ;
#15248=CARTESIAN_POINT ( 'NONE',  ( 0.3271848554491016414, -81.14583333333331439, -1.217465845835393967 ) ) ;
#15263=CARTESIAN_POINT ( 'NONE',  ( -0.4818985169295156301, -83.00656079444637214, 1.153343561654186722 ) ) ;
#15265=CARTESIAN_POINT ( 'NONE',  ( 0.000000000000000000, -86.39999999999999147, 0.000000000000000000 ) ) ;
#15270=CARTESIAN_POINT ( 'NONE',  ( 0.000000000000000000, -87.09999999999999432, 0.000000000000000000 ) ) ;
#15289=ADVANCED_FACE ( 'NONE', ( #51405 ), #45584, .F. ) ;
#15290=CARTESIAN_POINT ( 'NONE',  ( 0.000000000000000000, -80.74999999950000529, 0.000000000000000000 ) ) ;
#15307=CARTESIAN_POINT ( 'NONE',  ( 0.4701211166820882248, -80.44441647165540132, 1.158161630332676273 ) ) ;
#15319=CARTESIAN_POINT ( 'NONE',  ( -1.145477160176213927, -80.13298459133737595, -0.5001054580953478990 ) ) ;
#15324=CARTESIAN_POINT ( 'NONE',  ( -1.522056959221183225, -78.83826870896211858, 0.2244679071987824293 ) ) ;
#15331=DIRECTION ( 'NONE',  ( -1.000000000000000000, 0.000000000000000000, 0.000000000000000000 ) ) ;
#15340=CARTESIAN_POINT ( 'NONE',  ( -1.223837560276999969, -82.48513558557799286, 0.5728811815464999180 ) ) ;
#15344=CARTESIAN_POINT ( 'NONE',  ( -1.092232985442824100, -82.95833333333330017, 0.6295237254636200097 ) ) ;
#15351=CARTESIAN_POINT ( 'NONE',  ( 0.5930780265196999856, -81.91886708904999637, 1.214178601635999888 ) ) ;
#15354=CARTESIAN_POINT ( 'NONE',  ( 0.9995835529977264988, -82.19791666666664298, -0.7681833999686417114 ) ) ;
#15372=CARTESIAN_POINT ( 'NONE',  ( 1.249826681154805552, -81.35774364365171607, 0.1170858793740336135 ) ) ;
#15403=CARTESIAN_POINT ( 'NONE',  ( -0.6794254437148999903, -78.97955343955000274, -1.478865823597000029 ) ) ;
#15404=AXIS2_PLACEMENT_3D ( 'NONE', #3237, #57246, #56961 ) ;
#15412=CARTESIAN_POINT ( 'NONE',  ( 0.4877854313978999268, -80.47814348455999323, -1.631527605715999973 ) ) ;
#15420=CARTESIAN_POINT ( 'NONE',  ( -0.9465222407332000154, -81.15663953506998496, -0.8164530897714000757 ) ) ;
#15437=CARTESIAN_POINT ( 'NONE',  ( -0.1383183815461396793, -79.98410570061048475, 1.242547978336307368 ) ) ;
#15443=CARTESIAN_POINT ( 'NONE',  ( 0.09717712410696000003, -79.38911183579999431, 1.316523976680999963 ) ) ;
#15445=CARTESIAN_POINT ( 'NONE',  ( -0.9969507628167146862, -82.31880644388637336, -1.182831566122873879 ) ) ;
#15447=B_SPLINE_CURVE_WITH_KNOTS ( 'NONE', 3,
 ( #22954, #32088, #49538, #31491, #45109, #4662, #9966, #840, #22662, #37104 ),
 .UNSPECIFIED., .F., .F.,
 ( 4, 2, 2, 2, 4 ),
 ( 0.000000000000000000, 0.2500000000000000000, 0.5000000000000000000, 0.7500000000000000000, 1.000000000000000000 ),
 .UNSPECIFIED. ) ;
#15453=CARTESIAN_POINT ( 'NONE',  ( -0.8609083542497767416, -81.66505337382136531, -0.9059207732458428586 ) ) ;
#15454=( NAMED_UNIT ( * ) PLANE_ANGLE_UNIT ( ) SI_UNIT ( $, .RADIAN. ) );
#15480=CARTESIAN_POINT ( 'NONE',  ( 0.3786699527928999442, -79.91281982998998501, -1.660248773968999947 ) ) ;
#15484=CARTESIAN_POINT ( 'NONE',  ( 1.509159946879168546, -79.50498243737588666, 0.09554436634639965065 ) ) ;
#15498=CARTESIAN_POINT ( 'NONE',  ( 1.213359460643753218, -78.36975490881563644, 0.3041480126303982567 ) ) ;
#15509=DIRECTION ( 'NONE',  ( 0.000000000000000000, 0.7071067811866525998, -0.7071067811864425456 ) ) ;
#15513=CARTESIAN_POINT ( 'NONE',  ( -1.250000000000000000, -83.49999999999998579, 0.000000000000000000 ) ) ;
#15521=CARTESIAN_POINT ( 'NONE',  ( -0.1636548025077330659, -78.21466361286708491, -1.249383312717734063 ) ) ;
#15533=CARTESIAN_POINT ( 'NONE',  ( 0.2662832580731058774, -82.74250220263775191, -1.221068703491243079 ) ) ;
#15537=CARTESIAN_POINT ( 'NONE',  ( 1.411986188763491912, -77.96846487410871873, -0.5961744733279076280 ) ) ;
#15543=CARTESIAN_POINT ( 'NONE',  ( -1.443009460674115063, -81.32505097460641252, 0.4563349844573089120 ) ) ;
#15558=CARTESIAN_POINT ( 'NONE',  ( -0.4931998282677043655, -83.00735135618793947, 1.148627814754535903 ) ) ;
#15580=CARTESIAN_POINT ( 'NONE',  ( -1.552248384014999871, -82.85925875911100036, 0.6048007385293000526 ) ) ;
#15583=EDGE_LOOP ( 'NONE', ( #14812, #7976, #57421, #19673 ) ) ;
#15590=EDGE_CURVE ( 'NONE', #35380, #1475, #3812, .T. ) ;
#15591=CARTESIAN_POINT ( 'NONE',  ( 0.02044571250362530943, -80.72695277621694743, -1.249496931604304084 ) ) ;
#15598=VERTEX_POINT ( 'NONE', #15828 ) ;
#15600=CARTESIAN_POINT ( 'NONE',  ( 0.8777382552776737956, -80.41361731832262194, 0.8895207107364466736 ) ) ;
#15613=CARTESIAN_POINT ( 'NONE',  ( -0.2201962894297133100, -78.46348357500299642, -1.520989522816315054 ) ) ;
#15627=CARTESIAN_POINT ( 'NONE',  ( 0.2545367188273338632, -80.11228258266474711, 1.524467069150255982 ) ) ;
#15640=CARTESIAN_POINT ( 'NONE',  ( 0.000000000000000000, -86.20000000000000284, 0.000000000000000000 ) ) ;
#15655=CARTESIAN_POINT ( 'NONE',  ( 0.5173187029184005414, -81.44118298419677160, 1.138630597744533679 ) ) ;
#15690=CARTESIAN_POINT ( 'NONE',  ( 1.341343219651000229, -79.03170025523999698, -0.9216622887798999741 ) ) ;
#15700=CARTESIAN_POINT ( 'NONE',  ( -0.9181250412607999678, -79.90971054856998990, -1.434176897702999831 ) ) ;
#15710=DIRECTION ( 'NONE',  ( 0.000000000000000000, -1.000000000000000000, 0.000000000000000000 ) ) ;
#15734=CARTESIAN_POINT ( 'NONE',  ( 1.382775425143483394, -83.06597328304708583, -0.6152231662640477161 ) ) ;
#15735=CARTESIAN_POINT ( 'NONE',  ( -0.5441368889797353336, -79.68939737495202280, -1.127482903650173229 ) ) ;
#15743=VERTEX_POINT ( 'NONE', #25656 ) ;
#15766=CARTESIAN_POINT ( 'NONE',  ( 0.3526082373300999939, -79.84950314121999781, -1.545983222067000007 ) ) ;
#15789=CARTESIAN_POINT ( 'NONE',  ( -0.0009180708875000889333, -78.47527983758934056, 1.249867243019089358 ) ) ;
#15796=CARTESIAN_POINT ( 'NONE',  ( -3.000000000000000000, -86.20000000000000284, 0.000000000000000000 ) ) ;
#15800=CARTESIAN_POINT ( 'NONE',  ( -1.218115782252727985, -82.07993943974406648, 0.3280300537313449727 ) ) ;
#15817=VERTEX_POINT ( 'NONE', #35971 ) ;
#15824=CARTESIAN_POINT ( 'NONE',  ( -1.093100964505588690, -82.64204610221628400, -0.6296463513202182893 ) ) ;
#15828=CARTESIAN_POINT ( 'NONE',  ( -1.250000000000000000, -80.00000000000000000, 0.000000000000000000 ) ) ;
#15829=CARTESIAN_POINT ( 'NONE',  ( -0.3042520966058857579, -78.64066448665755615, 1.500984266365883446 ) ) ;
#15831=B_SPLINE_SURFACE_WITH_KNOTS ( 'NONE', 3, 3, ( 
 ( #20237, #33790, #24945, #56251, #42965, #38522, #56537, #52684, #30230, #34368, #52114, #57401, #16098, #7230, #25234, #16959, #12239, #43254, #2810, #20804, #38811, #31384, #49124, #31678, #35224, #8378, #39673, #40259, #49425, #22248, #40851, #44991, #27252, #53551, #31971 ),
 ( #36412, #53254, #57975, #44395, #18421, #54440, #21950, #443, #3667, #13976, #49724, #45292, #17531, #8975, #57679, #44696, #50014, #22838, #21667, #40560, #35522, #12804, #13090, #9560, #4251, #39962, #58272, #27544, #17237, #4842, #30803, #54140, #48836, #8674, #31087 ),
 ( #26663, #3947, #26376, #17835, #9267, #35823, #53852, #13384, #26961, #4547, #22549, #36124, #153, #18129, #13680, #28713, #45881, #33137, #24302, #50598, #46465, #46765, #14846, #32549, #33437, #5993, #51473, #42316, #55891, #23999, #42017, #1884, #1587, #41433, #19577 ),
 ( #15142, #1019, #41139, #19878, #32258, #37871, #15443, #10737, #23711, #18710, #10147, #54719, #11030, #5133, #6287, #19000, #50887, #730, #28124, #45588, #23130, #36704, #37576, #36992, #14262, #55008, #50304, #46174, #23421, #5700, #9854, #27835, #5413, #14556, #55593 ) ),
 .UNSPECIFIED., .F., .F., .F.,
 ( 4, 4 ),
 ( 4, 1, 1, 1, 1, 1, 1, 1, 1, 1, 1, 1, 1, 1, 1, 1, 1, 1, 1, 1, 1, 1, 1, 1, 1, 1, 1, 1, 1, 1, 1, 1, 4 ),
 ( -0.1331668876848000060, 1.133166887685000068 ),
 ( -0.01763212848115999765, 0.01102008030072000079, 0.03967228908261000164, 0.06832449786448999141, 0.09697670664638000093, 0.1256289154283000142, 0.1542811242101000124, 0.1829333329919999862, 0.2115855417738999877, 0.2402377505557999893, 0.2688899593376999908, 0.2975421681195999923, 0.3261943769014999939, 0.3548465856833000198, 0.3834987944651999658, 0.4121510032471000229, 0.4408032120290000244, 0.4694554208109000260, 0.4981076295927999720, 0.5267598383746000534, 0.5554120471565000550, 0.5840642559384000565, 0.6127164647203000580, 0.6413686735021999485, 0.6700208822840999501, 0.6986730910659999516, 0.7273252998478000331, 0.7559775086296999236, 0.7846297174115999251, 0.8132819261935000377, 0.8419341349753999282, 0.8705863437573000407, 0.8992385525391000112 ),
 .UNSPECIFIED. ) ;
#15848=CARTESIAN_POINT ( 'NONE',  ( -0.4784572937601109799, -83.00632309593854075, 1.154759755059053150 ) ) ;
#15871=CARTESIAN_POINT ( 'NONE',  ( -1.324613189995999862, -83.42769169510199845, -0.7038465009425000085 ) ) ;
#15890=CARTESIAN_POINT ( 'NONE',  ( 1.021667840366504487, -80.39937480585440710, 0.7203988087165839049 ) ) ;
#15907=EDGE_CURVE ( 'NONE', #42991, #7477, #44251, .T. ) ;
#15919=CARTESIAN_POINT ( 'NONE',  ( 1.490312334586760157, -81.01311113150978827, 0.2476722647248059406 ) ) ;
#15946=CARTESIAN_POINT ( 'NONE',  ( 1.118977020825177249, -81.38716913225974281, 0.5574429764450725688 ) ) ;
#15948=CARTESIAN_POINT ( 'NONE',  ( -1.093124704215232557, -82.14231321599577029, -0.6293855122744574926 ) ) ;
#15958=EDGE_LOOP ( 'NONE', ( #10881, #24755, #4264, #4412 ) ) ;
#15962=AXIS2_PLACEMENT_3D ( 'NONE', #26427, #4895, #12853 ) ;
#15970=LINE ( 'NONE', #11554, #17097 ) ;
#15971=ORIENTED_EDGE ( 'NONE', *, *, #6507, .F. ) ;
#15982=CARTESIAN_POINT ( 'NONE',  ( -1.578837173282999995, -79.36932442800998899, 0.3948290484592000271 ) ) ;
#15993=CARTESIAN_POINT ( 'NONE',  ( -0.5553526962645999321, -81.42553171121998901, -1.429183993495000138 ) ) ;
#16007=FACE_OUTER_BOUND ( 'NONE', #27848, .T. ) ;
#16028=CARTESIAN_POINT ( 'NONE',  ( -0.7285324502130352542, -82.93438848133038732, -1.325323562101084152 ) ) ;
#16029=CARTESIAN_POINT ( 'NONE',  ( 0.9143677338810914934, -79.79065590062214142, -0.8521684201040128359 ) ) ;
#16051=ORIENTED_EDGE ( 'NONE', *, *, #41797, .F. ) ;
#16060=CARTESIAN_POINT ( 'NONE',  ( -1.576937714420000081, -81.23916334729999278, 0.6430338560479000876 ) ) ;
#16064=CARTESIAN_POINT ( 'NONE',  ( -0.1057940869841550030, -79.86936252454921714, -1.506682504695135982 ) ) ;
#16083=CARTESIAN_POINT ( 'NONE',  ( 0.8124100789227103325, -78.41886625915758202, 0.9503163788704104276 ) ) ;
#16098=CARTESIAN_POINT ( 'NONE',  ( -1.504841238612000032, -78.86507235081998601, -0.7092193051005999394 ) ) ;
#16107=CARTESIAN_POINT ( 'NONE',  ( -1.249634766890562743, -78.11054148323580648, -0.1635212922017194592 ) ) ;
#16122=CARTESIAN_POINT ( 'NONE',  ( 0.4024786306066807651, -79.44944984597937321, 1.183223541616218011 ) ) ;
#16123=CARTESIAN_POINT ( 'NONE',  ( -0.9504519148020524888, -79.17842417668877886, 1.203406266442021977 ) ) ;
#16131=CARTESIAN_POINT ( 'NONE',  ( -0.7271731550489020091, -81.26431952766002098, 1.327098488219002004 ) ) ;
#16136=B_SPLINE_CURVE_WITH_KNOTS ( 'NONE', 3,
 ( #5996, #46178, #42319, #733, #19881, #24002, #33440, #37874, #51476, #5703, #32843, #54722, #14265, #32262, #50307, #9857, #27839, #52052, #15734, #34594, #2174, #21030, #25169, #51765, #29872, #2458, #12174, #16028, #11609, #57331, #43476, #34306, #47640, #7164, #29583, #43192, #52337, #52906, #52622, #11317, #30161, #47925, #2745, #7458, #48210, #7743, #33730, #24596, #25742, #6874, #43769, #34877, #16894, #11893, #42610, #20746, #25457, #24883, #38744, #56186, #56764, #16324, #3319, #38162, #12455, #3033, #20463, #39036, #42899, #30451, #6585, #57047, #16606, #29297, #47346, #21313, #39324, #34016, #20174, #38455, #56472, #35448, #54074, #371, #18352, #45219, #4181, #22475, #8026, #22177, #30733, #26313, #26022, #22769, #26894, #27181, #36342, #58200, #4768, #54368, #40486, #35750, #57612, #53480, #17172, #18059, #44051, #31019 ),
 .UNSPECIFIED., .F., .F.,
 ( 4, 2, 2, 2, 2, 2, 1, 2, 2, 2, 2, 2, 2, 2, 2, 2, 2, 2, 2, 2, 2, 2, 2, 2, 2, 2, 2, 2, 2, 2, 2, 2, 2, 2, 2, 2, 2, 2, 2, 2, 2, 2, 2, 2, 2, 2, 2, 2, 1, 2, 2, 2, 2, 2, 4 ),
 ( 0.000000000000000000, 0.01562500000000003469, 0.03125000000000006939, 0.04687500000000011796, 0.06250000000000016653, 0.07812500000000022204, 0.09375000000000024980, 0.1093750000000002914, 0.1250000000000003331, 0.1406250000000003608, 0.1562500000000004163, 0.1718750000000004441, 0.1875000000000004718, 0.2031250000000004996, 0.2187500000000005274, 0.2343750000000005274, 0.2500000000000004996, 0.2656250000000005551, 0.2812500000000005551, 0.2968750000000006106, 0.3125000000000006106, 0.3281250000000006661, 0.3437500000000007216, 0.3750000000000007216, 0.4062500000000007216, 0.4375000000000007216, 0.4687500000000007772, 0.5000000000000007772, 0.5312500000000007772, 0.5625000000000006661, 0.5937500000000006661, 0.6250000000000005551, 0.6562500000000005551, 0.6718750000000005551, 0.6875000000000006661, 0.7031250000000005551, 0.7187500000000004441, 0.7343750000000004441, 0.7500000000000003331, 0.7656250000000002220, 0.7812500000000002220, 0.7968750000000001110, 0.8125000000000000000, 0.8281250000000001110, 0.8437500000000001110, 0.8593750000000001110, 0.8750000000000001110, 0.8906250000000002220, 0.9062500000000002220, 0.9218750000000002220, 0.9375000000000003331, 0.9531250000000002220, 0.9687500000000001110, 0.9843750000000001110, 1.000000000000000000 ),
 .UNSPECIFIED. ) ;
#16175=CARTESIAN_POINT ( 'NONE',  ( -1.171666301184231207, -80.63007484519644663, -0.4570117860640778851 ) ) ;
#16183=CARTESIAN_POINT ( 'NONE',  ( 0.3529067879003955910, -80.45250755409055898, 1.199236710938469397 ) ) ;
#16189=ORIENTED_EDGE ( 'NONE', *, *, #5513, .T. ) ;
#16202=ADVANCED_FACE ( 'NONE', ( #36487 ), #49502, .F. ) ;
#16211=CARTESIAN_POINT ( 'NONE',  ( -0.3722592371509435560, -81.14469282965922048, 1.465311301645253916 ) ) ;
#16220=CARTESIAN_POINT ( 'NONE',  ( -1.115197308773999918, -81.11885036431999652, -0.5833774300368999022 ) ) ;
#16239=CARTESIAN_POINT ( 'NONE',  ( -0.4457402708948181580, -81.50411655302407610, 1.168277140437457895 ) ) ;
#16240=CARTESIAN_POINT ( 'NONE',  ( -0.8981901762082999952, -79.90929374366000104, -1.403037214508999986 ) ) ;
#16255=CARTESIAN_POINT ( 'NONE',  ( -1.277911487367000110, -78.60727590003000387, 0.6223777146390999659 ) ) ;
#16256=ORIENTED_EDGE ( 'NONE', *, *, #47997, .T. ) ;
#16278=CARTESIAN_POINT ( 'NONE',  ( 0.3877229342594999961, -77.97375042942999812, -1.580612325761999948 ) ) ;
#16289=CARTESIAN_POINT ( 'NONE',  ( -0.7740797122817000275, -83.24257374592500014, 1.516913212488000040 ) ) ;
#16290=CARTESIAN_POINT ( 'NONE',  ( -0.5437916395094000155, -79.48880658815998856, -1.373128015768000143 ) ) ;
#16295=AXIS2_PLACEMENT_3D ( 'NONE', #15640, #42514, #33919 ) ;
#16323=AXIS2_PLACEMENT_3D ( 'NONE', #46291, #6404, #1417 ) ;
#16324=CARTESIAN_POINT ( 'NONE',  ( 1.189282163301631279, -82.15500157885483645, 0.9888244770500705938 ) ) ;
#16326=CARTESIAN_POINT ( 'NONE',  ( 0.02451244981669795098, -79.72693319877517126, -1.249557414888817997 ) ) ;
#16354=CARTESIAN_POINT ( 'NONE',  ( 0.2491193812340000147, -79.34422942033999959, -1.565693046525999943 ) ) ;
#16360=EDGE_CURVE ( 'NONE', #56978, #20349, #52349, .T. ) ;
#16369=DIRECTION ( 'NONE',  ( 1.000000000000000000, 0.000000000000000000, 0.000000000000000000 ) ) ;
#16371=CARTESIAN_POINT ( 'NONE',  ( 0.7572423792512895657, -78.42344112683323942, 0.9945924809264382604 ) ) ;
#16383=CARTESIAN_POINT ( 'NONE',  ( -0.2929820310045200271, -81.99426728663597430, 1.218107854444346216 ) ) ;
#16393=B_SPLINE_CURVE_WITH_KNOTS ( 'NONE', 3,
 ( #30713, #48750, #8293, #53458, #22159, #17745 ),
 .UNSPECIFIED., .F., .F.,
 ( 4, 2, 4 ),
 ( 0.000000000000000000, 0.5000000000000000000, 1.000000000000000000 ),
 .UNSPECIFIED. ) ;
#16402=ORIENTED_EDGE ( 'NONE', *, *, #46126, .T. ) ;
#16411=CARTESIAN_POINT ( 'NONE',  ( -0.08250089784128371295, -79.48042012904160458, 1.249901427480934135 ) ) ;
#16412=CARTESIAN_POINT ( 'NONE',  ( -0.8863621734748006187, -78.67427446728444806, 1.251082152859870344 ) ) ;
#16469=CARTESIAN_POINT ( 'NONE',  ( -0.5354806933557879622, -80.51039173408095451, 1.129579107287216777 ) ) ;
#16478=CONICAL_SURFACE ( 'NONE', #20319, 2.949999999500999781, 0.7853981633972997312 ) ;
#16485=AXIS2_PLACEMENT_3D ( 'NONE', #35537, #31987, #5146 ) ;
#16487=CARTESIAN_POINT ( 'NONE',  ( -0.3707198704570134340, -77.95484660748586236, -1.462871543653826656 ) ) ;
#16498=CARTESIAN_POINT ( 'NONE',  ( 0.5212184487221598328, -80.59812269889569336, 1.458433989672604625 ) ) ;
#16499=CARTESIAN_POINT ( 'NONE',  ( 1.092232985442820992, -79.29166666666664298, 0.6295237254636267821 ) ) ;
#16507=CARTESIAN_POINT ( 'NONE',  ( -1.438065998794000100, -83.22447248197899228, -0.3363867981957999742 ) ) ;
#16528=CARTESIAN_POINT ( 'NONE',  ( -0.8906226101088000613, -79.40402002277998861, -1.206976125017999779 ) ) ;
#16529=VERTEX_POINT ( 'NONE', #47900 ) ;
#16540=CARTESIAN_POINT ( 'NONE',  ( -1.031488621067000011, -78.08296020222998379, 0.9779790477098000423 ) ) ;
#16557=CARTESIAN_POINT ( 'NONE',  ( 0.6295237254636258939, -83.16666666666667140, -1.092232985442821658 ) ) ;
#16561=CARTESIAN_POINT ( 'NONE',  ( 0.000000000000000000, -80.69999999999998863, 0.000000000000000000 ) ) ;
#16571=CARTESIAN_POINT ( 'NONE',  ( -1.495211702480000016, -81.34779729262000103, -0.3395960383748000133 ) ) ;
#16572=CARTESIAN_POINT ( 'NONE',  ( -1.376297233339999870, -80.35198252799999352, 0.7875294559552000750 ) ) ;
#16575=CARTESIAN_POINT ( 'NONE',  ( -1.250000000000000000, -79.50000000000000000, 0.000000000000000000 ) ) ;
#16587=ADVANCED_FACE ( 'NONE', ( #28990 ), #42586, .F. ) ;
#16589=CARTESIAN_POINT ( 'NONE',  ( -1.596536837631000072, -81.85265420858999619, -0.4757406268331999533 ) ) ;
#16599=CARTESIAN_POINT ( 'NONE',  ( -1.216847505586732492, -80.08203192589257924, 0.2879019704867851193 ) ) ;
#16601=MECHANICAL_DESIGN_GEOMETRIC_PRESENTATION_REPRESENTATION('',(#24135),#5957);
#16606=CARTESIAN_POINT ( 'NONE',  ( -0.5901797316841597141, -81.94244151454432767, -1.393023506703266357 ) ) ;
#16608=CARTESIAN_POINT ( 'NONE',  ( -0.1504192046052299503, -79.71605312332511062, -1.243133251493206304 ) ) ;
#16622=CARTESIAN_POINT ( 'NONE',  ( -0.8932107854388791068, -77.79557291679432751, -1.163659720379709883 ) ) ;
#16638=CARTESIAN_POINT ( 'NONE',  ( -1.478021081765000133, -80.22861590553999633, 0.8457367421919999018 ) ) ;
#16656=ORIENTED_EDGE ( 'NONE', *, *, #40352, .F. ) ;
#16665=LINE ( 'NONE', #52963, #16740 ) ;
#16674=CARTESIAN_POINT ( 'NONE',  ( 0.3246040448838053982, -81.95449045088716389, 1.207607888008069619 ) ) ;
#16702=CARTESIAN_POINT ( 'NONE',  ( -1.020136227765584547, -77.81721996128494823, -1.142300944648168670 ) ) ;
#16718=CARTESIAN_POINT ( 'NONE',  ( 1.233429448859959754, -82.86411798178254173, 0.2149029772794059101 ) ) ;
#16740=VECTOR ( 'NONE', #53245, 1000.000000000000000 ) ;
#16772=CARTESIAN_POINT ( 'NONE',  ( 0.000000000000000000, -80.74999999950000529, 0.000000000000000000 ) ) ;
#16774=VECTOR ( 'NONE', #11537, 1000.000000000000000 ) ;
#16786=CARTESIAN_POINT ( 'NONE',  ( 1.250000000000000222, -78.73958333333331439, -0.1636246173744659582 ) ) ;
#16787=CARTESIAN_POINT ( 'NONE',  ( -0.2601825140295693228, -80.86128609518755184, -1.488047444107771344 ) ) ;
#16788=LINE ( 'NONE', #48099, #50407 ) ;
#16797=CARTESIAN_POINT ( 'NONE',  ( 1.160935205181999885, -81.28727493794998793, -0.6914862246935000734 ) ) ;
#16811=DIRECTION ( 'NONE',  ( 0.000000000000000000, -1.000000000000000000, 0.000000000000000000 ) ) ;
#16817=CARTESIAN_POINT ( 'NONE',  ( -1.529754383668999962, -81.36195569118999060, -0.6588408878327000062 ) ) ;
#16824=CARTESIAN_POINT ( 'NONE',  ( -0.7681833999686477066, -78.42708333333334281, 0.9995835529977223910 ) ) ;
#16847=CARTESIAN_POINT ( 'NONE',  ( -0.1636246173744673738, -83.11458333333330017, -1.249999999999999778 ) ) ;
#16854=CARTESIAN_POINT ( 'NONE',  ( -1.104290071782900062, -79.13894817590623632, -0.5871211644529236162 ) ) ;
#16862=CARTESIAN_POINT ( 'NONE',  ( -0.8549356769920000154, -79.97302723733999130, -1.335470596990000036 ) ) ;
#16866=CARTESIAN_POINT ( 'NONE',  ( -1.552248384014999871, -82.68160978750299250, 0.6048007385293000526 ) ) ;
#16880=CARTESIAN_POINT ( 'NONE',  ( 0.7076411874954000591, -82.98952008057199237, -1.508144869335000138 ) ) ;
#16893=CARTESIAN_POINT ( 'NONE',  ( -0.6531259097149988424, -79.01686433677801347, 1.115453275870143202 ) ) ;
#16894=CARTESIAN_POINT ( 'NONE',  ( -0.9976315024470040482, -82.41817118228848926, -1.183693355290223570 ) ) ;
#16901=VERTEX_POINT ( 'NONE', #41971 ) ;
#16912=B_SPLINE_CURVE_WITH_KNOTS ( 'NONE', 3,
 ( #2739, #11309, #43184, #7450, #16599, #56757, #3025, #52331, #20166, #34009, #21023, #42603, #43470, #11886, #47338, #29864, #57040, #34585, #2166, #56177, #51758, #29290, #6867, #55887, #52616, #24876, #42893, #28708, #6278, #24295, #20453, #47047, #42310, #1877, #56466, #11024, #19872, #52044, #37866, #11601, #15437, #29007, #51468, #29577, #47634, #57899, #17166, #57606, #17756, #53473, #8020, #13014, #39602, #21597, #26016, #13310, #30727, #25735, #31013, #12733, #44323, #8894, #49051, #8599, #26888, #26585, #44042, #44619, #39316, #48762, #73, #4175, #22467, #17456, #35152, #3592, #3313, #22172, #57325, #30445, #21878, #53185, #35442, #43762, #8308, #31305 ),
 .UNSPECIFIED., .F., .F.,
 ( 4, 2, 2, 2, 1, 1, 2, 2, 2, 2, 2, 1, 1, 2, 2, 2, 2, 1, 1, 1, 2, 2, 2, 2, 2, 1, 1, 2, 2, 2, 2, 2, 1, 1, 2, 2, 2, 2, 2, 1, 1, 2, 2, 2, 2, 1, 1, 1, 2, 2, 4 ),
 ( 0.000000000000000000, 0.06250000000000065226, 0.09375000000000101308, 0.1093750000000011796, 0.1171875000000012490, 0.1210937500000010408, 0.1230468750000006661, 0.1250000000000002776, 0.1874999999999829581, 0.2187499999999746869, 0.2343749999999705791, 0.2421874999999685252, 0.2460937499999677480, 0.2480468749999675537, 0.2499999999999673872, 0.3124999999999732991, 0.3437499999999761857, 0.3593749999999776290, 0.3671874999999786282, 0.3710937499999789058, 0.3730468749999790723, 0.3749999999999792388, 0.4374999999999646394, 0.4687499999999570344, 0.4843749999999532041, 0.4921874999999515943, 0.4960937499999504841, 0.4980468749999502065, 0.4999999999999498734, 0.5624999999999505951, 0.5937499999999512612, 0.6093749999999515943, 0.6171874999999518163, 0.6210937499999518163, 0.6230468749999517053, 0.6249999999999514833, 0.6874999999999450440, 0.7187499999999413802, 0.7343749999999392708, 0.7421874999999382716, 0.7460937499999377165, 0.7480468749999377165, 0.7499999999999377165, 0.8124999999999399369, 0.8437499999999413802, 0.8593749999999421574, 0.8671874999999426015, 0.8710937499999427125, 0.8730468749999427125, 0.8749999999999427125, 1.000000000000000000 ),
 .UNSPECIFIED. ) ;
#16927=CARTESIAN_POINT ( 'NONE',  ( -1.217465845835394411, -81.02083333333330017, -0.3271848554491003647 ) ) ;
#16954=DIRECTION ( 'NONE',  ( -1.000000000000000000, 0.000000000000000000, 0.000000000000000000 ) ) ;
#16958=CARTESIAN_POINT ( 'NONE',  ( 0.2007160378926907962, -81.96275121485238913, 1.233601532853040750 ) ) ;
#16959=CARTESIAN_POINT ( 'NONE',  ( 0.1460928719284999844, -78.69802764147999596, 1.657165064314999992 ) ) ;
#16976=ORIENTED_EDGE ( 'NONE', *, *, #47448, .T. ) ;
#17004=CARTESIAN_POINT ( 'NONE',  ( 1.250000000000000000, -82.84999999999999432, 0.000000000000000000 ) ) ;
#17046=AXIS2_PLACEMENT_3D ( 'NONE', #49204, #53935, #18499 ) ;
#17055=CARTESIAN_POINT ( 'NONE',  ( -0.8328560967162584872, -77.92807624077448736, -1.259433156755825012 ) ) ;
#17066=CARTESIAN_POINT ( 'NONE',  ( 1.092232985442823212, -78.70833333333331439, -0.6295237254636224522 ) ) ;
#17067=CARTESIAN_POINT ( 'NONE',  ( 1.459813637468974301, -80.12054394350599296, 0.3988620006733276657 ) ) ;
#17076=CARTESIAN_POINT ( 'NONE',  ( -1.400413196275999805, -83.11904964980398347, 0.4410028580390000230 ) ) ;
#17097=VECTOR ( 'NONE', #51999, 1000.000000000000114 ) ;
#17109=CARTESIAN_POINT ( 'NONE',  ( -1.215029926349999956, -77.61107607421000409, 0.5215463190299000074 ) ) ;
#17127=CARTESIAN_POINT ( 'NONE',  ( -1.249999999999999778, -83.01041666666662877, -0.1636246173744686228 ) ) ;
#17135=DIRECTION ( 'NONE',  ( 0.000000000000000000, 1.000000000000000000, 0.000000000000000000 ) ) ;
#17142=CARTESIAN_POINT ( 'NONE',  ( -0.4406873220133000202, -81.61548177752000299, -1.134095991600000186 ) ) ;
#17146=CARTESIAN_POINT ( 'NONE',  ( -1.588687380433000174, -83.18688350838499446, 0.5002921117598999601 ) ) ;
#17151=CARTESIAN_POINT ( 'NONE',  ( 0.000000000000000000, -87.20000000000000284, 0.000000000000000000 ) ) ;
#17166=CARTESIAN_POINT ( 'NONE',  ( -0.007339070148793539611, -79.97594915642548585, 1.249695971876270129 ) ) ;
#17172=CARTESIAN_POINT ( 'NONE',  ( -0.5209265914808703934, -81.44646803115288947, -1.419575930094677751 ) ) ;
#17237=CARTESIAN_POINT ( 'NONE',  ( 0.3690512077139999625, -78.03748392311000259, -1.504494153444999816 ) ) ;
#17239=CARTESIAN_POINT ( 'NONE',  ( 0.9042486337774866545, -82.92610658917844546, -1.210803591118944089 ) ) ;
#17267=CARTESIAN_POINT ( 'NONE',  ( -1.500000000000000000, -83.24999999999998579, 0.000000000000000000 ) ) ;
#17353=CARTESIAN_POINT ( 'NONE',  ( -1.217210213920586703, -80.89993084598471285, -0.8960687109477767365 ) ) ;
#17365=CARTESIAN_POINT ( 'NONE',  ( 0.6237791458550000501, -82.80325357425300581, -1.329415719495999904 ) ) ;
#17388=CARTESIAN_POINT ( 'NONE',  ( 0.000000000000000000, -83.49999999999998579, 0.000000000000000000 ) ) ;
#17402=CARTESIAN_POINT ( 'NONE',  ( 0.8868875279287172786, -80.28835734964251003, -0.8803813265097053531 ) ) ;
#17415=CYLINDRICAL_SURFACE ( 'NONE', #18334, 1.250000000000000000 ) ;
#17419=CARTESIAN_POINT ( 'NONE',  ( 3.000000000000000000, -80.79999999999999716, 0.000000000000000000 ) ) ;
#17423=CARTESIAN_POINT ( 'NONE',  ( -1.154999620367486157, -83.06888870240290146, 0.4778175114515754163 ) ) ;
#17428=CARTESIAN_POINT ( 'NONE',  ( -1.407332420019999919, -81.97970439103998785, -0.4193609517060999936 ) ) ;
#17431=CARTESIAN_POINT ( 'NONE',  ( 1.401632346086000069, -80.60461938843998553, -0.7415008327037999614 ) ) ;
#17439=DIRECTION ( 'NONE',  ( 1.000000000000000000, 0.000000000000000000, 0.000000000000000000 ) ) ;
#17447=CARTESIAN_POINT ( 'NONE',  ( -0.6572886123566999972, -82.73688322013099139, 1.530761476772000140 ) ) ;
#17453=DIRECTION ( 'NONE',  ( -1.000000000000000000, 0.000000000000000000, 0.000000000000000000 ) ) ;
#17456=CARTESIAN_POINT ( 'NONE',  ( 0.9801167568178164036, -79.90410533936980642, 0.7793211621830089531 ) ) ;
#17483=CARTESIAN_POINT ( 'NONE',  ( -0.1625384163739970467, -79.48544409746807560, 1.242284532507756278 ) ) ;
#17485=EDGE_LOOP ( 'NONE', ( #28298, #6296, #27388 ) ) ;
#17530=CARTESIAN_POINT ( 'NONE',  ( 1.167992134012648231, -81.87908179006763021, 0.4465703791935540234 ) ) ;
#17531=CARTESIAN_POINT ( 'NONE',  ( -1.401271510176000046, -78.92838903957999719, -0.6604077434914998879 ) ) ;
#17533=CARTESIAN_POINT ( 'NONE',  ( 1.490703458528794600, -82.98683660370730308, -0.2499861325332328188 ) ) ;
#17540=CARTESIAN_POINT ( 'NONE',  ( 1.042299842011717770, -81.80361443818746636, -0.6898479045106226115 ) ) ;
#17544=DIRECTION ( 'NONE',  ( 0.7071067811865969777, -0.7071067811864980568, -1.359271113201994007E-10 ) ) ;
#17545=ORIENTED_EDGE ( 'NONE', *, *, #13563, .T. ) ;
#17638=CARTESIAN_POINT ( 'NONE',  ( -1.250000000000000000, -79.50000000000000000, 0.000000000000000000 ) ) ;
#17651=CARTESIAN_POINT ( 'NONE',  ( -1.404361994020937088, -80.87968703033534723, -0.5636150327419870987 ) ) ;
#17652=CARTESIAN_POINT ( 'NONE',  ( -1.250000000000000000, -78.60000000000000853, 0.000000000000000000 ) ) ;
#17663=CARTESIAN_POINT ( 'NONE',  ( 0.7473949548134999343, -82.10881715536000058, 1.530103832088000049 ) ) ;
#17682=CARTESIAN_POINT ( 'NONE',  ( -1.630114970985000022, -79.90535085241999980, -0.3434887894992000312 ) ) ;
#17692=EDGE_CURVE ( 'NONE', #45372, #31856, #51302, .T. ) ;
#17701=CARTESIAN_POINT ( 'NONE',  ( 0.4964284668415000490, -78.41931985888000156, -1.571764949136999823 ) ) ;
#17732=CARTESIAN_POINT ( 'NONE',  ( -1.285835855790000037, -81.91654517592999696, 0.7092774996876000104 ) ) ;
#17733=CARTESIAN_POINT ( 'NONE',  ( -0.6515920321739999688, -80.60493433575999234, -1.183807013712999900 ) ) ;
#17737=CARTESIAN_POINT ( 'NONE',  ( -0.5544740949720999845, -82.17239317537999455, 1.570928860995999932 ) ) ;
#17745=CARTESIAN_POINT ( 'NONE',  ( -1.250000000000000000, -79.50000000000000000, 0.000000000000000000 ) ) ;
#17756=CARTESIAN_POINT ( 'NONE',  ( 0.06191098829455312508, -79.97165892281826416, 1.249638892610136720 ) ) ;
#17778=AXIS2_PLACEMENT_3D ( 'NONE', #53151, #7984, #2988 ) ;
#17783=CARTESIAN_POINT ( 'NONE',  ( 0.8704580601414534380, -79.41396526092823649, 0.8969229247981558295 ) ) ;
#17800=VERTEX_POINT ( 'NONE', #35204 ) ;
#17820=AXIS2_PLACEMENT_3D ( 'NONE', #6018, #24028, #32574 ) ;
#17828=TOROIDAL_SURFACE ( 'NONE', #22543, 9.000000000000000000, 0.5000000000000000000 ) ;
#17834=CARTESIAN_POINT ( 'NONE',  ( 0.2617232932829000047, -79.34874659015000020, -1.644907507304999905 ) ) ;
#17835=CARTESIAN_POINT ( 'NONE',  ( -1.288905872365999850, -79.49283985636999716, -0.6300432575161000193 ) ) ;
#17837=CARTESIAN_POINT ( 'NONE',  ( -1.007661242079784136, -82.68318653106200600, 1.124876851017058588 ) ) ;
#17847=CARTESIAN_POINT ( 'NONE',  ( -0.7681833999686432657, -80.07291666666668561, -0.9995835529977258327 ) ) ;
#17860=ORIENTED_EDGE ( 'NONE', *, *, #7817, .F. ) ;
#17874=CARTESIAN_POINT ( 'NONE',  ( 1.258195058187999926, -80.85973563566999189, 0.4928692076250000276 ) ) ;
#17906=CARTESIAN_POINT ( 'NONE',  ( -0.6295237254636286695, -82.41666666666667140, 1.092232985442819881 ) ) ;
#17920=B_SPLINE_SURFACE_WITH_KNOTS ( 'NONE', 3, 3, ( 
 ( #41629, #37480, #1209, #19201, #29202, #42224, #55206, #10639, #51090, #28621, #46666, #6193, #46959, #6779, #20079, #24206, #1789, #19785, #37779, #55800, #15351, #10934, #11223, #47247, #24787, #53375, #57232, #56947, #43369, #21504, #16797, #34781, #11792, #16220, #39511 ),
 ( #52805, #34489, #17076, #20646, #52236, #53093, #57805, #17365, #44234, #26218, #30347, #12645, #38930, #29767, #25354, #25071, #21788, #56664, #43665, #8216, #12076, #3787, #47824, #39792, #7354, #12358, #34198, #43094, #35351, #2928, #12924, #3502, #7640, #35058, #30638 ),
 ( #20929, #16507, #47545, #48108, #52519, #25640, #7069, #2652, #48672, #30057, #57516, #3224, #21211, #39219, #48389, #7927, #25927, #43951, #41272, #9101, #36546, #22679, #32104, #50145, #18552, #14107, #40390, #22972, #35650, #53678, #36254, #9688, #31212, #54568, #27675 ),
 ( #13809, #45721, #5256, #31811, #40982, #49251, #856, #18840, #573, #23263, #48960, #4377, #36833, #13218, #45423, #54846, #8503, #26794, #26498, #44522, #17663, #4073, #22075, #40084, #27091, #8802, #35952, #44823, #58399, #17961, #53978, #49853, #13517, #27387, #31511 ) ),
 .UNSPECIFIED., .F., .F., .F.,
 ( 4, 4 ),
 ( 4, 1, 1, 1, 1, 1, 1, 1, 1, 1, 1, 1, 1, 1, 1, 1, 1, 1, 1, 1, 1, 1, 1, 1, 1, 1, 1, 1, 1, 1, 1, 1, 4 ),
 ( -0.1331668876848000060, 1.133166887685000068 ),
 ( -0.02000000000000000042, 0.01250000000000000069, 0.04499999999999999833, 0.07749999999999999944, 0.1100000000000000006, 0.1424999999999999878, 0.1749999999999999889, 0.2074999999999999900, 0.2399999999999999911, 0.2725000000000000200, 0.3049999999999999933, 0.3375000000000000222, 0.3699999999999999956, 0.4025000000000000244, 0.4349999999999999978, 0.4675000000000000266, 0.5000000000000000000, 0.5324999999999999734, 0.5649999999999999467, 0.5975000000000000311, 0.6300000000000000044, 0.6624999999999999778, 0.6949999999999999512, 0.7275000000000000355, 0.7600000000000000089, 0.7924999999999999822, 0.8249999999999999556, 0.8575000000000000400, 0.8900000000000000133, 0.9224999999999999867, 0.9549999999999999600, 0.9875000000000000444, 1.020000000000000018 ),
 .UNSPECIFIED. ) ;
#17924=CARTESIAN_POINT ( 'NONE',  ( -2.899999999999999911, -80.69999999999998863, 0.000000000000000000 ) ) ;
#17945=CYLINDRICAL_SURFACE ( 'NONE', #16323, 1.250000000000000000 ) ;
#17950=CARTESIAN_POINT ( 'NONE',  ( -0.06678984038673288492, -80.97078420075510508, -1.509580312845645533 ) ) ;
#17961=CARTESIAN_POINT ( 'NONE',  ( 1.647188161489999914, -81.54038421936999725, 0.4319573417677999849 ) ) ;
#17965=CARTESIAN_POINT ( 'NONE',  ( 0.000000000000000000, -77.59999999938000315, 0.000000000000000000 ) ) ;
#17982=CARTESIAN_POINT ( 'NONE',  ( 0.2617232932829000047, -79.52639556175999758, -1.644907507304999905 ) ) ;
#17983=ADVANCED_FACE ( 'NONE', ( #13280 ), #53744, .F. ) ;
#17997=CARTESIAN_POINT ( 'NONE',  ( 1.543541483667999925, -79.04849869623998870, 0.5782440448787000697 ) ) ;
#18001=CARTESIAN_POINT ( 'NONE',  ( 0.03063463627522158145, -80.22746756300657012, -1.249376046788328809 ) ) ;
#18024=CARTESIAN_POINT ( 'NONE',  ( 0.4779442704572000045, -82.04270613248999666, -1.511941137165000004 ) ) ;
#18025=CARTESIAN_POINT ( 'NONE',  ( -0.4634070002434999558, -79.61543996570000559, -1.170148800580000037 ) ) ;
#18029=CARTESIAN_POINT ( 'NONE',  ( 0.7311670807272000472, -82.10923396026998944, 1.496881327486000002 ) ) ;
#18038=EDGE_CURVE ( 'NONE', #12786, #5620, #19260, .T. ) ;
#18055=CARTESIAN_POINT ( 'NONE',  ( -0.5000217545454540558, -81.50798104061337312, 1.145512068557146046 ) ) ;
#18059=CARTESIAN_POINT ( 'NONE',  ( -0.8598574106787247873, -81.42622421550363754, -1.245561739481349850 ) ) ;
#18090=CARTESIAN_POINT ( 'NONE',  ( -0.7004323366084000968, -78.35998666379998667, -1.469032877812000093 ) ) ;
#18093=CARTESIAN_POINT ( 'NONE',  ( 0.1636246173744697330, -78.13541666666664298, -1.249999999999999778 ) ) ;
#18128=CARTESIAN_POINT ( 'NONE',  ( -0.5713041596650000331, -79.30664044673999058, -1.442599867604999808 ) ) ;
#18129=CARTESIAN_POINT ( 'NONE',  ( -1.386642946985999769, -78.93602415856999244, 0.3678330367775999865 ) ) ;
#18131=CARTESIAN_POINT ( 'NONE',  ( -0.7940119350559891043, -83.16902664729457229, 1.287159878948278546 ) ) ;
#18136=CARTESIAN_POINT ( 'NONE',  ( 1.234706307098893063, -81.83799849444270080, -0.1953252668292917160 ) ) ;
#18147=CARTESIAN_POINT ( 'NONE',  ( 1.153231315078470320, -80.38161910157300838, 0.4820617830468132414 ) ) ;
#18162=CARTESIAN_POINT ( 'NONE',  ( -1.250000000000000000, -81.99999999999998579, 0.000000000000000000 ) ) ;
#18170=CARTESIAN_POINT ( 'NONE',  ( -1.172849536488999922, -80.03866583923000633, 0.6711148834816000885 ) ) ;
#18172=CARTESIAN_POINT ( 'NONE',  ( -0.9367133515736633109, -79.15782022828253162, -0.8274681181213610071 ) ) ;
#18211=DIRECTION ( 'NONE',  ( -1.000000000000000000, 0.000000000000000000, 0.000000000000000000 ) ) ;
#18214=CARTESIAN_POINT ( 'NONE',  ( -0.4635254915624000271, -77.75000000000000000, 1.426584774443000025 ) ) ;
#18225=CARTESIAN_POINT ( 'NONE',  ( -1.500000000000000000, -83.31666666666666288, 0.000000000000000000 ) ) ;
#18232=CARTESIAN_POINT ( 'NONE',  ( -0.9465222407332000154, -81.55663953507000485, -0.8164530897714000757 ) ) ;
#18252=CARTESIAN_POINT ( 'NONE',  ( 1.546185472753518253, -80.59627361124843503, -0.05127335055895310828 ) ) ;
#18260=DIRECTION ( 'NONE',  ( 0.000000000000000000, -1.000000000000000000, 0.000000000000000000 ) ) ;
#18283=ORIENTED_EDGE ( 'NONE', *, *, #54132, .T. ) ;
#18294=CARTESIAN_POINT ( 'NONE',  ( 0.0005663502821746999169, -77.83168747231999873, -1.534844259237000186 ) ) ;
#18297=CARTESIAN_POINT ( 'NONE',  ( 0.7037555052193149585, -77.85416666683801168, -1.219334037115995306 ) ) ;
#18321=CARTESIAN_POINT ( 'NONE',  ( -1.477496145247999992, -82.86377592892299049, 0.5756751103899000466 ) ) ;
#18334=AXIS2_PLACEMENT_3D ( 'NONE', #46582, #555, #9965 ) ;
#18349=CARTESIAN_POINT ( 'NONE',  ( -0.4892219813473719370, -81.50720965163131382, 1.150157418190592695 ) ) ;
#18351=CARTESIAN_POINT ( 'NONE',  ( 0.000000000000000000, -76.75499999999999545, 0.000000000000000000 ) ) ;
#18352=CARTESIAN_POINT ( 'NONE',  ( -0.6593618895071804431, -81.76024717370675887, 1.360737063013982118 ) ) ;
#18380=CARTESIAN_POINT ( 'NONE',  ( 1.328072050606999843, -78.47134980335999899, -0.9406846882429998891 ) ) ;
#18420=CARTESIAN_POINT ( 'NONE',  ( -1.542698325316999908, -81.18036382834999642, 0.6290719308543000210 ) ) ;
#18421=CARTESIAN_POINT ( 'NONE',  ( -1.502804487684999968, -79.37384159782000381, 0.3758151099642999537 ) ) ;
#18424=CARTESIAN_POINT ( 'NONE',  ( 0.04925444800588205801, -82.62245651653309153, 1.509272080436812935 ) ) ;
#18431=CARTESIAN_POINT ( 'NONE',  ( 0.7194808217321505550, -81.77430475710248459, -1.022317606335187756 ) ) ;
#18451=CARTESIAN_POINT ( 'NONE',  ( 2.899999999413999774, -80.69999999940999658, 1.301622050773000211E-09 ) ) ;
#18457=CARTESIAN_POINT ( 'NONE',  ( -0.4789091134304000463, -81.23884839998999041, -1.232458658897999992 ) ) ;
#18467=DIRECTION ( 'NONE',  ( 0.000000000000000000, -1.000000000000000000, 0.000000000000000000 ) ) ;
#18499=DIRECTION ( 'NONE',  ( -1.000000000000000000, 0.000000000000000000, 0.000000000000000000 ) ) ;
#18512=CARTESIAN_POINT ( 'NONE',  ( 1.244892399546890349, -82.84341106141995681, -0.1110735506749953583 ) ) ;
#18530=CARTESIAN_POINT ( 'NONE',  ( 0.000000000000000000, -80.79999999999999716, -3.000000000000982325 ) ) ;
#18538=CARTESIAN_POINT ( 'NONE',  ( -1.250013176831791695, -78.10006463709670754, 4.053087819277079897E-06 ) ) ;
#18543=CARTESIAN_POINT ( 'NONE',  ( -0.03896466140217625523, -78.47771600701551620, 1.249276069285430335 ) ) ;
#18552=CARTESIAN_POINT ( 'NONE',  ( -0.7427769915940999335, -81.79286360614999296, -1.400956470667000131 ) ) ;
#18577=CARTESIAN_POINT ( 'NONE',  ( 1.250000000000000000, -80.84999999999999432, 0.000000000000000000 ) ) ;
#18587=CARTESIAN_POINT ( 'NONE',  ( -0.6427777546026000044, -79.36308811491998938, -1.517687492048999998 ) ) ;
#18592=CARTESIAN_POINT ( 'NONE',  ( 0.6680158199250733064, -80.27032678700797419, -1.057154657451736091 ) ) ;
#18614=CARTESIAN_POINT ( 'NONE',  ( 1.308628125960000110, -82.16918203637000317, -0.6662886516973000051 ) ) ;
#18615=CARTESIAN_POINT ( 'NONE',  ( -0.5717664302369001028, -81.11020805664000477, -1.224358761826999986 ) ) ;
#18616=CARTESIAN_POINT ( 'NONE',  ( 0.1636246173744642929, -79.36458333333331439, 1.250000000000000888 ) ) ;
#18650=DIRECTION ( 'NONE',  ( -1.000000000000000000, 0.000000000000000000, -2.716802477432001181E-13 ) ) ;
#18675=CARTESIAN_POINT ( 'NONE',  ( 1.169626569868999821, -78.02236249102999466, 1.131652196797999999 ) ) ;
#18709=CARTESIAN_POINT ( 'NONE',  ( 1.587978134902999994, -80.54482878599999651, 0.5035716945827000135 ) ) ;
#18710=CARTESIAN_POINT ( 'NONE',  ( 1.088015599395999899, -79.22206712645999005, -0.7475960909009999877 ) ) ;
#18712=CARTESIAN_POINT ( 'NONE',  ( -1.226932303529735480, -82.19734641482862969, 0.9440816031200599534 ) ) ;
#18715=CARTESIAN_POINT ( 'NONE',  ( 1.244083471246176797, -79.84158205231473460, -0.1422760444506795119 ) ) ;
#18718=CARTESIAN_POINT ( 'NONE',  ( 0.5884030026776352340, -81.76430342800995277, -1.102917213597483848 ) ) ;
#18724=EDGE_LOOP ( 'NONE', ( #37437, #3726, #41416, #3978 ) ) ;
#18737=DIRECTION ( 'NONE',  ( 0.000000000000000000, -1.000000000000000000, 2.322499949178999976E-14 ) ) ;
#18745=CARTESIAN_POINT ( 'NONE',  ( -1.384313526018999818, -80.67041546398999685, -0.4900246725272000003 ) ) ;
#18824=CARTESIAN_POINT ( 'NONE',  ( -0.9577002445776288120, -83.04511862308959280, 0.8030944468889523735 ) ) ;
#18835=CARTESIAN_POINT ( 'NONE',  ( -0.3271848554490991434, -80.60416666666665719, -1.217465845835395299 ) ) ;
#18840=CARTESIAN_POINT ( 'NONE',  ( 0.7233469165846999616, -82.92988695178998171, -1.541617362406000113 ) ) ;
#18855=VECTOR ( 'NONE', #10453, 1000.000000000000000 ) ;
#18869=ORIENTED_EDGE ( 'NONE', *, *, #3610, .F. ) ;
#18873=CARTESIAN_POINT ( 'NONE',  ( 0.7435525986707999246, -78.04141375144000392, 1.342724626677000099 ) ) ;
#18874=EDGE_LOOP ( 'NONE', ( #13991, #44678, #6148, #14026 ) ) ;
#18876=CARTESIAN_POINT ( 'NONE',  ( -0.4665716294809927334, -80.19474127330990143, -1.159543645027278247 ) ) ;
#18877=CARTESIAN_POINT ( 'NONE',  ( 1.101185748242720974, -77.87369791681820175, -0.8451993228706300432 ) ) ;
#18879=CARTESIAN_POINT ( 'NONE',  ( 1.101723890961501473, -79.15951310949000685, 1.033017321146173506 ) ) ;
#18898=ORIENTED_EDGE ( 'NONE', *, *, #31409, .T. ) ;
#18899=CARTESIAN_POINT ( 'NONE',  ( -1.211920851286000023, -81.49548374185999933, -0.6339750518301998650 ) ) ;
#18900=CARTESIAN_POINT ( 'NONE',  ( -1.250231197918746817, -78.61063498648076120, -0.1636698104632014206 ) ) ;
#18902=CARTESIAN_POINT ( 'NONE',  ( 0.1636246173744642929, -82.86458333333334281, 1.250000000000000888 ) ) ;
#18927=CARTESIAN_POINT ( 'NONE',  ( -0.9038625163532321150, -81.53983264272325471, 0.8630782802490172267 ) ) ;
#18934=CARTESIAN_POINT ( 'NONE',  ( -0.06733317885808998149, -78.76457060935999266, -1.419816196976000144 ) ) ;
#18961=CARTESIAN_POINT ( 'NONE',  ( 1.623578234368999951, -78.02589724511999236, 0.1125035222880000074 ) ) ;
#19000=CARTESIAN_POINT ( 'NONE',  ( 0.1159286286506000102, -78.88797770777999574, 1.315005111595999976 ) ) ;
#19002=CARTESIAN_POINT ( 'NONE',  ( -0.2221408358902347280, -81.86333133491983460, -1.493708899689074387 ) ) ;
#19003=DIRECTION ( 'NONE',  ( 0.000000000000000000, 0.000000000000000000, -1.000000000000000000 ) ) ;
#19008=CARTESIAN_POINT ( 'NONE',  ( -0.2175832845984233821, -81.71159084714736309, -1.231031275339559583 ) ) ;
#19009=SHAPE_REPRESENTATION_RELATIONSHIP ( 'NONE' , 'NONE' ,  #33899, #34903 ) ;
#19027=ORIENTED_EDGE ( 'NONE', *, *, #51400, .T. ) ;
#19028=VERTEX_POINT ( 'NONE', #26935 ) ;
#19038=CARTESIAN_POINT ( 'NONE',  ( 1.447659443890000119, -80.92320979808999937, -0.6470525719642999940 ) ) ;
#19073=FACE_OUTER_BOUND ( 'NONE', #18874, .T. ) ;
#19092=VERTEX_POINT ( 'NONE', #32236 ) ;
#19114=CARTESIAN_POINT ( 'NONE',  ( -0.4786064949803862101, -83.00633325748620450, 1.154698265544586766 ) ) ;
#19121=CARTESIAN_POINT ( 'NONE',  ( -0.5884528863794137310, -79.75615526183086956, 1.392588485531083942 ) ) ;
#19157=AXIS2_PLACEMENT_3D ( 'NONE', #50358, #42074, #28473 ) ;
#19158=CARTESIAN_POINT ( 'NONE',  ( -1.067955516321597242, -80.55659099282243574, 0.6499150159960976891 ) ) ;
#19162=VERTEX_POINT ( 'NONE', #4743 ) ;
#19170=CARTESIAN_POINT ( 'NONE',  ( 1.350260416954781384, -77.89973958345846938, -0.1758964602772491170 ) ) ;
#19174=CARTESIAN_POINT ( 'NONE',  ( -0.6085898190276557429, -79.25767112076529486, 1.380970375365989433 ) ) ;
#19192=CARTESIAN_POINT ( 'NONE',  ( -1.186490757027999887, -81.53774735892999104, -0.2694786029208000033 ) ) ;
#19201=CARTESIAN_POINT ( 'NONE',  ( -0.6142531002814000107, -82.99257374592500014, 1.203711489715000305 ) ) ;
#19213=ORIENTED_EDGE ( 'NONE', *, *, #34452, .T. ) ;
#19219=CARTESIAN_POINT ( 'NONE',  ( -0.8865732340429423042, -81.53829647950151127, 0.8807237917444714626 ) ) ;
#19223=CARTESIAN_POINT ( 'NONE',  ( 1.249381860769000152, -78.80611706015999118, -0.3870755167071000535 ) ) ;
#19250=CARTESIAN_POINT ( 'NONE',  ( 1.621809933883000099, -78.52703137313999093, 0.1356303529659999840 ) ) ;
#19252=CARTESIAN_POINT ( 'NONE',  ( -0.9111626473548137817, -79.16027324500811346, -0.8557194560358774016 ) ) ;
#19260=B_SPLINE_CURVE_WITH_KNOTS ( 'NONE', 3,
 ( #22437, #12702, #52868, #14375, #45997, #30698, #40452, #39854, #30412, #5523, #53441, #48733, #17423, #8276, #23531, #9967, #44, #18824, #39572, #25986, #34838, #12423, #12983, #48447, #7988, #3563, #3848, #26279, #57870, #11429, #38275, #55715, #15558, #1126, #15263, #23822, #19405, #19114, #15848, #19997, #20281, #24118, #55121, #51874, #37696, #29409, #28826, #50715, #28536, #10256, #11147, #37105, #42136, #33837, #2285, #37983, #37397, #33255, #29122, #51004, #47462, #56007, #10853, #1703, #19697, #46584, #51297, #46875, #6986, #47168, #46289, #6699, #24708, #24419, #6110, #42433, #42720, #56295, #6402, #2002, #33550, #14665, #41544, #51589, #55414, #32662, #10553, #28238, #5816, #41840, #1415, #14962, #32959, #25565, #57153, #56873, #43585, #7852, #16718, #3148, #30565, #17004 ),
 .UNSPECIFIED., .F., .F.,
 ( 4, 2, 2, 2, 1, 1, 1, 2, 2, 2, 2, 2, 1, 1, 1, 2, 2, 2, 2, 2, 1, 1, 1, 2, 2, 2, 2, 2, 2, 2, 2, 1, 2, 2, 2, 2, 1, 1, 2, 2, 2, 2, 2, 2, 2, 2, 2, 1, 2, 2, 2, 2, 1, 1, 1, 2, 2, 2, 4 ),
 ( 0.000000000000000000, 0.06250000000008198997, 0.09375000000012330414, 0.1093750000001438710, 0.1171875000001541683, 0.1210937500001593031, 0.1230468750001619399, 0.1240234375001631334, 0.1250000000001643130, 0.1875000000002498834, 0.2187500000002923772, 0.2343750000003131384, 0.2421875000003240463, 0.2460937500003289036, 0.2480468750003312906, 0.2490234375003324285, 0.2500000000003335665, 0.3125000000004117262, 0.3437500000004511391, 0.3593750000004708456, 0.3671875000004808376, 0.3710937500004856116, 0.3730468750004848344, 0.3740234375004842238, 0.3750000000004836131, 0.4375000000004443668, 0.4687500000004250489, 0.5000000000004057865, 0.5312500000003864686, 0.5468750000003772538, 0.5546875000003725908, 0.5585937500003702594, 0.5605468750003689271, 0.5625000000003675948, 0.5937500000003431699, 0.6093750000003311795, 0.6171875000003249623, 0.6210937500003218537, 0.6230468750003202993, 0.6250000000003187450, 0.6875000000002745582, 0.7187500000002521316, 0.7343750000002409184, 0.7421875000002361444, 0.7500000000002312595, 0.7812500000002134959, 0.7968750000002042810, 0.8046875000001999512, 0.8085937500001977307, 0.8125000000001955103, 0.8437500000001791900, 0.8593750000001713074, 0.8671875000001671996, 0.8710937500001649791, 0.8730468750001639799, 0.8740234375001629807, 0.8750000000001620926, 0.9375000000000810463, 1.000000000000000000 ),
 .UNSPECIFIED. ) ;
#19262=CARTESIAN_POINT ( 'NONE',  ( -1.605277969432999940, -80.85709877522999989, -0.5682425234610001263 ) ) ;
#19275=VERTEX_POINT ( 'NONE', #41460 ) ;
#19285=CARTESIAN_POINT ( 'NONE',  ( -1.250000000000000000, -81.09999999999999432, 0.000000000000000000 ) ) ;
#19291=CARTESIAN_POINT ( 'NONE',  ( 0.6544915521845998674, -81.17247804586000370, 1.531959166345999934 ) ) ;
#19294=CARTESIAN_POINT ( 'NONE',  ( -1.501968397107060316, -81.74187130586206251, 0.1553300411971603456 ) ) ;
#19306=CARTESIAN_POINT ( 'NONE',  ( 0.000000000000000000, -80.74999999950000529, -2.949999999500999781 ) ) ;
#19313=CARTESIAN_POINT ( 'NONE',  ( -1.287598599762399321, -77.77604166675226338, -0.7431007365616121296 ) ) ;
#19323=CARTESIAN_POINT ( 'NONE',  ( -1.250000000000001332, -81.48958333333334281, 0.1636246173744632659 ) ) ;
#19330=CARTESIAN_POINT ( 'NONE',  ( 0.2122939316688999822, -79.21759604279999678, -1.334248387208000208 ) ) ;
#19355=EDGE_CURVE ( 'NONE', #32332, #26523, #46674, .T. ) ;
#19376=B_SPLINE_SURFACE_WITH_KNOTS ( 'NONE', 3, 3, ( 
 ( #15993, #1271, #42865, #19546, #47020, #37254, #37544, #24850, #20141, #38420, #19262, #55561, #37841, #33981, #46435, #19847, #15412, #32811, #2423, #1555, #33405, #47310, #2139, #10403, #52018, #15700, #29262, #10995, #51443, #6550, #28978, #56151, #24559, #28388, #42576 ),
 ( #55266, #33694, #11572, #23967, #6839, #51733, #14814, #29552, #47607, #23680, #5964, #41986, #33107, #25709, #57874, #17431, #3288, #35416, #52874, #16572, #39001, #56731, #25992, #52304, #25424, #16862, #39288, #25132, #43736, #48176, #57010, #21281, #39577, #16290, #52589 ),
 ( #53446, #29837, #12139, #57300, #34269, #8282, #43439, #30127, #30702, #44016, #11860, #26284, #57580, #53160, #12427, #34843, #48452, #30420, #3568, #7995, #47889, #7708, #12709, #12990, #30987, #3853, #38710, #21572, #7420, #7131, #2999, #20996, #43157, #39860, #34557 ),
 ( #17142, #2714, #20711, #35128, #48738, #44298, #21851, #36017, #58167, #18615, #44592, #31574, #23326, #9750, #49026, #27446, #44891, #17733, #49, #36892, #49621, #26863, #35720, #36604, #9168, #4442, #917, #41044, #27736, #54044, #8869, #54627, #14164, #18025, #31278 ) ),
 .UNSPECIFIED., .F., .F., .F.,
 ( 4, 4 ),
 ( 4, 1, 1, 1, 1, 1, 1, 1, 1, 1, 1, 1, 1, 1, 1, 1, 1, 1, 1, 1, 1, 1, 1, 1, 1, 1, 1, 1, 1, 1, 1, 1, 4 ),
 ( -0.1331668876848000060, 1.133166887685000068 ),
 ( -0.02000000000000000042, 0.01250000000000000069, 0.04499999999999999833, 0.07749999999999999944, 0.1100000000000000006, 0.1424999999999999878, 0.1749999999999999889, 0.2074999999999999900, 0.2399999999999999911, 0.2725000000000000200, 0.3049999999999999933, 0.3375000000000000222, 0.3699999999999999956, 0.4025000000000000244, 0.4349999999999999978, 0.4675000000000000266, 0.5000000000000000000, 0.5324999999999999734, 0.5649999999999999467, 0.5975000000000000311, 0.6300000000000000044, 0.6624999999999999778, 0.6949999999999999512, 0.7275000000000000355, 0.7600000000000000089, 0.7924999999999999822, 0.8249999999999999556, 0.8575000000000000400, 0.8900000000000000133, 0.9224999999999999867, 0.9549999999999999600, 0.9875000000000000444, 1.020000000000000018 ),
 .UNSPECIFIED. ) ;
#19385=CARTESIAN_POINT ( 'NONE',  ( 1.231359744498104147, -82.83660106426310676, -0.2141053253869658335 ) ) ;
#19389=CARTESIAN_POINT ( 'NONE',  ( -0.5296483783707884863, -79.34647407982620848, -1.412499042453858600 ) ) ;
#19390=LINE ( 'NONE', #46275, #11437 ) ;
#19399=DIRECTION ( 'NONE',  ( -1.000000000000000000, 0.000000000000000000, 0.000000000000000000 ) ) ;
#19405=CARTESIAN_POINT ( 'NONE',  ( -0.4788566569365060865, -83.00635035241097626, 1.154595247919521173 ) ) ;
#19417=CARTESIAN_POINT ( 'NONE',  ( -1.092232985442822102, -80.54166666666664298, -0.6295237254636245616 ) ) ;
#19432=CARTESIAN_POINT ( 'NONE',  ( 0.3958579896396000608, -81.53291524179999783, -1.618315812554999900 ) ) ;
#19453=EDGE_LOOP ( 'NONE', ( #50435, #19594, #5354, #55829, #57189, #44334, #53427, #45849, #46058, #17860 ) ) ;
#19458=CARTESIAN_POINT ( 'NONE',  ( -0.3738612770365654647, -80.20118014076501822, -1.192774224883461187 ) ) ;
#19462=CARTESIAN_POINT ( 'NONE',  ( 1.459619044399156129, -79.07920200935929245, -0.3821340575799183625 ) ) ;
#19481=CARTESIAN_POINT ( 'NONE',  ( -0.1636246173744726473, -78.88541666666664298, 1.249999999999999112 ) ) ;
#19505=CARTESIAN_POINT ( 'NONE',  ( 0.8823246602996009935, -81.41312424128729219, 0.8850044837457081703 ) ) ;
#19518=AXIS2_PLACEMENT_3D ( 'NONE', #17388, #43976, #48983 ) ;
#19539=CARTESIAN_POINT ( 'NONE',  ( 1.341343219651000229, -79.09091657910998663, -0.9216622887798999741 ) ) ;
#19546=CARTESIAN_POINT ( 'NONE',  ( -1.576937714420000081, -81.29921328099999300, 0.6430338560479000876 ) ) ;
#19566=AXIS2_PLACEMENT_3D ( 'NONE', #51184, #19580, #19003 ) ;
#19576=CARTESIAN_POINT ( 'NONE',  ( -0.5713041596650000331, -79.36585677060999444, -1.442599867604999808 ) ) ;
#19577=CARTESIAN_POINT ( 'NONE',  ( 0.1536065772846999800, -77.82239276298000163, 1.313283405909000168 ) ) ;
#19579=CARTESIAN_POINT ( 'NONE',  ( 1.188464411453045155, -82.05564304759461436, 0.9880997565357596546 ) ) ;
#19580=DIRECTION ( 'NONE',  ( 0.000000000000000000, -1.000000000000000000, 0.000000000000000000 ) ) ;
#19582=CARTESIAN_POINT ( 'NONE',  ( 1.222194407272268135, -79.83372676383018529, -0.2630658939555856612 ) ) ;
#19585=CARTESIAN_POINT ( 'NONE',  ( -0.8804009821880611764, -81.66335410272444051, -0.8868692789278864730 ) ) ;
#19588=DIRECTION ( 'NONE',  ( 0.000000000000000000, -0.7071067811866525998, -0.7071067811864425456 ) ) ;
#19593=ADVANCED_FACE ( 'NONE', ( #34465 ), #7328, .T. ) ;
#19594=ORIENTED_EDGE ( 'NONE', *, *, #52535, .F. ) ;
#19597=DIRECTION ( 'NONE',  ( 1.000000000000000000, 0.000000000000000000, 0.000000000000000000 ) ) ;
#19616=CARTESIAN_POINT ( 'NONE',  ( -0.5581707956298000983, -81.04937075464998486, 1.358247929972999701 ) ) ;
#19635=CARTESIAN_POINT ( 'NONE',  ( 0.7419868901144667239, -78.42466652974195540, 1.005884453515640597 ) ) ;
#19645=CARTESIAN_POINT ( 'NONE',  ( -0.5982973345652318198, -82.01490259020367546, 1.110242726331215790 ) ) ;
#19653=FACE_OUTER_BOUND ( 'NONE', #30244, .T. ) ;
#19658=CARTESIAN_POINT ( 'NONE',  ( 0.6291625305437360538, -78.26672467768266017, -1.091960772762393006 ) ) ;
#19673=ORIENTED_EDGE ( 'NONE', *, *, #33087, .T. ) ;
#19674=CARTESIAN_POINT ( 'NONE',  ( -1.218920058826058916, -79.58278420342887216, 0.2778685722280217485 ) ) ;
#19675=CARTESIAN_POINT ( 'NONE',  ( 1.378196749914432973, -78.03568483536376732, 0.6686781945394131288 ) ) ;
#19690=B_SPLINE_CURVE_WITH_KNOTS ( 'NONE', 3,
 ( #27958, #50140, #45418, #1715, #37117, #50726, #14103, #36539, #41555, #14387, #18835, #28247, #22967, #46301, #19417, #37407, #55428, #40977 ),
 .UNSPECIFIED., .F., .F.,
 ( 4, 2, 2, 2, 2, 2, 2, 2, 4 ),
 ( 0.000000000000000000, 0.1250000000000000833, 0.2500000000000001110, 0.3750000000000000000, 0.4999999999999999445, 0.6249999999999998890, 0.7499999999999997780, 0.8749999999999998890, 1.000000000000000000 ),
 .UNSPECIFIED. ) ;
#19696=VECTOR ( 'NONE', #46205, 1000.000000000000114 ) ;
#19697=CARTESIAN_POINT ( 'NONE',  ( 0.4701836139821906069, -82.94435837239699083, 1.158166872552657045 ) ) ;
#19713=ORIENTED_EDGE ( 'NONE', *, *, #38085, .T. ) ;
#19715=EDGE_CURVE ( 'NONE', #31102, #15817, #48765, .T. ) ;
#19735=CARTESIAN_POINT ( 'NONE',  ( 0.01020306644930230565, -80.72629856499307266, -1.249600794397132564 ) ) ;
#19744=CARTESIAN_POINT ( 'NONE',  ( -1.092042939088145648, -80.55956894660957346, 0.6086570842360274902 ) ) ;
#19754=CARTESIAN_POINT ( 'NONE',  ( -0.8249880669573600445, -80.16805825303950428, -0.9389422545057994896 ) ) ;
#19758=CARTESIAN_POINT ( 'NONE',  ( -1.275548104907354485, -78.30286137473437691, 0.8563608086819030074 ) ) ;
#19773=CARTESIAN_POINT ( 'NONE',  ( 0.6721823118158000154, -81.85354343447998815, 1.172239651246999914 ) ) ;
#19777=CARTESIAN_POINT ( 'NONE',  ( 0.7681833999686413783, -78.82291666666668561, 0.9995835529977274980 ) ) ;
#19785=CARTESIAN_POINT ( 'NONE',  ( -1.266615395500999997, -82.10834473437999748, -0.4708042714212999913 ) ) ;
#19803=CARTESIAN_POINT ( 'NONE',  ( 0.8303084959499684725, -81.41757219168246706, 0.9342352573978692787 ) ) ;
#19808=B_SPLINE_CURVE_WITH_KNOTS ( 'NONE', 3,
 ( #11101, #28491, #46832, #24375, #14333, #46245, #23780, #27906, #28786, #55372, #24666, #10213, #45952, #42674, #1087, #38233, #32330, #23489 ),
 .UNSPECIFIED., .F., .F.,
 ( 4, 2, 2, 2, 2, 2, 2, 2, 4 ),
 ( 0.000000000000000000, 0.1250000000000000833, 0.2500000000000001110, 0.3750000000000000000, 0.4999999999999999445, 0.6249999999999998890, 0.7499999999999997780, 0.8749999999999998890, 1.000000000000000000 ),
 .UNSPECIFIED. ) ;
#19810=CARTESIAN_POINT ( 'NONE',  ( -0.9836304129562999377, -79.07916002803999334, 1.026102791697000027 ) ) ;
#19814=VERTEX_POINT ( 'NONE', #49824 ) ;
#19835=DIRECTION ( 'NONE',  ( 1.000000000000000000, 0.000000000000000000, 0.000000000000000000 ) ) ;
#19836=CARTESIAN_POINT ( 'NONE',  ( -0.7004323366084000968, -78.47841931153999440, -1.469032877812000093 ) ) ;
#19847=CARTESIAN_POINT ( 'NONE',  ( 1.505228744355000092, -80.54130269966999833, -0.7963060858757999849 ) ) ;
#19862=EDGE_CURVE ( 'NONE', #26523, #3682, #149, .T. ) ;
#19872=CARTESIAN_POINT ( 'NONE',  ( -0.4360978520027915528, -80.00346707738961527, 1.172260374082638945 ) ) ;
#19877=CARTESIAN_POINT ( 'NONE',  ( -0.9131908197385000259, -81.40406183460000022, -1.254418330386999791 ) ) ;
#19878=CARTESIAN_POINT ( 'NONE',  ( -1.186038146469999832, -79.55615654513999857, -0.5797594326791000174 ) ) ;
#19880=CARTESIAN_POINT ( 'NONE',  ( 1.023096227096927491, -81.93418301853687069, -1.110676516153182414 ) ) ;
#19881=CARTESIAN_POINT ( 'NONE',  ( -1.215509798056741531, -83.29877716300683232, 0.8975879569896133559 ) ) ;
#19883=CARTESIAN_POINT ( 'NONE',  ( -0.3277658534251963740, -80.99651576041503631, 1.218475390182661711 ) ) ;
#19885=CARTESIAN_POINT ( 'NONE',  ( -0.4528890155571457798, -81.69566638204462095, -1.164992333293775051 ) ) ;
#19889=EDGE_LOOP ( 'NONE', ( #8596, #36656, #16402, #54349 ) ) ;
#19906=CIRCLE ( 'NONE', #22753, 3.000000000000000000 ) ;
#19914=CARTESIAN_POINT ( 'NONE',  ( -0.5839839591423000575, -79.36543996570000559, -1.474617623361999863 ) ) ;
#19919=CARTESIAN_POINT ( 'NONE',  ( 1.290219381540931742, -79.54546911372847262, 0.8289380708588135471 ) ) ;
#19933=CARTESIAN_POINT ( 'NONE',  ( 0.7167766847591896529, -78.42666800608485289, 1.023989290741913694 ) ) ;
#19957=VERTEX_POINT ( 'NONE', #38777 ) ;
#19962=EDGE_LOOP ( 'NONE', ( #45309, #14644, #16189, #12466 ) ) ;
#19973=CARTESIAN_POINT ( 'NONE',  ( 0.4636642495210216430, -82.75527458966378447, -1.160904140311521227 ) ) ;
#19978=CARTESIAN_POINT ( 'NONE',  ( -1.260816076409378761, -78.29616218522681947, -0.8268161317517029874 ) ) ;
#19985=CARTESIAN_POINT ( 'NONE',  ( -1.487911162517577823, -81.33517288243102428, 0.2674502543427375034 ) ) ;
#19995=AXIS2_PLACEMENT_3D ( 'NONE', #34154, #56331, #32995 ) ;
#19997=CARTESIAN_POINT ( 'NONE',  ( -0.4803308748150663110, -83.00644942323957309, 1.153985611485086160 ) ) ;
#20022=CARTESIAN_POINT ( 'NONE',  ( -1.462746796095000024, -81.34738048770999796, -0.3322225316158000097 ) ) ;
#20042=CARTESIAN_POINT ( 'NONE',  ( 0.8513071080735492568, -80.41589136472569521, 0.9149315643236480833 ) ) ;
#20043=EDGE_CURVE ( 'NONE', #26509, #16529, #48026, .T. ) ;
#20049=ORIENTED_EDGE ( 'NONE', *, *, #37762, .T. ) ;
#20053=CONICAL_SURFACE ( 'NONE', #19157, 10.04999999996000071, 0.7853981633972997312 ) ;
#20059=CARTESIAN_POINT ( 'NONE',  ( -0.4698087411539742519, -78.74903415325783840, 1.463278444719919635 ) ) ;
#20069=CARTESIAN_POINT ( 'NONE',  ( -1.289397738844999974, -81.47443067016000384, -0.2928510814055000355 ) ) ;
#20073=CARTESIAN_POINT ( 'NONE',  ( -0.3271848554491046945, -82.89583333333328596, 1.217465845835393301 ) ) ;
#20079=CARTESIAN_POINT ( 'NONE',  ( 1.242145130744999992, -82.29782237970999859, -0.5320213307544999770 ) ) ;
#20081=ORIENTED_EDGE ( 'NONE', *, *, #21743, .T. ) ;
#20091=AXIS2_PLACEMENT_3D ( 'NONE', #32459, #23621, #23336 ) ;
#20098=CARTESIAN_POINT ( 'NONE',  ( 0.05551074714531987336, -81.47208037662812785, 1.249630598122650982 ) ) ;
#20102=CARTESIAN_POINT ( 'NONE',  ( 1.331074987945999988, -78.92186531869998589, 0.4986494974128999336 ) ) ;
#20104=CARTESIAN_POINT ( 'NONE',  ( 0.7681833999686413783, -78.32291666666668561, 0.9995835529977274980 ) ) ;
#20131=CARTESIAN_POINT ( 'NONE',  ( 0.4326115402657000342, -79.03523500932999468, -1.568920109259999807 ) ) ;
#20141=CARTESIAN_POINT ( 'NONE',  ( 0.5947595261268000533, -80.98341720544999589, -1.595643580583000043 ) ) ;
#20166=CARTESIAN_POINT ( 'NONE',  ( -1.171857579988537124, -80.07201495124374446, 0.4348164940204689022 ) ) ;
#20173=CARTESIAN_POINT ( 'NONE',  ( 0.7681090888009013407, -78.92317030813214274, 0.9998401714662717987 ) ) ;
#20174=CARTESIAN_POINT ( 'NONE',  ( -1.511181634424322739, -81.85134434412550775, -0.03904378459183766026 ) ) ;
#20179=CARTESIAN_POINT ( 'NONE',  ( -0.8831554397796215206, -81.66311148394188990, -0.8841190442798870786 ) ) ;
#20181=CARTESIAN_POINT ( 'NONE',  ( 9.500000000000000000, -87.20000000000000284, 0.000000000000000000 ) ) ;
#20205=CARTESIAN_POINT ( 'NONE',  ( -0.9103895169571000201, -79.34438689399999589, -1.233764334031000054 ) ) ;
#20226=CARTESIAN_POINT ( 'NONE',  ( 1.159297299441395701, -78.38080567615219252, 0.4674996523628443534 ) ) ;
#20236=CARTESIAN_POINT ( 'NONE',  ( -1.124740126079791569, -82.06431169942482029, 0.5547021489710047826 ) ) ;
#20237=CARTESIAN_POINT ( 'NONE',  ( 0.4286008670186999825, -79.47756961838999246, -1.472170099309999980 ) ) ;
#20246=AXIS2_PLACEMENT_3D ( 'NONE', #2245, #30525, #42676 ) ;
#20259=CARTESIAN_POINT ( 'NONE',  ( 0.7170858719455162067, -82.77394172231353764, -1.023701603912586133 ) ) ;
#20261=ORIENTED_EDGE ( 'NONE', *, *, #54132, .F. ) ;
#20265=CARTESIAN_POINT ( 'NONE',  ( -1.304299203641290150, -78.79190939947621075, -0.7577321730552538659 ) ) ;
#20271=CARTESIAN_POINT ( 'NONE',  ( 1.180475833332838898, -81.15297854159264546, 0.9435589873242250514 ) ) ;
#20281=CARTESIAN_POINT ( 'NONE',  ( -0.3505635783453250331, -82.99769806729025845, 1.207601184449180964 ) ) ;
#20319=AXIS2_PLACEMENT_3D ( 'NONE', #16772, #26766, #40362 ) ;
#20321=CARTESIAN_POINT ( 'NONE',  ( -0.4793197146253041496, -80.50639153267658799, 1.154396842167616954 ) ) ;
#20327=EDGE_LOOP ( 'NONE', ( #28807, #10219, #12647 ) ) ;
#20335=CARTESIAN_POINT ( 'NONE',  ( 0.1335152958906870024, -77.98161697419730842, -1.503794547195192788 ) ) ;
#20349=VERTEX_POINT ( 'NONE', #44257 ) ;
#20350=CARTESIAN_POINT ( 'NONE',  ( -0.8896385144511894660, -81.17505783692462273, 1.220758139846876977 ) ) ;
#20356=ADVANCED_FACE ( 'NONE', ( #12947 ), #3811, .F. ) ;
#20380=CARTESIAN_POINT ( 'NONE',  ( -0.02778611078446202240, -81.47725253223261177, 1.249451979124360346 ) ) ;
#20425=CARTESIAN_POINT ( 'NONE',  ( 1.647188161489999914, -81.60043415305999304, 0.4319573417677999849 ) ) ;
#20434=CARTESIAN_POINT ( 'NONE',  ( 0.4376773866434802152, -81.25363771554175685, -1.170757306240687301 ) ) ;
#20446=CARTESIAN_POINT ( 'NONE',  ( -0.5487783150233148666, -79.44506368774518990, -1.407050603238668041 ) ) ;
#20453=CARTESIAN_POINT ( 'NONE',  ( -0.5576869831189765758, -80.01218415722107125, 1.118859008776958763 ) ) ;
#20463=CARTESIAN_POINT ( 'NONE',  ( 1.023842844794183415, -82.03353868496313339, -1.111437593429350557 ) ) ;
#20465=CARTESIAN_POINT ( 'NONE',  ( -1.249633652174288123, -81.09028336531811476, 0.1639779393582905531 ) ) ;
#20481=ORIENTED_EDGE ( 'NONE', *, *, #43456, .F. ) ;
#20489=CARTESIAN_POINT ( 'NONE',  ( -1.217465845835396188, -79.97916666666667140, 0.3271848554490955907 ) ) ;
#20492=CARTESIAN_POINT ( 'NONE',  ( -1.605277969432999940, -80.79704884152999966, -0.5682425234610001263 ) ) ;
#20512=CARTESIAN_POINT ( 'NONE',  ( 1.178220910110199249, -78.37735903784117397, 0.4169870122232715581 ) ) ;
#20531=PLANE ( 'NONE',  #24758 ) ;
#20547=CARTESIAN_POINT ( 'NONE',  ( 0.02044864296007851273, -82.72696752574205448, -1.249602587815580979 ) ) ;
#20551=CARTESIAN_POINT ( 'NONE',  ( 1.250000000000000000, -79.34999999999999432, 0.000000000000000000 ) ) ;
#20552=CARTESIAN_POINT ( 'NONE',  ( 0.3438320055965143895, -78.89273934135498223, -1.494433517359873287 ) ) ;
#20559=CARTESIAN_POINT ( 'NONE',  ( -1.506676414812727183, -81.35541669807993514, -0.1142558127726139849 ) ) ;
#20571=CARTESIAN_POINT ( 'NONE',  ( -0.7681833999686477066, -80.42708333333334281, 0.9995835529977223910 ) ) ;
#20593=CARTESIAN_POINT ( 'NONE',  ( 0.5021253177900999454, -82.03818896268001026, -1.588436081161999969 ) ) ;
#20602=CARTESIAN_POINT ( 'NONE',  ( 0.03580840776424319000, -80.72793405598493166, -1.249249415733939994 ) ) ;
#20608=CARTESIAN_POINT ( 'NONE',  ( -0.8876925766968319920, -80.53848003073616724, 0.8795304379308518383 ) ) ;
#20623=DIRECTION ( 'NONE',  ( -1.000000000000000000, 0.000000000000000000, 0.000000000000000000 ) ) ;
#20635=CARTESIAN_POINT ( 'NONE',  ( 1.500158885365614037, -79.99082255360691818, -0.1727759592422631052 ) ) ;
#20636=EDGE_CURVE ( 'NONE', #32917, #23434, #4318, .T. ) ;
#20646=CARTESIAN_POINT ( 'NONE',  ( -0.6675286376147999690, -83.05589043469399257, 1.308112063971999861 ) ) ;
#20665=CARTESIAN_POINT ( 'NONE',  ( 0.7780701227561770406, -81.42184096910574453, 0.9786064938539484892 ) ) ;
#20668=CARTESIAN_POINT ( 'NONE',  ( 1.250000000000000000, -82.34999999999999432, 0.000000000000000000 ) ) ;
#20672=B_SPLINE_CURVE_WITH_KNOTS ( 'NONE', 3,
 ( #35911, #53944, #18225, #13478 ),
 .UNSPECIFIED., .F., .F.,
 ( 4, 4 ),
 ( 0.000000000000000000, 1.000000000000000000 ),
 .UNSPECIFIED. ) ;
#20690=CARTESIAN_POINT ( 'NONE',  ( 1.249999999999999778, -81.26041666666667140, 0.1636246173744711763 ) ) ;
#20691=ORIENTED_EDGE ( 'NONE', *, *, #15907, .F. ) ;
#20701=CARTESIAN_POINT ( 'NONE',  ( -0.5563122350442734065, -81.58886627922497325, -1.147641270936760716 ) ) ;
#20702=CARTESIAN_POINT ( 'NONE',  ( -1.462188802161999979, -79.42500599778999515, -0.7147474581103999691 ) ) ;
#20709=CARTESIAN_POINT ( 'NONE',  ( -1.405367936307999832, -81.36885036431999652, -0.7351702954167999016 ) ) ;
#20711=CARTESIAN_POINT ( 'NONE',  ( -1.240843214692000096, -81.55232256240998368, -0.5344114414419000036 ) ) ;
#20715=CARTESIAN_POINT ( 'NONE',  ( 0.7076411874954000591, -82.87108743283400258, -1.508144869335000138 ) ) ;
#20719=CARTESIAN_POINT ( 'NONE',  ( -0.6953472622417047333, -81.17859467677989471, -1.050534455880961060 ) ) ;
#20746=CARTESIAN_POINT ( 'NONE',  ( -1.528577347423822896, -82.33719591969246210, 0.2446291273937655775 ) ) ;
#20747=CARTESIAN_POINT ( 'NONE',  ( 0.5145317771005305518, -79.75915092270044227, -1.139023839920036529 ) ) ;
#20748=ADVANCED_FACE ( 'NONE', ( #32271 ), #8686, .T. ) ;
#20773=CARTESIAN_POINT ( 'NONE',  ( 0.7681833999686413783, -79.82291666666668561, 0.9995835529977274980 ) ) ;
#20775=CARTESIAN_POINT ( 'NONE',  ( -0.8549356769920000154, -79.78634392611000692, -1.335470596990000036 ) ) ;
#20777=CARTESIAN_POINT ( 'NONE',  ( 1.021232999834709165, -79.43413075375887900, -1.113201301497944717 ) ) ;
#20791=CARTESIAN_POINT ( 'NONE',  ( 0.8550973397286725231, -78.41513696957164825, 0.9116979360512381669 ) ) ;
#20804=CARTESIAN_POINT ( 'NONE',  ( 0.4193126674068999860, -78.47530136235999976, -1.609880760976999836 ) ) ;
#20813=CARTESIAN_POINT ( 'NONE',  ( 1.249999999999999778, -81.76041666666665719, 0.1636246173744711763 ) ) ;
#20817=AXIS2_PLACEMENT_3D ( 'NONE', #282, #18260, #54275 ) ;
#20818=VERTEX_POINT ( 'NONE', #22851 ) ;
#20823=EDGE_CURVE ( 'NONE', #54925, #19957, #13396, .T. ) ;
#20827=CARTESIAN_POINT ( 'NONE',  ( 0.4179219924009388576, -82.75223496485374142, -1.178037307492067365 ) ) ;
#20831=CARTESIAN_POINT ( 'NONE',  ( 0.8643672385586788076, -79.07759423480628413, 1.266515284944065511 ) ) ;
#20861=EDGE_CURVE ( 'NONE', #48338, #15598, #38824, .T. ) ;
#20863=PRESENTATION_STYLE_ASSIGNMENT (( #42733 ) ) ;
#20887=CARTESIAN_POINT ( 'NONE',  ( -0.4467308992050549321, -80.50409186563182118, 1.167926343017146484 ) ) ;
#20919=CARTESIAN_POINT ( 'NONE',  ( 1.248378436199009789, -80.95238111698088801, -0.8512954593689909810 ) ) ;
#20923=ADVANCED_FACE ( 'NONE', ( #46188 ), #37881, .F. ) ;
#20929=CARTESIAN_POINT ( 'NONE',  ( -1.260823269212999920, -83.24552555368300943, -0.6699510868867000202 ) ) ;
#20932=CARTESIAN_POINT ( 'NONE',  ( -0.3271848554490991434, -82.10416666666665719, -1.217465845835395299 ) ) ;
#20942=EDGE_CURVE ( 'NONE', #50158, #29213, #9864, .T. ) ;
#20945=CARTESIAN_POINT ( 'NONE',  ( 0.000000000000000000, -77.70312499986998489, 0.000000000000000000 ) ) ;
#20947=CARTESIAN_POINT ( 'NONE',  ( 0.3704480504712000521, -79.97245295876999194, -1.624200486671999899 ) ) ;
#20950=DIRECTION ( 'NONE',  ( 0.000000000000000000, 0.000000000000000000, -1.000000000000000000 ) ) ;
#20964=B_SPLINE_CURVE_WITH_KNOTS ( 'NONE', 3,
 ( #20668, #56397, #38667, #2101, #46981, #38090, #6509, #43392, #25377, #56112, #30080, #2951, #24809, #48131, #15948, #7663, #47564, #24519 ),
 .UNSPECIFIED., .F., .F.,
 ( 4, 2, 2, 2, 2, 2, 2, 2, 4 ),
 ( 0.000000000000000000, 0.1250000000000000555, 0.2500000000000001110, 0.3750000000000001110, 0.5000000000000001110, 0.6250000000000000000, 0.7500000000000000000, 0.8750000000000000000, 1.000000000000000000 ),
 .UNSPECIFIED. ) ;
#20980=CARTESIAN_POINT ( 'NONE',  ( -1.499999999971000086, -77.75000000002998490, -1.761798912373000190E-09 ) ) ;
#20991=VECTOR ( 'NONE', #55849, 1000.000000000000000 ) ;
#20995=CARTESIAN_POINT ( 'NONE',  ( 0.6196687357644999894, -82.48466316460299197, -1.586136063883000213 ) ) ;
#20996=CARTESIAN_POINT ( 'NONE',  ( 1.195983586496999873, -79.65738863544999049, -0.8522763136304999376 ) ) ;
#21004=CARTESIAN_POINT ( 'NONE',  ( -0.4230197004537654126, -81.19773207085326305, -1.184957207720425343 ) ) ;
#21009=DIRECTION ( 'NONE',  ( -1.000000000000000000, 0.000000000000000000, 0.000000000000000000 ) ) ;
#21013=CARTESIAN_POINT ( 'NONE',  ( 0.5021253177900999454, -81.97897263881000640, -1.588436081161999969 ) ) ;
#21023=CARTESIAN_POINT ( 'NONE',  ( -1.159815416435145519, -80.06983562126566767, 0.4658135504333426047 ) ) ;
#21030=CARTESIAN_POINT ( 'NONE',  ( 0.9049231439593581339, -83.02548565174980411, -1.211648235339166657 ) ) ;
#21032=CARTESIAN_POINT ( 'NONE',  ( 0.1863217586117132951, -79.73704994264652157, -1.236983196908801208 ) ) ;
#21040=EDGE_CURVE ( 'NONE', #28137, #50285, #43129, .T. ) ;
#21050=ORIENTED_EDGE ( 'NONE', *, *, #42314, .T. ) ;
#21051=VERTEX_POINT ( 'NONE', #20181 ) ;
#21061=CARTESIAN_POINT ( 'NONE',  ( -0.5415696896749999656, -80.67073041130998945, 1.614471809804999936 ) ) ;
#21095=CARTESIAN_POINT ( 'NONE',  ( 1.250000000000000000, -81.84999999999999432, 0.000000000000000000 ) ) ;
#21101=DIRECTION ( 'NONE',  ( 0.000000000000000000, -1.000000000000000000, 0.000000000000000000 ) ) ;
#21104=CARTESIAN_POINT ( 'NONE',  ( 0.7681833999686413783, -81.82291666666667140, 0.9995835529977274980 ) ) ;
#21117=CARTESIAN_POINT ( 'NONE',  ( 0.1997943094379295570, -82.73830915514584206, -1.234411186249315673 ) ) ;
#21163=DIRECTION ( 'NONE',  ( 0.000000000000000000, -1.000000000000000000, 0.000000000000000000 ) ) ;
#21176=CARTESIAN_POINT ( 'NONE',  ( 0.7505680871121789277, -80.42410011460410146, 1.001643424464033760 ) ) ;
#21184=VECTOR ( 'NONE', #49667, 1000.000000000000000 ) ;
#21191=CARTESIAN_POINT ( 'NONE',  ( 0.000000000000000000, -76.75499999999999545, 0.000000000000000000 ) ) ;
#21192=CARTESIAN_POINT ( 'NONE',  ( 0.6217590130341388299, -78.00838734090868343, -1.375229810813027198 ) ) ;
#21202=CARTESIAN_POINT ( 'NONE',  ( -1.497746365902677956, -80.73982606612976554, 0.1936102584281759742 ) ) ;
#21211=CARTESIAN_POINT ( 'NONE',  ( 0.6000739755967000599, -82.55077418747099216, 1.467756090344000119 ) ) ;
#21235=CARTESIAN_POINT ( 'NONE',  ( 0.2617232932829000047, -79.46717923788999371, -1.644907507304999905 ) ) ;
#21247=CARTESIAN_POINT ( 'NONE',  ( 0.2826255412215000207, -78.50241276046999417, 1.393030722100999874 ) ) ;
#21255=DIRECTION ( 'NONE',  ( 0.000000000000000000, 1.000000000000000000, 0.000000000000000000 ) ) ;
#21272=CARTESIAN_POINT ( 'NONE',  ( -1.160437014136601830, -79.13041490960291924, -0.4645391383290830012 ) ) ;
#21281=CARTESIAN_POINT ( 'NONE',  ( 1.291435174072999903, -79.59407194668000329, -0.9202965842325999679 ) ) ;
#21313=CARTESIAN_POINT ( 'NONE',  ( -1.193682973855900498, -81.90195388324707437, -0.9265664831431897897 ) ) ;
#21314=CARTESIAN_POINT ( 'NONE',  ( 0.2287542621979772872, -79.73975884029870542, -1.229773590461207267 ) ) ;
#21366=EDGE_CURVE ( 'NONE', #15598, #43389, #8909, .T. ) ;
#21378=CARTESIAN_POINT ( 'NONE',  ( -0.07104694739953303084, -81.98010065232054444, 1.247827375486972645 ) ) ;
#21411=CIRCLE ( 'NONE', #49712, 9.950000000000001066 ) ;
#21483=CARTESIAN_POINT ( 'NONE',  ( 0.9109609374202407572, -78.02623425204966168, -1.202808138275179184 ) ) ;
#21494=CARTESIAN_POINT ( 'NONE',  ( -0.6295237254636235624, -78.58333333333331439, -1.092232985442822990 ) ) ;
#21495=CARTESIAN_POINT ( 'NONE',  ( -1.091678962010041332, -80.91005275380919670, -1.044836448518165595 ) ) ;
#21504=CARTESIAN_POINT ( 'NONE',  ( 1.307088170492999968, -81.35043415305999304, 0.3427697847655999941 ) ) ;
#21523=CARTESIAN_POINT ( 'NONE',  ( -1.603789611582999930, -80.41062457329998381, -0.4506860216877000558 ) ) ;
#21524=EDGE_LOOP ( 'NONE', ( #2108, #43138, #57427, #47556 ) ) ;
#21538=CARTESIAN_POINT ( 'NONE',  ( -1.375956693795999941, -77.66350764398998763, -0.3562251950211999807 ) ) ;
#21571=CARTESIAN_POINT ( 'NONE',  ( -1.491081270832000039, -81.78991179838999415, 0.8224925373206000145 ) ) ;
#21572=CARTESIAN_POINT ( 'NONE',  ( -1.223477145616999939, -79.91002549588999671, 0.8121269926547999285 ) ) ;
#21576=CARTESIAN_POINT ( 'NONE',  ( -1.510823314100999903, -83.28820597566100048, -0.3534059060544000319 ) ) ;
#21597=CARTESIAN_POINT ( 'NONE',  ( 0.3859961575645005083, -79.95043709814795818, 1.188828431463626822 ) ) ;
#21608=ORIENTED_EDGE ( 'NONE', *, *, #26417, .F. ) ;
#21666=CARTESIAN_POINT ( 'NONE',  ( 0.6719893610791689564, -81.92997134543871596, 1.053977402048356549 ) ) ;
#21667=CARTESIAN_POINT ( 'NONE',  ( 1.264115560106999991, -78.59429962090999311, -0.8953837640199000525 ) ) ;
#21672=EDGE_CURVE ( 'NONE', #57688, #57178, #56692, .T. ) ;
#21675=ORIENTED_EDGE ( 'NONE', *, *, #6996, .F. ) ;
#21677=CARTESIAN_POINT ( 'NONE',  ( -1.092232985442824100, -81.95833333333330017, 0.6295237254636200097 ) ) ;
#21685=ORIENTED_EDGE ( 'NONE', *, *, #3610, .T. ) ;
#21718=ORIENTED_EDGE ( 'NONE', *, *, #45175, .F. ) ;
#21743=EDGE_CURVE ( 'NONE', #19957, #57178, #7261, .T. ) ;
#21752=CARTESIAN_POINT ( 'NONE',  ( 0.000000000000000000, -77.69999999999998863, 0.000000000000000000 ) ) ;
#21772=CARTESIAN_POINT ( 'NONE',  ( 1.250000000000000000, -83.24999999999998579, 0.000000000000000000 ) ) ;
#21777=CARTESIAN_POINT ( 'NONE',  ( -0.1636246173744726473, -80.88541666666665719, 1.249999999999999112 ) ) ;
#21778=CARTESIAN_POINT ( 'NONE',  ( -1.417852237051780540, -79.87761815572260105, -0.5262009856692363430 ) ) ;
#21781=LINE ( 'NONE', #22069, #50261 ) ;
#21788=CARTESIAN_POINT ( 'NONE',  ( -0.6004489902433000070, -82.23482063826000399, -1.340115349862999850 ) ) ;
#21827=CARTESIAN_POINT ( 'NONE',  ( 0.5801429252975863760, -80.26374239380967879, -1.107237889240993534 ) ) ;
#21850=CARTESIAN_POINT ( 'NONE',  ( -1.339567984323000172, -82.99025183280099327, -0.6016691479808000675 ) ) ;
#21851=CARTESIAN_POINT ( 'NONE',  ( 1.258195058187999926, -81.29968570196999167, 0.4928692076250000276 ) ) ;
#21856=CARTESIAN_POINT ( 'NONE',  ( -1.510823314100999903, -83.22898965179099662, -0.3534059060544000319 ) ) ;
#21865=ORIENTED_EDGE ( 'NONE', *, *, #5001, .T. ) ;
#21870=CARTESIAN_POINT ( 'NONE',  ( 1.431241028886999889, -81.47764180916999521, -0.8524881072380000591 ) ) ;
#21875=CARTESIAN_POINT ( 'NONE',  ( 0.5928849308894093006, -77.96093750004841638, 1.162612760383189947 ) ) ;
#21878=CARTESIAN_POINT ( 'NONE',  ( 1.150057798432680745, -79.88230094492989508, 0.4893180354286167377 ) ) ;
#21903=CARTESIAN_POINT ( 'NONE',  ( -0.3229108565016139409, -79.49587948166266926, 1.210510340675584162 ) ) ;
#21935=DIRECTION ( 'NONE',  ( 0.000000000000000000, -1.000000000000000000, 0.000000000000000000 ) ) ;
#21944=DIRECTION ( 'NONE',  ( 0.000000000000000000, 0.000000000000000000, -1.000000000000000000 ) ) ;
#21949=CARTESIAN_POINT ( 'NONE',  ( 0.6503206246681177971, -81.93155565340288149, 1.067516121945689900 ) ) ;
#21950=CARTESIAN_POINT ( 'NONE',  ( 0.1140339002500000004, -79.26247845825999150, 1.544894080918999713 ) ) ;
#21976=ORIENTED_EDGE ( 'NONE', *, *, #58164, .F. ) ;
#22059=CARTESIAN_POINT ( 'NONE',  ( 1.217465845835393967, -83.27083333333331439, 0.3271848554491025851 ) ) ;
#22066=CARTESIAN_POINT ( 'NONE',  ( -0.4440249787718509311, -80.74810222861310649, 1.446726180314430010 ) ) ;
#22067=CARTESIAN_POINT ( 'NONE',  ( -0.7735775726147171572, -78.52788082791856539, 0.9939198430596817291 ) ) ;
#22069=CARTESIAN_POINT ( 'NONE',  ( 1.250000000000000000, -80.25000000000000000, 0.000000000000000000 ) ) ;
#22075=CARTESIAN_POINT ( 'NONE',  ( 1.517511648408000013, -81.98249872513999037, -0.7726417995267998995 ) ) ;
#22089=DIRECTION ( 'NONE',  ( 1.000000000000000000, 0.000000000000000000, 0.000000000000000000 ) ) ;
#22090=CYLINDRICAL_SURFACE ( 'NONE', #27831, 1.250000000000000000 ) ;
#22093=B_SPLINE_CURVE_WITH_KNOTS ( 'NONE', 3,
 ( #38153, #56175, #8595, #22169, #54357, #21875, #40768, #3589, #362, #49639 ),
 .UNSPECIFIED., .F., .F.,
 ( 4, 2, 2, 2, 4 ),
 ( 0.000000000000000000, 0.2500000000000000000, 0.5000000000000000000, 0.7500000000000000000, 1.000000000000000000 ),
 .UNSPECIFIED. ) ;
#22096=CONICAL_SURFACE ( 'NONE', #4202, 2.399999999383999771, 0.7853981633972997312 ) ;
#22113=CARTESIAN_POINT ( 'NONE',  ( 0.06588118243728999235, -79.39804249476999587, -1.568452433177999872 ) ) ;
#22118=CARTESIAN_POINT ( 'NONE',  ( 0.2449793097989906576, -80.24093316106807094, -1.227248574985329688 ) ) ;
#22145=CARTESIAN_POINT ( 'NONE',  ( -0.7427769915940999335, -81.97954691737999156, -1.400956470667000131 ) ) ;
#22147=CARTESIAN_POINT ( 'NONE',  ( -1.250000000000000000, -78.60000000000000853, 0.000000000000000000 ) ) ;
#22159=CARTESIAN_POINT ( 'NONE',  ( -1.250000000000000000, -79.51887984502333495, -0.2965639121358008001 ) ) ;
#22164=CARTESIAN_POINT ( 'NONE',  ( 0.3958579896396000608, -81.41448259405999011, -1.618315812554999900 ) ) ;
#22169=CARTESIAN_POINT ( 'NONE',  ( 1.075291064028265797, -77.93750000007800338, 0.7806521200495090129 ) ) ;
#22172=CARTESIAN_POINT ( 'NONE',  ( 1.120846582852062401, -79.88692784018829229, 0.5535639178212069522 ) ) ;
#22177=CARTESIAN_POINT ( 'NONE',  ( 0.6451515509158406436, -81.68939381893659402, 1.369045774478446553 ) ) ;
#22199=CARTESIAN_POINT ( 'NONE',  ( 0.9981636088842267274, -79.40219188384969584, 0.7561152057269426852 ) ) ;
#22210=EDGE_CURVE ( 'NONE', #19028, #43389, #29609, .T. ) ;
#22247=CARTESIAN_POINT ( 'NONE',  ( 0.5893919561240600347, -81.93594225748110205, 1.102503278612346316 ) ) ;
#22248=CARTESIAN_POINT ( 'NONE',  ( -0.7373102530955000233, -77.91848566455999503, -1.491280593247999997 ) ) ;
#22250=CARTESIAN_POINT ( 'NONE',  ( -1.355824619571554868, -82.71355153832641349, 0.6688378176153790822 ) ) ;
#22255=CARTESIAN_POINT ( 'NONE',  ( 0.4857358544503080355, -81.75688173250232182, -1.151682746447475036 ) ) ;
#22258=CARTESIAN_POINT ( 'NONE',  ( 1.217465845835394855, -80.22916666666665719, -0.3271848554490981997 ) ) ;
#22287=CARTESIAN_POINT ( 'NONE',  ( -0.5136231202413000796, -80.98605406588998790, 1.249846006485000105 ) ) ;
#22331=AXIS2_PLACEMENT_3D ( 'NONE', #5231, #36514, #45691 ) ;
#22335=ORIENTED_EDGE ( 'NONE', *, *, #48851, .T. ) ;
#22368=CARTESIAN_POINT ( 'NONE',  ( -1.511213184804566678, -80.84932130686019036, -0.0005575924518816717133 ) ) ;
#22371=CONICAL_SURFACE ( 'NONE', #19566, 2.399999999383999771, 0.7853981633972997312 ) ;
#22397=CARTESIAN_POINT ( 'NONE',  ( -0.8906226101088000613, -79.46323634664999247, -1.206976125017999779 ) ) ;
#22413=CARTESIAN_POINT ( 'NONE',  ( -0.2078880262912795873, -79.31385681300682222, -1.400979628114630060 ) ) ;
#22414=CARTESIAN_POINT ( 'NONE',  ( -1.640079623176999846, -78.26202514954999856, 0.1643931535720999926 ) ) ;
#22417=AXIS2_PLACEMENT_3D ( 'NONE', #56161, #15710, #47321 ) ;
#22418=CARTESIAN_POINT ( 'NONE',  ( 0.7058627945297136774, -80.27327360843820259, -1.031809627508295302 ) ) ;
#22437=CARTESIAN_POINT ( 'NONE',  ( -1.250000000000000000, -83.09999999999999432, 0.000000000000000000 ) ) ;
#22441=VERTEX_POINT ( 'NONE', #15513 ) ;
#22442=CARTESIAN_POINT ( 'NONE',  ( 1.424157265477999923, -83.17957200447399657, 0.6972603243668999973 ) ) ;
#22447=CARTESIAN_POINT ( 'NONE',  ( -0.6811744818814000624, -82.36187082071000987, -1.520282978132999840 ) ) ;
#22467=CARTESIAN_POINT ( 'NONE',  ( 0.9312054229806641104, -79.90880812854101123, 0.8360461126382245922 ) ) ;
#22475=CARTESIAN_POINT ( 'NONE',  ( 0.08826574687577952438, -81.71975954240951978, 1.508524260310913689 ) ) ;
#22484=ORIENTED_EDGE ( 'NONE', *, *, #13739, .F. ) ;
#22489=VERTEX_POINT ( 'NONE', #33508 ) ;
#22494=CARTESIAN_POINT ( 'NONE',  ( 0.9057247795391590861, -82.41316108956780795, 0.9056628583376803432 ) ) ;
#22513=EDGE_CURVE ( 'NONE', #50534, #54581, #19808, .T. ) ;
#22543=AXIS2_PLACEMENT_3D ( 'NONE', #3282, #34263, #7987 ) ;
#22548=CARTESIAN_POINT ( 'NONE',  ( -0.7048934085577001074, -80.86062486154999362, -1.509431780672999990 ) ) ;
#22549=CARTESIAN_POINT ( 'NONE',  ( 0.3813430617698000402, -79.10306886790999670, -1.382988530009999995 ) ) ;
#22551=CARTESIAN_POINT ( 'NONE',  ( -0.5530976515504120172, -82.84513323647280458, -1.407674718852016227 ) ) ;
#22552=DIRECTION ( 'NONE',  ( -1.000000000000000000, 0.000000000000000000, 0.000000000000000000 ) ) ;
#22567=ORIENTED_EDGE ( 'NONE', *, *, #7090, .F. ) ;
#22591=AXIS2_PLACEMENT_3D ( 'NONE', #54069, #13605, #49052 ) ;
#22596=CARTESIAN_POINT ( 'NONE',  ( -1.250000000000000000, -82.49999999999998579, 0.000000000000000000 ) ) ;
#22611=B_SPLINE_CURVE_WITH_KNOTS ( 'NONE', 3,
 ( #49934, #27170, #9478, #1220, #23628, #32466, #49343, #935, #41640, #31889 ),
 .UNSPECIFIED., .F., .F.,
 ( 4, 2, 2, 2, 4 ),
 ( 0.000000000000000000, 0.2500000000000000555, 0.5000000000000001110, 0.7500000000000002220, 1.000000000000000000 ),
 .UNSPECIFIED. ) ;
#22630=DIRECTION ( 'NONE',  ( -1.000000000000000000, 0.000000000000000000, 0.000000000000000000 ) ) ;
#22662=CARTESIAN_POINT ( 'NONE',  ( -0.006417454803627380307, -79.62467248096164951, -1.262730415849851573 ) ) ;
#22667=CARTESIAN_POINT ( 'NONE',  ( -1.250000000000000000, -80.99999999999998579, 0.000000000000000000 ) ) ;
#22669=CARTESIAN_POINT ( 'NONE',  ( 0.9951084243826858744, -81.03151564770095661, -1.137131669208984786 ) ) ;
#22679=CARTESIAN_POINT ( 'NONE',  ( 1.503815466746999840, -81.98234125147999407, 0.5029271919957000181 ) ) ;
#22711=CARTESIAN_POINT ( 'NONE',  ( 1.595957623597000108, -77.99986730064999563, -0.4120752205041999794 ) ) ;
#22715=CARTESIAN_POINT ( 'NONE',  ( 0.8949709245464939622, -80.28907454115488918, -0.8721969588273668084 ) ) ;
#22737=CARTESIAN_POINT ( 'NONE',  ( -0.4275916205537000359, -81.79006927205000466, 1.526944760756999919 ) ) ;
#22738=CARTESIAN_POINT ( 'NONE',  ( -0.6532870389514158216, -78.68357565247356433, -1.115868458321769952 ) ) ;
#22740=CARTESIAN_POINT ( 'NONE',  ( -1.250000000000001332, -78.98958333333331439, 0.1636246173744632659 ) ) ;
#22753=AXIS2_PLACEMENT_3D ( 'NONE', #46408, #4779, #9794 ) ;
#22765=CARTESIAN_POINT ( 'NONE',  ( -0.9386777138244112306, -81.54303105412684261, 0.8252884126292686640 ) ) ;
#22769=CARTESIAN_POINT ( 'NONE',  ( 1.412381594861192191, -81.62866237199072827, 0.5432125840743284861 ) ) ;
#22775=EDGE_CURVE ( 'NONE', #12955, #41153, #673, .T. ) ;
#22801=CARTESIAN_POINT ( 'NONE',  ( 1.136899222205000060, -79.08384707092999122, 1.164526648744999893 ) ) ;
#22824=CARTESIAN_POINT ( 'NONE',  ( 0.000000000000000000, -76.75499999999999545, 0.000000000000000000 ) ) ;
#22837=CARTESIAN_POINT ( 'NONE',  ( -0.5298108134926000634, -80.61193089235000286, 1.579417458585999912 ) ) ;
#22838=CARTESIAN_POINT ( 'NONE',  ( 1.543707792073999885, -78.64998119068999927, 0.1290987484668000007 ) ) ;
#22846=CARTESIAN_POINT ( 'NONE',  ( 1.060064467237852970, -81.80564032585678547, -0.6624441280364113949 ) ) ;
#22851=CARTESIAN_POINT ( 'NONE',  ( -0.4635254915624000271, -77.75000000000000000, 1.426584774443000025 ) ) ;
#22852=EDGE_LOOP ( 'NONE', ( #26973, #48913, #16256, #43083 ) ) ;
#22873=EDGE_CURVE ( 'NONE', #50534, #5620, #1888, .T. ) ;
#22877=CARTESIAN_POINT ( 'NONE',  ( 1.195983586496999873, -79.34407194668000329, -0.8522763136304999376 ) ) ;
#22926=ORIENTED_EDGE ( 'NONE', *, *, #5485, .T. ) ;
#22943=VECTOR ( 'NONE', #58116, 1000.000000000000000 ) ;
#22952=DIRECTION ( 'NONE',  ( 0.000000000000000000, 1.000000000000000000, 0.000000000000000000 ) ) ;
#22954=CARTESIAN_POINT ( 'NONE',  ( 1.250000000000000000, -79.75000000000000000, 0.000000000000000000 ) ) ;
#22958=CARTESIAN_POINT ( 'NONE',  ( 3.425937024882473377E-06, -77.82827182887865547, -1.422119424801547627 ) ) ;
#22964=CARTESIAN_POINT ( 'NONE',  ( -0.1240015960471890777, -78.48315057415604201, 1.244361994668307769 ) ) ;
#22967=CARTESIAN_POINT ( 'NONE',  ( -0.7681833999686432657, -80.57291666666668561, -0.9995835529977258327 ) ) ;
#22972=CARTESIAN_POINT ( 'NONE',  ( -0.4275916205537000359, -81.60338596081999185, 1.526944760756999919 ) ) ;
#22976=ADVANCED_FACE ( 'NONE', ( #23714 ), #22371, .T. ) ;
#23004=CARTESIAN_POINT ( 'NONE',  ( -0.1733946080540000045, -79.15336183579998419, 1.639152535173999947 ) ) ;
#23008=CARTESIAN_POINT ( 'NONE',  ( 1.148914256626027530, -80.31786800289191319, -0.4925239578509333360 ) ) ;
#23028=CARTESIAN_POINT ( 'NONE',  ( 1.413069887183999951, -82.10586534759998756, -0.7194652256120001033 ) ) ;
#23029=CARTESIAN_POINT ( 'NONE',  ( -0.3271710452716786732, -78.70441584275798164, -1.250829328336668045 ) ) ;
#23030=CARTESIAN_POINT ( 'NONE',  ( -0.6295237254636286695, -79.41666666666665719, 1.092232985442819881 ) ) ;
#23088=CARTESIAN_POINT ( 'NONE',  ( -0.6580604922749000441, -79.36225491982999358, -1.488334326434000099 ) ) ;
#23091=EDGE_CURVE ( 'NONE', #12208, #28137, #16136, .T. ) ;
#23092=VECTOR ( 'NONE', #47094, 1000.000000000000000 ) ;
#23129=CARTESIAN_POINT ( 'NONE',  ( -1.570423240223999928, -80.79746564644000273, -0.5559045111934000083 ) ) ;
#23130=CARTESIAN_POINT ( 'NONE',  ( -0.5681478814570000146, -78.60956985887999338, -1.191589642135999938 ) ) ;
#23133=CARTESIAN_POINT ( 'NONE',  ( -1.320760026772257456, -83.20951332364732878, 0.7341362115397076504 ) ) ;
#23139=CARTESIAN_POINT ( 'NONE',  ( 1.249949556334875034, -81.84594067282965568, -0.07348289510804084657 ) ) ;
#23140=DIRECTION ( 'NONE',  ( 1.000000000000000000, 0.000000000000000000, 0.000000000000000000 ) ) ;
#23146=CARTESIAN_POINT ( 'NONE',  ( -0.9224894341409000109, -78.71213903957999491, -1.081399571158999873 ) ) ;
#23167=CARTESIAN_POINT ( 'NONE',  ( 0.6650966107743999656, -80.48093781866000995, 1.309234371339000225 ) ) ;
#23171=B_SPLINE_CURVE_WITH_KNOTS ( 'NONE', 3,
 ( #737, #31685, #23139, #18136, #54447, #41146, #44405, #5140, #57983, #31094, #36133, #45000, #4556, #13098, #54149, #49433, #8983, #22846, #39970, #35830, #17540, #12813, #9275, #26968, #27263, #35531, #50022, #44704, #450, #36420, #18431, #53559, #27552, #18718, #36713, #30811, #48843, #4258, #22255, #40269, #50896, #10746, #41730, #6003, #46475, #10440, #6298, #37585, #28133, #24310, #42614, #15151, #55603, #29022, #42324, #11039, #19008, #37292, #9861, #37000, #1893, #24600, #19885, #46184, #42027, #47060, #55308, #14854, #1309, #32849, #1595, #2178, #37878, #1026, #55899, #15453, #33145, #14563, #19585, #20179, #24008, #14270, #51190, #28721, #27843, #33444, #46774, #32557, #51481, #23719, #6590, #28427, #32268, #54726, #50313, #45888, #5421, #23430 ),
 .UNSPECIFIED., .F., .F.,
 ( 4, 2, 2, 2, 1, 1, 2, 2, 2, 1, 1, 1, 2, 2, 2, 2, 2, 2, 2, 2, 1, 1, 1, 2, 2, 2, 2, 2, 1, 1, 1, 2, 2, 2, 2, 2, 1, 1, 1, 2, 2, 2, 2, 2, 1, 1, 1, 2, 2, 2, 2, 2, 1, 1, 1, 2, 2, 2, 4 ),
 ( 0.000000000000000000, 0.06250000000005537237, 0.09375000000008305856, 0.1093750000000968947, 0.1171875000001040279, 0.1210937500001075945, 0.1230468750001091766, 0.1250000000001107725, 0.1562500000001333378, 0.1718750000001446621, 0.1796875000001502964, 0.1835937500001527667, 0.1855468750001543765, 0.1875000000001559586, 0.2187500000001829925, 0.2343750000001968703, 0.2500000000002107203, 0.3125000000002646772, 0.3437500000002917111, 0.3593750000003052003, 0.3671875000003119727, 0.3710937500003154699, 0.3730468750003171352, 0.3740234375003181899, 0.3750000000003193001, 0.4375000000002924883, 0.4687500000002794431, 0.4843750000002731704, 0.4921875000002697842, 0.4960937500002681744, 0.4980468750002673417, 0.4990234375002667311, 0.5000000000002661205, 0.5625000000002297051, 0.5937500000002110534, 0.6093750000002020606, 0.6171875000001972866, 0.6210937500001948441, 0.6230468750001939560, 0.6240234375001935119, 0.6250000000001929568, 0.6875000000001660894, 0.7187500000001526557, 0.7343750000001459943, 0.7421875000001429967, 0.7460937500001416645, 0.7480468750001411093, 0.7490234375001408873, 0.7500000000001406653, 0.8125000000000772715, 0.8437500000000451861, 0.8593750000000291989, 0.8671875000000212053, 0.8710937500000168754, 0.8730468750000147660, 0.8740234375000135447, 0.8750000000000122125, 0.9375000000000061062, 1.000000000000000000 ),
 .UNSPECIFIED. ) ;
#23184=CARTESIAN_POINT ( 'NONE',  ( -1.092232985442822102, -79.04166666666662877, -0.6295237254636245616 ) ) ;
#23196=FACE_BOUND ( 'NONE', #25881, .T. ) ;
#23226=CARTESIAN_POINT ( 'NONE',  ( 0.8837568277754281887, -82.78815962236846815, -0.8834506328319239321 ) ) ;
#23263=CARTESIAN_POINT ( 'NONE',  ( -1.553390134080000040, -82.80356852156999992, -0.6977077157647000316 ) ) ;
#23288=ORIENTED_EDGE ( 'NONE', *, *, #13626, .F. ) ;
#23289=CARTESIAN_POINT ( 'NONE',  ( -1.180289549356538625, -80.57346338427628041, 0.4123096908613480549 ) ) ;
#23295=CARTESIAN_POINT ( 'NONE',  ( -1.250000000000000000, -82.99999999999998579, 0.000000000000000000 ) ) ;
#23296=CARTESIAN_POINT ( 'NONE',  ( -1.338663453569000072, -79.24733985637000444, -0.7509245179382000313 ) ) ;
#23306=CARTESIAN_POINT ( 'NONE',  ( 1.149457566070329673, -79.04350818708034865, -0.9787974342808838379 ) ) ;
#23308=ORIENTED_EDGE ( 'NONE', *, *, #41033, .T. ) ;
#23325=CARTESIAN_POINT ( 'NONE',  ( 1.250322495222000008, -82.80093166112899894, 0.5125084194436000384 ) ) ;
#23326=CARTESIAN_POINT ( 'NONE',  ( -0.4297501350614000293, -80.92073041130998945, 1.281126864269000132 ) ) ;
#23328=CARTESIAN_POINT ( 'NONE',  ( 1.249999999999999778, -82.76041666666665719, 0.1636246173744711763 ) ) ;
#23336=DIRECTION ( 'NONE',  ( -1.000000000000000000, 0.000000000000000000, 0.000000000000000000 ) ) ;
#23384=CARTESIAN_POINT ( 'NONE',  ( -1.578837173282999995, -79.25089178026999548, 0.3948290484592000271 ) ) ;
#23420=CARTESIAN_POINT ( 'NONE',  ( 1.472546342128999930, -80.42245324701998754, -0.7790162248558000213 ) ) ;
#23421=CARTESIAN_POINT ( 'NONE',  ( 0.3144971358097000125, -78.16411730064999119, -1.282096067459000066 ) ) ;
#23423=CARTESIAN_POINT ( 'NONE',  ( -0.9781074130570392988, -81.68114129133320489, 1.150371876388886383 ) ) ;
#23425=FACE_OUTER_BOUND ( 'NONE', #33453, .T. ) ;
#23426=CARTESIAN_POINT ( 'NONE',  ( 1.163576041378186599, -79.82060005907925415, -0.4561830117966773623 ) ) ;
#23427=AXIS2_PLACEMENT_3D ( 'NONE', #47880, #12130, #30118 ) ;
#23430=CARTESIAN_POINT ( 'NONE',  ( -1.250000000000000000, -81.59999999999999432, 0.000000000000000000 ) ) ;
#23434=VERTEX_POINT ( 'NONE', #6043 ) ;
#23435=EDGE_CURVE ( 'NONE', #27512, #7116, #21411, .T. ) ;
#23440=CARTESIAN_POINT ( 'NONE',  ( 0.000000000000000000, -87.20000000000000284, 0.000000000000000000 ) ) ;
#23449=CARTESIAN_POINT ( 'NONE',  ( 0.9995835529977233902, -81.30208333333334281, 0.7681833999686461523 ) ) ;
#23455=CARTESIAN_POINT ( 'NONE',  ( -0.8692139286044998636, -81.28111201704999189, -1.194008811194000153 ) ) ;
#23464=LINE ( 'NONE', #22596, #52356 ) ;
#23468=CARTESIAN_POINT ( 'NONE',  ( -1.249999999999999778, -79.01041666666665719, -0.1636246173744686228 ) ) ;
#23484=CARTESIAN_POINT ( 'NONE',  ( 0.000000000000000000, -80.69999999999998863, 0.000000000000000000 ) ) ;
#23489=CARTESIAN_POINT ( 'NONE',  ( -1.250000000000000000, -82.49999999999998579, 0.000000000000000000 ) ) ;
#23497=CARTESIAN_POINT ( 'NONE',  ( -1.250000000000000000, -81.99999999999998579, 0.000000000000000000 ) ) ;
#23513=ORIENTED_EDGE ( 'NONE', *, *, #50912, .T. ) ;
#23516=AXIS2_PLACEMENT_3D ( 'NONE', #13084, #49718, #21944 ) ;
#23531=CARTESIAN_POINT ( 'NONE',  ( -1.108406828139037570, -83.06136306326980900, 0.5900032945368707260 ) ) ;
#23536=DIRECTION ( 'NONE',  ( -1.000000000000000000, 0.000000000000000000, 0.000000000000000000 ) ) ;
#23537=CARTESIAN_POINT ( 'NONE',  ( -1.388062938059625884, -79.81688670877672109, 0.5997038735736672788 ) ) ;
#23548=EDGE_CURVE ( 'NONE', #15743, #14217, #19690, .T. ) ;
#23575=CARTESIAN_POINT ( 'NONE',  ( -1.239753235927716357, -80.59053486374234865, 0.1581211216746350179 ) ) ;
#23586=CARTESIAN_POINT ( 'NONE',  ( -0.4122473303297303215, -80.19853687741431258, -1.179911485936611770 ) ) ;
#23590=CARTESIAN_POINT ( 'NONE',  ( -0.2871694602881026959, -79.23982420962433082, 1.481336007913308883 ) ) ;
#23607=CARTESIAN_POINT ( 'NONE',  ( -1.486838331013629722, -81.23578785145382142, 0.2672933875640012280 ) ) ;
#23616=FACE_OUTER_BOUND ( 'NONE', #5997, .T. ) ;
#23621=DIRECTION ( 'NONE',  ( 0.000000000000000000, -1.000000000000000000, 0.000000000000000000 ) ) ;
#23628=CARTESIAN_POINT ( 'NONE',  ( 0.9521775314477300967, -79.29341203308139541, -0.8298931526774534495 ) ) ;
#23642=CARTESIAN_POINT ( 'NONE',  ( 0.3375844306956000129, -79.28888630715999852, -1.278415048790000119 ) ) ;
#23670=CARTESIAN_POINT ( 'NONE',  ( 0.1198033158700999995, -79.13952864070999738, 1.623056241665000066 ) ) ;
#23680=CARTESIAN_POINT ( 'NONE',  ( -0.6709475781581999421, -80.98357467910000196, -1.436741477991000160 ) ) ;
#23705=EDGE_CURVE ( 'NONE', #41153, #9574, #16665, .T. ) ;
#23710=CARTESIAN_POINT ( 'NONE',  ( -1.630114970985000022, -79.72770188080998821, -0.3434887894992000312 ) ) ;
#23711=CARTESIAN_POINT ( 'NONE',  ( 1.313811648119000086, -79.27774869623999621, 0.1287517855103000042 ) ) ;
#23713=CARTESIAN_POINT ( 'NONE',  ( 0.8719698933019950360, -81.92406134944869223, -1.233151496242500533 ) ) ;
#23714=FACE_OUTER_BOUND ( 'NONE', #28623, .T. ) ;
#23716=CARTESIAN_POINT ( 'NONE',  ( 1.156157754792947578, -79.81928919401691758, -0.4747237588690541021 ) ) ;
#23719=CARTESIAN_POINT ( 'NONE',  ( -1.149810464072230198, -81.63223063354799081, -0.4900990545918544883 ) ) ;
#23731=CARTESIAN_POINT ( 'NONE',  ( -1.499999999971000086, -77.75000000002998490, -1.761798912373000190E-09 ) ) ;
#23746=CARTESIAN_POINT ( 'NONE',  ( -0.5042965048037999498, -80.60741372253998804, 1.503356827960000031 ) ) ;
#23766=VECTOR ( 'NONE', #2195, 1000.000000000000114 ) ;
#23780=CARTESIAN_POINT ( 'NONE',  ( 0.6295237254636258939, -82.66666666666667140, -1.092232985442821658 ) ) ;
#23799=CARTESIAN_POINT ( 'NONE',  ( 1.216162773206594938, -82.83133620506080774, -0.2928064032228187008 ) ) ;
#23822=CARTESIAN_POINT ( 'NONE',  ( -0.4796248374066554576, -83.00640320879189460, 1.154279267341133952 ) ) ;
#23847=CARTESIAN_POINT ( 'NONE',  ( 1.611423453808999984, -81.65923367201999383, 0.4225784326546000447 ) ) ;
#23878=CARTESIAN_POINT ( 'NONE',  ( 1.197231442357009623, -77.88020833347827931, -0.6890657380265718945 ) ) ;
#23882=CARTESIAN_POINT ( 'NONE',  ( -1.115567212185924584, -78.90965635352397101, -1.056363245188180811 ) ) ;
#23900=CARTESIAN_POINT ( 'NONE',  ( 1.092232985442820992, -78.79166666666664298, 0.6295237254636267821 ) ) ;
#23916=CARTESIAN_POINT ( 'NONE',  ( -1.135826688880000157, -81.40663953506998496, -0.9797437077257000748 ) ) ;
#23925=CARTESIAN_POINT ( 'NONE',  ( -0.6571235693794531540, -81.51954227144281617, 1.063877270815418274 ) ) ;
#23930=CARTESIAN_POINT ( 'NONE',  ( 0.8011517691903999872, -77.75748566455999367, -1.033896367111999837 ) ) ;
#23956=CARTESIAN_POINT ( 'NONE',  ( -0.9536002873971000104, -79.19521021049000353, 1.318830682536000110 ) ) ;
#23958=CARTESIAN_POINT ( 'NONE',  ( -0.9292580750797257982, -79.15854484711744021, -0.8358713317426036404 ) ) ;
#23967=CARTESIAN_POINT ( 'NONE',  ( -1.468405992501000012, -81.36252996976000418, 0.5987774653158000060 ) ) ;
#23998=CARTESIAN_POINT ( 'NONE',  ( -0.5713041596650000331, -79.42507309447999830, -1.442599867604999808 ) ) ;
#23999=CARTESIAN_POINT ( 'NONE',  ( -0.6358204470927000251, -78.04511904209999784, -1.286007741733000032 ) ) ;
#24002=CARTESIAN_POINT ( 'NONE',  ( -0.9519843368319620414, -83.27853334735807778, 1.174365823974324652 ) ) ;
#24008=CARTESIAN_POINT ( 'NONE',  ( -0.9160563294565400305, -81.66020893391389279, -0.8511632488320945988 ) ) ;
#24010=PRESENTATION_STYLE_ASSIGNMENT (( #47061 ) ) ;
#24013=CARTESIAN_POINT ( 'NONE',  ( -0.9995835529977249445, -80.05208333333331439, -0.7681833999686439318 ) ) ;
#24028=DIRECTION ( 'NONE',  ( 0.000000000000000000, -1.000000000000000000, 0.000000000000000000 ) ) ;
#24039=CARTESIAN_POINT ( 'NONE',  ( 0.8322913257134999521, -79.47039037689999930, 1.209850638715999960 ) ) ;
#24081=CARTESIAN_POINT ( 'NONE',  ( 0.000000000000000000, -76.75499999999999545, 0.000000000000000000 ) ) ;
#24095=CARTESIAN_POINT ( 'NONE',  ( 1.155800523840101679, -82.81894139901449137, -0.4759988703850971392 ) ) ;
#24099=CARTESIAN_POINT ( 'NONE',  ( -1.165699973591947547, -78.19533224334435317, 0.9553630080629633703 ) ) ;
#24107=CARTESIAN_POINT ( 'NONE',  ( 0.9995835529977264988, -81.19791666666664298, -0.7681833999686417114 ) ) ;
#24118=CARTESIAN_POINT ( 'NONE',  ( -0.2410965598014278566, -82.99083135149682278, 1.228665170874773338 ) ) ;
#24120=CARTESIAN_POINT ( 'NONE',  ( -1.092232985442824100, -80.45833333333330017, 0.6295237254636200097 ) ) ;
#24135=STYLED_ITEM ( 'NONE', ( #20863 ), #36811 ) ;
#24142=CARTESIAN_POINT ( 'NONE',  ( 0.8286895765316001361, -81.72239288712999894, 1.445177540541999983 ) ) ;
#24145=ORIENTED_EDGE ( 'NONE', *, *, #29545, .T. ) ;
#24163=CARTESIAN_POINT ( 'NONE',  ( -1.006352879438885184, -80.54967111464023333, 0.7434871015420349005 ) ) ;
#24175=CARTESIAN_POINT ( 'NONE',  ( -0.2770819934162573883, -80.20771142070574911, -1.219419118597123930 ) ) ;
#24180=CARTESIAN_POINT ( 'NONE',  ( 1.433939993129704771, -78.57056504184866697, -0.5545599285302943438 ) ) ;
#24196=CARTESIAN_POINT ( 'NONE',  ( -1.288646058034000008, -83.49568302734098779, 0.4058063692239000098 ) ) ;
#24200=CARTESIAN_POINT ( 'NONE',  ( 0.6295237254636211199, -78.83333333333335702, 1.092232985442824322 ) ) ;
#24206=CARTESIAN_POINT ( 'NONE',  ( 0.4917238316050000502, -82.23466316459999348, -1.258641686703000140 ) ) ;
#24225=CARTESIAN_POINT ( 'NONE',  ( 0.4658870802631708830, -81.44483258142587090, 1.159784591535937937 ) ) ;
#24230=CARTESIAN_POINT ( 'NONE',  ( -1.175921224601000015, -78.54395921125998825, 0.5727056776607999389 ) ) ;
#24247=CARTESIAN_POINT ( 'NONE',  ( 1.218445119259581544, -82.37149458593418672, 0.3277830641851678384 ) ) ;
#24260=CARTESIAN_POINT ( 'NONE',  ( 1.328072050606999843, -78.53056612723000285, -0.9406846882429998891 ) ) ;
#24261=CARTESIAN_POINT ( 'NONE',  ( -1.003367537693320877, -79.15123299649694388, -0.7504123186897171394 ) ) ;
#24295=CARTESIAN_POINT ( 'NONE',  ( -0.5890800888495719700, -80.01449628974698669, 1.102351224369839677 ) ) ;
#24301=CARTESIAN_POINT ( 'NONE',  ( -0.5298108134926000634, -80.73036354008999638, 1.579417458585999912 ) ) ;
#24302=CARTESIAN_POINT ( 'NONE',  ( 1.170683199339999758, -78.65761630967999452, -0.8292048310924000631 ) ) ;
#24304=CARTESIAN_POINT ( 'NONE',  ( -0.9345908190077275579, -82.17710307665237224, 1.232018202299275611 ) ) ;
#24306=ORIENTED_EDGE ( 'NONE', *, *, #11738, .T. ) ;
#24308=CARTESIAN_POINT ( 'NONE',  ( 6.091423516370726666E-05, -80.97567851488123836, 1.280875928844625644 ) ) ;
#24310=CARTESIAN_POINT ( 'NONE',  ( 0.03373185335276917413, -81.72769218985609996, -1.249292863317937652 ) ) ;
#24317=EDGE_CURVE ( 'NONE', #56551, #41164, #35021, .T. ) ;
#24333=CARTESIAN_POINT ( 'NONE',  ( 1.250000000000000000, -81.24999999999998579, 0.000000000000000000 ) ) ;
#24342=CARTESIAN_POINT ( 'NONE',  ( 0.7712594847575999779, -80.60757119619998434, 1.518214662813999860 ) ) ;
#24359=CARTESIAN_POINT ( 'NONE',  ( 0.7088972746458148677, -78.42728435963773848, 1.029425822873615282 ) ) ;
#24375=CARTESIAN_POINT ( 'NONE',  ( 1.092232985442823212, -82.70833333333331439, -0.6295237254636224522 ) ) ;
#24384=LINE ( 'NONE', #42683, #37887 ) ;
#24394=CARTESIAN_POINT ( 'NONE',  ( -0.1639670297146121059, -82.71513557757415924, -1.249649658132720331 ) ) ;
#24399=CARTESIAN_POINT ( 'NONE',  ( -1.185909154492194695, -79.19522916700250903, 0.9691166662416358379 ) ) ;
#24419=CARTESIAN_POINT ( 'NONE',  ( 0.8703341916068573214, -82.91432341927395555, 0.8966700837326383455 ) ) ;
#24442=CARTESIAN_POINT ( 'NONE',  ( -0.6572886123566999972, -82.79609954400000049, 1.530761476772000140 ) ) ;
#24449=ORIENTED_EDGE ( 'NONE', *, *, #30681, .T. ) ;
#24459=ORIENTED_EDGE ( 'NONE', *, *, #24317, .T. ) ;
#24461=CARTESIAN_POINT ( 'NONE',  ( -0.6016272266181392769, -80.51522408813923448, 1.095825561504355061 ) ) ;
#24474=CARTESIAN_POINT ( 'NONE',  ( -0.5583711603394299061, -78.94535017580587066, -1.433472983738463435 ) ) ;
#24486=CARTESIAN_POINT ( 'NONE',  ( -1.232656909444999949, -83.05356852156999992, -0.5536498640889000455 ) ) ;
#24499=EDGE_LOOP ( 'NONE', ( #55234, #38467 ) ) ;
#24501=CARTESIAN_POINT ( 'NONE',  ( -0.2201363562291999698, -79.46327907014000402, -1.483758735329000045 ) ) ;
#24515=CARTESIAN_POINT ( 'NONE',  ( -0.4788088652293910341, -81.50646803775929072, 1.154537243539281555 ) ) ;
#24519=CARTESIAN_POINT ( 'NONE',  ( -1.250000000000000000, -82.09999999999999432, 0.000000000000000000 ) ) ;
#24521=CARTESIAN_POINT ( 'NONE',  ( -1.301447353884999991, -78.07207508323999434, 0.1304503950232999976 ) ) ;
#24549=CARTESIAN_POINT ( 'NONE',  ( 0.8819056695273819191, -81.68554651168997793, -0.9213067782626794822 ) ) ;
#24550=CARTESIAN_POINT ( 'NONE',  ( -0.7213013439201000354, -77.97728518351999583, -1.458901041394999876 ) ) ;
#24551=CARTESIAN_POINT ( 'NONE',  ( -1.151522233741549606, -79.13191606329839090, -0.4866886816611077915 ) ) ;
#24559=CARTESIAN_POINT ( 'NONE',  ( 0.2675321060165000153, -79.46759604279999678, -1.681415376183999832 ) ) ;
#24567=CARTESIAN_POINT ( 'NONE',  ( -0.03502584505609534354, -81.22258658432861012, -1.254136478721574299 ) ) ;
#24585=CARTESIAN_POINT ( 'NONE',  ( -1.121108069640562199, -81.13836208406755190, -0.5751273790267441566 ) ) ;
#24595=CARTESIAN_POINT ( 'NONE',  ( -0.4798816485349043925, -81.65077628406871213, 1.434309721071634236 ) ) ;
#24596=CARTESIAN_POINT ( 'NONE',  ( 1.502590276041740447, -82.58012170747866776, -0.3796259133681765263 ) ) ;
#24597=CARTESIAN_POINT ( 'NONE',  ( -1.058270554699162869, -79.64529829993477961, -0.6656290506933998374 ) ) ;
#24598=CARTESIAN_POINT ( 'NONE',  ( 1.218586970313583207, -80.87149228721223437, 0.3277392589856675809 ) ) ;
#24600=CARTESIAN_POINT ( 'NONE',  ( -0.4278239563775090293, -81.69741778646303487, -1.174506411635975134 ) ) ;
#24608=VERTEX_POINT ( 'NONE', #17419 ) ;
#24628=CARTESIAN_POINT ( 'NONE',  ( -0.4036326496859999891, -80.10214000165998982, 1.533452771621000021 ) ) ;
#24645=CARTESIAN_POINT ( 'NONE',  ( 0.6540410530999497540, -78.43152095752569153, 1.066316062253257702 ) ) ;
#24655=FACE_OUTER_BOUND ( 'NONE', #10353, .T. ) ;
#24662=EDGE_CURVE ( 'NONE', #7670, #54925, #5310, .T. ) ;
#24666=CARTESIAN_POINT ( 'NONE',  ( -0.3271848554490991434, -82.60416666666665719, -1.217465845835395299 ) ) ;
#24684=ORIENTED_EDGE ( 'NONE', *, *, #7574, .T. ) ;
#24688=CARTESIAN_POINT ( 'NONE',  ( -1.162279827862261916, -79.57043678867249525, 0.4597564725974967459 ) ) ;
#24689=CARTESIAN_POINT ( 'NONE',  ( 1.162102752763446878, -78.94315431229624380, -1.000785636504023524 ) ) ;
#24708=CARTESIAN_POINT ( 'NONE',  ( 0.8599086838611078587, -82.91523954447930578, 0.9066764497312405080 ) ) ;
#24712=CARTESIAN_POINT ( 'NONE',  ( 0.9995835529977233902, -80.30208333333334281, 0.7681833999686461523 ) ) ;
#24720=( NAMED_UNIT ( * ) SI_UNIT ( $, .STERADIAN. ) SOLID_ANGLE_UNIT ( ) );
#24727=DIRECTION ( 'NONE',  ( -1.000000000000000000, 0.000000000000000000, 0.000000000000000000 ) ) ;
#24740=CARTESIAN_POINT ( 'NONE',  ( 0.7676926012113186593, -80.77788394861798338, -0.9996391181222294975 ) ) ;
#24748=CARTESIAN_POINT ( 'NONE',  ( -0.008218136894757548452, -80.47612516791997450, 1.249622453350030638 ) ) ;
#24753=ORIENTED_EDGE ( 'NONE', *, *, #6783, .F. ) ;
#24755=ORIENTED_EDGE ( 'NONE', *, *, #20942, .T. ) ;
#24758=AXIS2_PLACEMENT_3D ( 'NONE', #37655, #14630, #50675 ) ;
#24769=FACE_OUTER_BOUND ( 'NONE', #44206, .T. ) ;
#24778=CARTESIAN_POINT ( 'NONE',  ( 0.9533626797078339488, -80.07179590631209010, 1.220572805882581990 ) ) ;
#24787=CARTESIAN_POINT ( 'NONE',  ( -0.6329778402533998705, -81.66623022861000436, -1.193863583722999833 ) ) ;
#24795=LINE ( 'NONE', #33924, #29862 ) ;
#24805=AXIS2_PLACEMENT_3D ( 'NONE', #290, #14115, #54853 ) ;
#24806=CARTESIAN_POINT ( 'NONE',  ( 0.4350654701194750507, -81.44699977334819607, 1.171762940142557552 ) ) ;
#24809=CARTESIAN_POINT ( 'NONE',  ( -0.7678540140355195609, -82.17356543371400335, -0.9996003491978228128 ) ) ;
#24811=CARTESIAN_POINT ( 'NONE',  ( 0.8160112056498999289, -78.81700217913999040, -1.163845997288000200 ) ) ;
#24841=CARTESIAN_POINT ( 'NONE',  ( -1.560595261880000084, -77.86592204395999772, 0.4619550309703999713 ) ) ;
#24842=CARTESIAN_POINT ( 'NONE',  ( -1.141620584689441609, -79.13348047058508428, -0.5094065323112431098 ) ) ;
#24849=CARTESIAN_POINT ( 'NONE',  ( -0.6962927961685000389, -82.42150394949298686, -1.554024870232999955 ) ) ;
#24850=CARTESIAN_POINT ( 'NONE',  ( 1.554657762476000071, -81.04657642056000100, -0.6948770361563999520 ) ) ;
#24874=DIRECTION ( 'NONE',  ( 0.000000000000000000, -1.000000000000000000, 0.000000000000000000 ) ) ;
#24876=CARTESIAN_POINT ( 'NONE',  ( -0.8402681406225442906, -80.03420601024139103, 0.9269689668249517789 ) ) ;
#24883=CARTESIAN_POINT ( 'NONE',  ( -0.9352798328955729268, -82.27646447274652530, 1.232869141408684754 ) ) ;
#24884=CARTESIAN_POINT ( 'NONE',  ( -0.4573940628493604055, -79.69555677089692836, -1.163073868470372974 ) ) ;
#24909=PRODUCT_DEFINITION_SHAPE ( 'NONE', 'NONE',  #39775 ) ;
#24915=CARTESIAN_POINT ( 'NONE',  ( 1.401632346086000069, -80.41793607721000114, -0.7415008327037999614 ) ) ;
#24944=CARTESIAN_POINT ( 'NONE',  ( -0.9802155852345567633, -82.04731661387214103, 0.7777929719928468044 ) ) ;
#24945=CARTESIAN_POINT ( 'NONE',  ( -0.6726658035522998791, -79.42188804861000051, -1.521367134781000052 ) ) ;
#24966=ORIENTED_EDGE ( 'NONE', *, *, #49890, .F. ) ;
#24967=CARTESIAN_POINT ( 'NONE',  ( 0.1572691907071377126, -82.73563599228513965, -1.240367807619981777 ) ) ;
#24972=CARTESIAN_POINT ( 'NONE',  ( 1.108327923370202361, -78.43900460289381726, -1.059889875604768106 ) ) ;
#24993=CARTESIAN_POINT ( 'NONE',  ( 1.217465845835393967, -80.27083333333332860, 0.3271848554491025851 ) ) ;
#25012=CARTESIAN_POINT ( 'NONE',  ( -1.374853770045000090, -81.36843355940999345, -0.7192078502473999713 ) ) ;
#25024=CARTESIAN_POINT ( 'NONE',  ( 0.9997866688655676626, -80.79871906944751458, -0.7680295045374020413 ) ) ;
#25029=ORIENTED_EDGE ( 'NONE', *, *, #40383, .F. ) ;
#25031=CARTESIAN_POINT ( 'NONE',  ( -0.1782592318590009717, -80.48666753183738365, 1.238841185009283308 ) ) ;
#25057=CARTESIAN_POINT ( 'NONE',  ( -0.9995835529977249445, -78.55208333333330017, -0.7681833999686439318 ) ) ;
#25060=CARTESIAN_POINT ( 'NONE',  ( 1.475564620878634159, -80.98274612424530972, -0.3262207497478352147 ) ) ;
#25071=CARTESIAN_POINT ( 'NONE',  ( 0.5343721329914999929, -82.29797985336999488, -1.367806479096000061 ) ) ;
#25088=CARTESIAN_POINT ( 'NONE',  ( 0.7175553326157163569, -81.42660517918807273, 1.024974559415771536 ) ) ;
#25092=B_SPLINE_CURVE_WITH_KNOTS ( 'NONE', 3,
 ( #7820, #3675, #43847, #21677, #42974, #56546, #57690, #2530, #34087, #11682, #52694, #57411, #21104, #2818, #47709, #25243, #20813, #39110 ),
 .UNSPECIFIED., .F., .F.,
 ( 4, 2, 2, 2, 2, 2, 2, 2, 4 ),
 ( 0.000000000000000000, 0.1249999999999999722, 0.2500000000000000000, 0.3750000000000000000, 0.5000000000000001110, 0.6250000000000001110, 0.7500000000000000000, 0.8750000000000000000, 1.000000000000000000 ),
 .UNSPECIFIED. ) ;
#25106=AXIS2_PLACEMENT_3D ( 'NONE', #7859, #3154, #43888 ) ;
#25124=CARTESIAN_POINT ( 'NONE',  ( 1.136899222205000060, -79.20227971866999894, 1.164526648744999893 ) ) ;
#25132=CARTESIAN_POINT ( 'NONE',  ( -1.321122997307999869, -79.84670880711999530, 0.8769429413327000100 ) ) ;
#25140=CARTESIAN_POINT ( 'NONE',  ( 1.187590719512276793, -81.32127699930184406, -0.4706845472736139180 ) ) ;
#25146=ORIENTED_EDGE ( 'NONE', *, *, #9512, .F. ) ;
#25152=CARTESIAN_POINT ( 'NONE',  ( -1.306018640041678225, -79.39152295432234041, -0.7583383393078939605 ) ) ;
#25167=CARTESIAN_POINT ( 'NONE',  ( -1.115142639999363361, -79.05850612728720250, 0.6526272847765023366 ) ) ;
#25169=CARTESIAN_POINT ( 'NONE',  ( 0.5739046245057122242, -83.00524183610107798, -1.400512781010780916 ) ) ;
#25171=ORIENTED_EDGE ( 'NONE', *, *, #5001, .F. ) ;
#25199=CARTESIAN_POINT ( 'NONE',  ( 1.585573224116000102, -81.04968570196999167, 0.6211121348122999875 ) ) ;
#25203=CARTESIAN_POINT ( 'NONE',  ( -1.416867025158235149, -79.77826750275583834, -0.5258000735673173942 ) ) ;
#25207=DIRECTION ( 'NONE',  ( 0.000000000000000000, -1.000000000000000000, 0.000000000000000000 ) ) ;
#25219=CARTESIAN_POINT ( 'NONE',  ( 1.484562552624000054, -81.98291553004999344, -0.7558657512595999828 ) ) ;
#25233=CARTESIAN_POINT ( 'NONE',  ( -0.8918818467572275921, -82.03888351926970302, 0.8753769929997189392 ) ) ;
#25234=CARTESIAN_POINT ( 'NONE',  ( -0.9554492926093999250, -78.75370921126000212, 1.361857491384999896 ) ) ;
#25243=CARTESIAN_POINT ( 'NONE',  ( 1.217465845835393967, -81.77083333333330017, 0.3271848554491025851 ) ) ;
#25249=EDGE_LOOP ( 'NONE', ( #57078, #13618, #39941 ) ) ;
#25256=VERTEX_POINT ( 'NONE', #5243 ) ;
#25261=CARTESIAN_POINT ( 'NONE',  ( -0.8109968711390208584, -78.17012475787373660, 1.272002705921249754 ) ) ;
#25269=CARTESIAN_POINT ( 'NONE',  ( -1.282582078921783664, -81.30480715895743060, 0.8019254487526868980 ) ) ;
#25276=EDGE_CURVE ( 'NONE', #8320, #12955, #10081, .T. ) ;
#25310=EDGE_CURVE ( 'NONE', #14217, #48338, #51895, .T. ) ;
#25318=CARTESIAN_POINT ( 'NONE',  ( 0.2421190662860195630, -80.45992770227913127, 1.227031503692224357 ) ) ;
#25343=CARTESIAN_POINT ( 'NONE',  ( 0.2749350294349880430, -79.88960586272550302, -1.486957691345828225 ) ) ;
#25354=CARTESIAN_POINT ( 'NONE',  ( 1.349879140156000190, -82.36113906847999999, -0.5781647238538999423 ) ) ;
#25369=VECTOR ( 'NONE', #18737, 1000.000000000000000 ) ;
#25373=CARTESIAN_POINT ( 'NONE',  ( -1.497546582071999977, -80.85273907906999113, 0.7298035716741000378 ) ) ;
#25377=CARTESIAN_POINT ( 'NONE',  ( 0.1638729951965073595, -82.23606986915045525, -1.249733270349860481 ) ) ;
#25387=VERTEX_POINT ( 'NONE', #31605 ) ;
#25410=EDGE_CURVE ( 'NONE', #13850, #30955, #41320, .T. ) ;
#25413=FACE_OUTER_BOUND ( 'NONE', #13755, .T. ) ;
#25414=CARTESIAN_POINT ( 'NONE',  ( 0.4102083068199999794, -78.47488455744999669, -1.574926093281000083 ) ) ;
#25416=CARTESIAN_POINT ( 'NONE',  ( -1.166171049469810983, -79.12942819682623963, -0.4499060407731832467 ) ) ;
#25423=CARTESIAN_POINT ( 'NONE',  ( 1.606311393998999915, -83.05309610059499903, -0.5653197666394998988 ) ) ;
#25424=CARTESIAN_POINT ( 'NONE',  ( 0.3526082373300999939, -80.03618645244999641, -1.545983222067000007 ) ) ;
#25428=CARTESIAN_POINT ( 'NONE',  ( -0.4492251327744000156, -81.60790313063000667, 1.604198796042999753 ) ) ;
#25432=CARTESIAN_POINT ( 'NONE',  ( 0.4638405057549351840, -81.25547559012920829, -1.160654197406111976 ) ) ;
#25440=CARTESIAN_POINT ( 'NONE',  ( 1.579899301681999990, -82.10529106903000240, 0.5283722218587000308 ) ) ;
#25444=DIRECTION ( 'NONE',  ( 0.000000000000000000, -1.000000000000000000, 1.258252761242000063E-14 ) ) ;
#25455=CARTESIAN_POINT ( 'NONE',  ( 0.1633825985461731523, -78.96481209864140283, 1.249810919385931030 ) ) ;
#25457=CARTESIAN_POINT ( 'NONE',  ( -1.227822524791635894, -82.29670828839515195, 0.9447229247095449978 ) ) ;
#25458=CARTESIAN_POINT ( 'NONE',  ( -1.137583167366030601, -79.63440963302888065, -0.5175359492836348885 ) ) ;
#25465=ORIENTED_EDGE ( 'NONE', *, *, #26429, .F. ) ;
#25485=EDGE_CURVE ( 'NONE', #31243, #36858, #48690, .T. ) ;
#25486=CARTESIAN_POINT ( 'NONE',  ( -0.8477325451633000997, -79.28107020522999449, -1.148851298854000058 ) ) ;
#25520=CARTESIAN_POINT ( 'NONE',  ( 1.225067527671359402, -81.86605588079059714, 0.2479480639099045647 ) ) ;
#25535=ORIENTED_EDGE ( 'NONE', *, *, #18038, .F. ) ;
#25537=AXIS2_PLACEMENT_3D ( 'NONE', #25725, #3013, #21009 ) ;
#25543=CARTESIAN_POINT ( 'NONE',  ( 0.8653617893380854964, -82.78648746760886468, -0.9018584769693096526 ) ) ;
#25547=CARTESIAN_POINT ( 'NONE',  ( -0.6256548411826953204, -79.51725861580031562, 1.084699083566985189 ) ) ;
#25565=CARTESIAN_POINT ( 'NONE',  ( 1.151824538291304378, -82.88178188827541248, 0.4855375567635726308 ) ) ;
#25603=CARTESIAN_POINT ( 'NONE',  ( 0.7926223457823362573, -80.42074650411231573, 0.9670736177117366106 ) ) ;
#25612=AXIS2_PLACEMENT_3D ( 'NONE', #1669, #5784, #6951 ) ;
#25625=CARTESIAN_POINT ( 'NONE',  ( -0.7681833999686477066, -83.42708333333331439, 0.9995835529977223910 ) ) ;
#25631=CARTESIAN_POINT ( 'NONE',  ( 1.179653558262802049, -81.05359780786231738, 0.9428567377702261609 ) ) ;
#25640=CARTESIAN_POINT ( 'NONE',  ( 1.424157265477999923, -82.99288869324199425, 0.6972603243668999973 ) ) ;
#25643=CARTESIAN_POINT ( 'NONE',  ( -1.250000000000000000, -81.99999999999998579, 0.000000000000000000 ) ) ;
#25656=CARTESIAN_POINT ( 'NONE',  ( 1.250000000000000000, -80.74999999999998579, 0.000000000000000000 ) ) ;
#25658=CARTESIAN_POINT ( 'NONE',  ( 1.551146335801999898, -81.10931883074999860, 0.6076261867840000441 ) ) ;
#25696=CARTESIAN_POINT ( 'NONE',  ( 0.6727641735938050260, -81.66943313961250794, -1.083490727392691033 ) ) ;
#25699=CARTESIAN_POINT ( 'NONE',  ( -1.168412079197438169, -79.12903572094943172, -0.4440620687051278770 ) ) ;
#25708=CARTESIAN_POINT ( 'NONE',  ( 1.463006681111000074, -81.53727493794998793, -0.8714086385761999898 ) ) ;
#25709=CARTESIAN_POINT ( 'NONE',  ( 0.7181780477660000273, -80.73093781866000995, 1.413724517075999998 ) ) ;
#25714=CARTESIAN_POINT ( 'NONE',  ( -1.519662023741000123, -82.74476900261298340, -0.6825586799200999977 ) ) ;
#25725=CARTESIAN_POINT ( 'NONE',  ( 0.000000000000000000, -76.75499999999999545, 0.000000000000000000 ) ) ;
#25735=CARTESIAN_POINT ( 'NONE',  ( 0.4666069534000411023, -79.94482168187342097, 1.159469772846831948 ) ) ;
#25742=CARTESIAN_POINT ( 'NONE',  ( 1.137309322218171381, -82.53963407618115866, -1.048735418599893832 ) ) ;
#25744=CARTESIAN_POINT ( 'NONE',  ( 0.5791152278277256205, -79.76384116944609559, -1.107571749123516192 ) ) ;
#25815=DIRECTION ( 'NONE',  ( 0.000000000000000000, -1.000000000000000000, 0.000000000000000000 ) ) ;
#25836=CARTESIAN_POINT ( 'NONE',  ( 0.7848080566249374668, -77.91804990316740032, -1.315710784708647108 ) ) ;
#25844=CARTESIAN_POINT ( 'NONE',  ( 1.194439549549000112, -80.29130269966999833, -0.6318903263597999143 ) ) ;
#25869=AXIS2_PLACEMENT_3D ( 'NONE', #48278, #25815, #38527 ) ;
#25881=EDGE_LOOP ( 'NONE', ( #24966, #41231 ) ) ;
#25890=CARTESIAN_POINT ( 'NONE',  ( 1.089041876986236002, -80.39116380685027252, 0.6134409219567780180 ) ) ;
#25912=CARTESIAN_POINT ( 'NONE',  ( 0.1636246173744642929, -83.36458333333334281, 1.250000000000000888 ) ) ;
#25918=CARTESIAN_POINT ( 'NONE',  ( 0.1201377420412941266, -80.61836603707203608, 1.540619319635312401 ) ) ;
#25927=CARTESIAN_POINT ( 'NONE',  ( -0.6483708932059000229, -82.29813732702999118, -1.447070110047999902 ) ) ;
#25929=EDGE_LOOP ( 'NONE', ( #46470, #1979, #686, #48675 ) ) ;
#25948=CARTESIAN_POINT ( 'NONE',  ( -0.6332123272625999055, -81.29485358483999846, 1.540853336418999797 ) ) ;
#25960=CARTESIAN_POINT ( 'NONE',  ( -0.1956594527234810643, -79.26382142333196157, -1.318569963859137495 ) ) ;
#25976=CARTESIAN_POINT ( 'NONE',  ( 0.9995835529977264988, -83.19791666666662877, -0.7681833999686417114 ) ) ;
#25986=CARTESIAN_POINT ( 'NONE',  ( -0.9172530285194190336, -83.04126087647844656, 0.8486422117887013616 ) ) ;
#25992=CARTESIAN_POINT ( 'NONE',  ( 1.539929345890999945, -80.16250488267000662, 0.3781723503825999422 ) ) ;
#25993=CARTESIAN_POINT ( 'NONE',  ( -1.247959326960667914, -77.91666666666564822, 0.5507335004918384458 ) ) ;
#25997=CARTESIAN_POINT ( 'NONE',  ( -1.324613189995999862, -83.30925904736399445, -0.7038465009425000085 ) ) ;
#26003=ORIENTED_EDGE ( 'NONE', *, *, #40514, .F. ) ;
#26008=CARTESIAN_POINT ( 'NONE',  ( -1.588687380433000174, -83.30531615612299845, 0.5002921117598999601 ) ) ;
#26016=CARTESIAN_POINT ( 'NONE',  ( 0.4202526907024859981, -79.94806991484146863, 1.177036590369186397 ) ) ;
#26022=CARTESIAN_POINT ( 'NONE',  ( 1.329645096041070840, -81.63878427981505581, 0.7189625959783054743 ) ) ;
#26024=CIRCLE ( 'NONE', #29803, 10.05000000000000071 ) ;
#26041=CARTESIAN_POINT ( 'NONE',  ( 0.6297217878212084674, -82.43399434138464699, 1.093297131891592278 ) ) ;
#26092=CARTESIAN_POINT ( 'NONE',  ( 1.151300139434892067, -81.88191447522581257, 0.4866929889698630163 ) ) ;
#26102=CARTESIAN_POINT ( 'NONE',  ( -0.3273598336528602548, -78.20425139990393859, -1.217721295151624750 ) ) ;
#26147=ADVANCED_FACE ( 'NONE', ( #35420 ), #818, .F. ) ;
#26148=ORIENTED_EDGE ( 'NONE', *, *, #43456, .T. ) ;
#26171=CYLINDRICAL_SURFACE ( 'NONE', #57902, 10.14999999999999858 ) ;
#26182=ORIENTED_EDGE ( 'NONE', *, *, #38342, .F. ) ;
#26209=CARTESIAN_POINT ( 'NONE',  ( -1.118791686563179066, -79.90798387919549839, -1.016611780088532591 ) ) ;
#26218=CARTESIAN_POINT ( 'NONE',  ( -1.339567984323000172, -82.67693514403299559, -0.6016691479808000675 ) ) ;
#26221=CARTESIAN_POINT ( 'NONE',  ( -0.1636246173744673738, -82.11458333333330017, -1.249999999999999778 ) ) ;
#26232=CARTESIAN_POINT ( 'NONE',  ( -10.14999999998000035, -87.10000000002298748, 2.878919856867000406E-10 ) ) ;
#26236=DIRECTION ( 'NONE',  ( 0.000000000000000000, -1.000000000000000000, 0.000000000000000000 ) ) ;
#26252=CARTESIAN_POINT ( 'NONE',  ( -0.5985389898873999526, -79.29977142615000218, -1.413233628500000005 ) ) ;
#26256=CARTESIAN_POINT ( 'NONE',  ( 0.1323978365314348593, -80.23382476822598619, -1.243286041401693742 ) ) ;
#26279=CARTESIAN_POINT ( 'NONE',  ( -0.7704861717791524622, -83.02778078094171121, 0.9968608840825577966 ) ) ;
#26283=CARTESIAN_POINT ( 'NONE',  ( -1.486328135279999962, -82.42166142315099364, -0.5524720742449998889 ) ) ;
#26284=CARTESIAN_POINT ( 'NONE',  ( -1.320073427535999988, -80.92057293764999315, 0.6433150820290999272 ) ) ;
#26288=CARTESIAN_POINT ( 'NONE',  ( 0.7311670807272000472, -82.05001763639998558, 1.496881327486000002 ) ) ;
#26304=CARTESIAN_POINT ( 'NONE',  ( -0.1955901218635645589, -79.56269089637430625, -1.318552432567616783 ) ) ;
#26310=B_SPLINE_CURVE_WITH_KNOTS ( 'NONE', 3,
 ( #34767, #16786, #30045, #17066, #7342, #3490, #11500, #56366, #6766, #12348, #47529, #21494, #29474, #25057, #47811, #57504, #39500, #30335 ),
 .UNSPECIFIED., .F., .F.,
 ( 4, 2, 2, 2, 2, 2, 2, 2, 4 ),
 ( 0.000000000000000000, 0.1250000000000000833, 0.2500000000000001110, 0.3750000000000000000, 0.4999999999999999445, 0.6249999999999998890, 0.7499999999999997780, 0.8749999999999998890, 1.000000000000000000 ),
 .UNSPECIFIED. ) ;
#26313=CARTESIAN_POINT ( 'NONE',  ( 1.106525018319362674, -81.65902809546365404, 1.029255714463842786 ) ) ;
#26375=CARTESIAN_POINT ( 'NONE',  ( 0.6088572233645838105, -81.93455332008454661, 1.091931018960549560 ) ) ;
#26376=CARTESIAN_POINT ( 'NONE',  ( -0.5800742227073999446, -79.54852142615000332, -1.311952909603000039 ) ) ;
#26378=CARTESIAN_POINT ( 'NONE',  ( -1.430508845346486702, -82.72367320741450669, 0.4901804664080808838 ) ) ;
#26401=VERTEX_POINT ( 'NONE', #22958 ) ;
#26417=EDGE_CURVE ( 'NONE', #9574, #13712, #51478, .T. ) ;
#26427=CARTESIAN_POINT ( 'NONE',  ( 0.000000000000000000, -83.49999999999998579, 0.000000000000000000 ) ) ;
#26429=EDGE_CURVE ( 'NONE', #19092, #515, #52924, .T. ) ;
#26445=EDGE_LOOP ( 'NONE', ( #38027, #41150, #37663, #21718, #26914 ) ) ;
#26481=CARTESIAN_POINT ( 'NONE',  ( 0.6295237254636211199, -83.33333333333332860, 1.092232985442824322 ) ) ;
#26488=CARTESIAN_POINT ( 'NONE',  ( 0.5215562184170206006, -80.69749268949153986, 1.459483306257267854 ) ) ;
#26498=CARTESIAN_POINT ( 'NONE',  ( -1.542276019614999827, -82.23513558557998238, 0.7219429580085000575 ) ) ;
#26509=VERTEX_POINT ( 'NONE', #47171 ) ;
#26516=CARTESIAN_POINT ( 'NONE',  ( -0.4240539849974000464, -80.28430614307998781, 1.611036072322000079 ) ) ;
#26523=VERTEX_POINT ( 'NONE', #34704 ) ;
#26532=CARTESIAN_POINT ( 'NONE',  ( -1.481892012897999988, -78.73390927755998803, 0.7217217885958999712 ) ) ;
#26535=CARTESIAN_POINT ( 'NONE',  ( -1.456099130830773136, -79.27085162341434454, -0.3904854336919924562 ) ) ;
#26536=CARTESIAN_POINT ( 'NONE',  ( -0.1112851791610966062, -80.21855645632498977, -1.247194601161994543 ) ) ;
#26559=CARTESIAN_POINT ( 'NONE',  ( 0.7304821784857000733, -81.79022674571000096, 1.273910602969000161 ) ) ;
#26565=CARTESIAN_POINT ( 'NONE',  ( -1.508789225394999933, -82.17633606662001000, 0.7062677124845000431 ) ) ;
#26576=CARTESIAN_POINT ( 'NONE',  ( -1.596536837631000072, -81.79343788471999233, -0.4757406268331999533 ) ) ;
#26585=CARTESIAN_POINT ( 'NONE',  ( 0.8052405978830968758, -79.91960879271107387, 0.9563048914733230932 ) ) ;
#26601=ORIENTED_EDGE ( 'NONE', *, *, #11831, .T. ) ;
#26607=CARTESIAN_POINT ( 'NONE',  ( -1.249727466589207525, -82.59024373000691810, 0.1639556666535628981 ) ) ;
#26611=CARTESIAN_POINT ( 'NONE',  ( 1.250002295818805509, -79.35918108845754659, 0.1442765043559274540 ) ) ;
#26657=AXIS2_PLACEMENT_3D ( 'NONE', #38913, #52218, #39197 ) ;
#26662=CARTESIAN_POINT ( 'NONE',  ( 0.6397441051095902331, -81.93232338606405563, 1.073892556932021236 ) ) ;
#26663=CARTESIAN_POINT ( 'NONE',  ( 0.3696045101069000416, -79.60420299592999527, -1.269527782653000036 ) ) ;
#26665=CARTESIAN_POINT ( 'NONE',  ( -1.463637355772988258, -83.22975666182372834, 0.3812367531431999357 ) ) ;
#26674=EDGE_CURVE ( 'NONE', #8817, #7824, #5041, .T. ) ;
#26697=CARTESIAN_POINT ( 'NONE',  ( 0.1865657191063679332, -77.88443992253993997, -1.522241462990436611 ) ) ;
#26705=FACE_OUTER_BOUND ( 'NONE', #6159, .T. ) ;
#26713=B_SPLINE_CURVE_WITH_KNOTS ( 'NONE', 3,
 ( #40066, #48941, #48372, #4055 ),
 .UNSPECIFIED., .F., .F.,
 ( 4, 4 ),
 ( 0.000000000000000000, 1.000000000000000000 ),
 .UNSPECIFIED. ) ;
#26766=DIRECTION ( 'NONE',  ( 0.000000000000000000, -1.000000000000000000, 0.000000000000000000 ) ) ;
#26784=CARTESIAN_POINT ( 'NONE',  ( -0.2986795320787701824, -79.95859341831706502, -1.481281548820393423 ) ) ;
#26794=CARTESIAN_POINT ( 'NONE',  ( -1.596184505169000012, -82.29829480068998748, -0.5933059756569000198 ) ) ;
#26810=DIRECTION ( 'NONE',  ( 0.000000000000000000, 0.000000000000000000, -1.000000000000000000 ) ) ;
#26813=CARTESIAN_POINT ( 'NONE',  ( -0.5713041596650000331, -79.48428941834998795, -1.442599867604999808 ) ) ;
#26830=CARTESIAN_POINT ( 'NONE',  ( -1.630350418686000280, -79.25822497536000810, 0.2425001497127999839 ) ) ;
#26832=EDGE_LOOP ( 'NONE', ( #4037, #12831, #24306, #5369 ) ) ;
#26835=CARTESIAN_POINT ( 'NONE',  ( 1.071781563306112961, -80.30709819530763127, -0.6451663486076436582 ) ) ;
#26861=CARTESIAN_POINT ( 'NONE',  ( 0.4644997175289000135, -83.30604790835199935, 1.393065715888999856 ) ) ;
#26863=CARTESIAN_POINT ( 'NONE',  ( 0.6904535216592000424, -80.35229747532000033, 1.161570125514999940 ) ) ;
#26885=DIRECTION ( 'NONE',  ( 0.000000000000000000, 1.000000000000000000, 0.000000000000000000 ) ) ;
#26888=CARTESIAN_POINT ( 'NONE',  ( 0.7858904643604428530, -79.92117315916847531, 0.9723009331349696804 ) ) ;
#26894=CARTESIAN_POINT ( 'NONE',  ( 1.502971460259269421, -81.60841855634211583, 0.1731872554293665267 ) ) ;
#26914=ORIENTED_EDGE ( 'NONE', *, *, #21743, .F. ) ;
#26935=CARTESIAN_POINT ( 'NONE',  ( 1.250000000000000000, -80.34999999999999432, 0.000000000000000000 ) ) ;
#26960=CARTESIAN_POINT ( 'NONE',  ( -0.5432945554243000519, -81.30668225856999243, -1.398152719143000100 ) ) ;
#26961=CARTESIAN_POINT ( 'NONE',  ( 1.427761453950999959, -79.21443200746999480, 0.1399187141794999978 ) ) ;
#26963=CARTESIAN_POINT ( 'NONE',  ( 1.136477888908663081, -82.44026647294511179, -1.048016447884216662 ) ) ;
#26968=CARTESIAN_POINT ( 'NONE',  ( 0.9664454468687677657, -81.79568272211004398, -0.7933871688991031013 ) ) ;
#26973=ORIENTED_EDGE ( 'NONE', *, *, #46120, .F. ) ;
#26975=EDGE_CURVE ( 'NONE', #19162, #10981, #26024, .T. ) ;
#27000=CARTESIAN_POINT ( 'NONE',  ( -1.214718215476999985, -80.54393956010999034, 0.5919720313516000365 ) ) ;
#27002=CARTESIAN_POINT ( 'NONE',  ( -0.6014246001485028525, -79.18513522466939492, -1.095746199531517862 ) ) ;
#27054=ORIENTED_EDGE ( 'NONE', *, *, #16360, .T. ) ;
#27079=CARTESIAN_POINT ( 'NONE',  ( 1.349333182780099394, -81.06188137117389658, -0.6856402333970393892 ) ) ;
#27081=CARTESIAN_POINT ( 'NONE',  ( -0.9976490992766898769, -78.54879995622603417, 0.7538695216397535148 ) ) ;
#27091=CARTESIAN_POINT ( 'NONE',  ( -0.7976765672644999805, -81.85618029491999437, -1.504502914139000058 ) ) ;
#27115=ORIENTED_EDGE ( 'NONE', *, *, #42314, .F. ) ;
#27123=CARTESIAN_POINT ( 'NONE',  ( 1.437308235806999956, -78.98518200747000151, 0.5384467711458000849 ) ) ;
#27128=CARTESIAN_POINT ( 'NONE',  ( 1.046031006193842927, -80.30401498017664608, -0.6871684749293296424 ) ) ;
#27148=CARTESIAN_POINT ( 'NONE',  ( 0.5770204343780001022, -82.54797985337199862, -1.476971271490000071 ) ) ;
#27154=CARTESIAN_POINT ( 'NONE',  ( -0.6572886123566999972, -82.67766689626199650, 1.530761476772000140 ) ) ;
#27170=CARTESIAN_POINT ( 'NONE',  ( 1.249029712508835432, -79.33891269701508975, -0.1789285167953770239 ) ) ;
#27177=CARTESIAN_POINT ( 'NONE',  ( -1.250000000000000000, -81.59999999999999432, 0.000000000000000000 ) ) ;
#27181=CARTESIAN_POINT ( 'NONE',  ( 1.519477976411357734, -81.58817474069346076, -0.2151540744559326535 ) ) ;
#27213=CARTESIAN_POINT ( 'NONE',  ( -0.7004323366084000968, -78.30077033992999702, -1.469032877812000093 ) ) ;
#27216=CARTESIAN_POINT ( 'NONE',  ( 0.7681833999686451531, -78.17708333333332860, -0.9995835529977240563 ) ) ;
#27247=CIRCLE ( 'NONE', #30054, 3.000000000000000000 ) ;
#27251=CARTESIAN_POINT ( 'NONE',  ( -0.9131908197385000259, -81.28562918685999250, -1.254418330386999791 ) ) ;
#27252=CARTESIAN_POINT ( 'NONE',  ( -0.9160157088357999688, -77.75144095521999077, 1.388507278780999998 ) ) ;
#27254=CARTESIAN_POINT ( 'NONE',  ( -0.3124162970411396567, -82.35929312023905879, -1.516261523662276511 ) ) ;
#27263=CARTESIAN_POINT ( 'NONE',  ( 0.9259190077282706266, -81.79188721789226690, -0.8394937396800135065 ) ) ;
#27268=CARTESIAN_POINT ( 'NONE',  ( 1.250000000000000000, -80.25000000000000000, 0.000000000000000000 ) ) ;
#27293=CARTESIAN_POINT ( 'NONE',  ( -1.223477145616999939, -79.59670880711999530, 0.8121269926547999285 ) ) ;
#27330=CARTESIAN_POINT ( 'NONE',  ( 1.250000000000000000, -82.24999999999998579, 0.000000000000000000 ) ) ;
#27345=EDGE_LOOP ( 'NONE', ( #595, #14068, #36140, #2406 ) ) ;
#27375=CARTESIAN_POINT ( 'NONE',  ( -0.6295237254636286695, -80.91666666666667140, 1.092232985442819881 ) ) ;
#27377=CARTESIAN_POINT ( 'NONE',  ( -1.513474386345976086, -80.33310400781647331, 0.3226607623109409295 ) ) ;
#27379=CARTESIAN_POINT ( 'NONE',  ( -0.9465222407332000154, -81.55663953507000485, -0.8164530897714000757 ) ) ;
#27387=CARTESIAN_POINT ( 'NONE',  ( -1.405367936307999832, -81.30880043062998652, -0.7351702954167999016 ) ) ;
#27388=ORIENTED_EDGE ( 'NONE', *, *, #58205, .T. ) ;
#27415=CARTESIAN_POINT ( 'NONE',  ( -1.249603222883986842, -80.59829424211288540, 0.03721083154114489255 ) ) ;
#27423=CARTESIAN_POINT ( 'NONE',  ( -0.1614608359008000149, -79.09004514702999700, 1.526338918310999881 ) ) ;
#27431=CARTESIAN_POINT ( 'NONE',  ( -1.750000000000000000, -77.50000000000000000, 0.000000000000000000 ) ) ;
#27437=DIRECTION ( 'NONE',  ( 1.000000000000000000, 0.000000000000000000, 0.000000000000000000 ) ) ;
#27439=CARTESIAN_POINT ( 'NONE',  ( 0.000000000000000000, -76.75499999999999545, 0.000000000000000000 ) ) ;
#27445=CARTESIAN_POINT ( 'NONE',  ( 1.457613149566999944, -82.61113906848200372, -0.6243081169531999874 ) ) ;
#27446=CARTESIAN_POINT ( 'NONE',  ( 1.194439549549000112, -80.73125276597998834, -0.6318903263597999143 ) ) ;
#27457=CYLINDRICAL_SURFACE ( 'NONE', #20091, 9.500000000000000000 ) ;
#27473=CARTESIAN_POINT ( 'NONE',  ( -0.4814337422054900673, -81.50665477282878157, 1.153442787083076793 ) ) ;
#27501=ADVANCED_FACE ( 'NONE', ( #11948 ), #54324, .T. ) ;
#27506=CARTESIAN_POINT ( 'NONE',  ( -0.8961266428360998848, -77.63259150256999419, 1.358359200922999888 ) ) ;
#27512=VERTEX_POINT ( 'NONE', #29926 ) ;
#27544=CARTESIAN_POINT ( 'NONE',  ( 1.251226418338000190, -78.09316549288999454, -0.9133082017320000023 ) ) ;
#27546=CARTESIAN_POINT ( 'NONE',  ( 1.290261244888944558, -82.95647159644285296, -0.7858742426583964491 ) ) ;
#27552=CARTESIAN_POINT ( 'NONE',  ( 0.6127881360814133593, -81.76611797205174526, -1.089408548475932381 ) ) ;
#27564=AXIS2_PLACEMENT_3D ( 'NONE', #2673, #42245, #20950 ) ;
#27583=CARTESIAN_POINT ( 'NONE',  ( 1.426111243542000029, -79.91250488267000662, 0.3502211593775000353 ) ) ;
#27597=CARTESIAN_POINT ( 'NONE',  ( 0.3271848554491016414, -79.14583333333330017, -1.217465845835393967 ) ) ;
#27615=PLANE ( 'NONE',  #12530 ) ;
#27625=ORIENTED_EDGE ( 'NONE', *, *, #34452, .F. ) ;
#27635=CIRCLE ( 'NONE', #44632, 10.05000000000000071 ) ;
#27665=CARTESIAN_POINT ( 'NONE',  ( 1.092232985442820992, -80.79166666666665719, 0.6295237254636267821 ) ) ;
#27667=CARTESIAN_POINT ( 'NONE',  ( 1.024957315614702491, -79.66505809141212069, 1.112825025314110539 ) ) ;
#27668=CARTESIAN_POINT ( 'NONE',  ( -1.250000000000000000, -81.51887984502332074, -0.2965639121358149555 ) ) ;
#27672=CARTESIAN_POINT ( 'NONE',  ( 1.250000000000000000, -82.24999999999998579, 0.000000000000000000 ) ) ;
#27675=CARTESIAN_POINT ( 'NONE',  ( -1.392304720662999928, -81.22443067016000384, -0.3162235598901000366 ) ) ;
#27684=CARTESIAN_POINT ( 'NONE',  ( -9.950000000000001066, -86.20000000000000284, 0.000000000000000000 ) ) ;
#27711=CARTESIAN_POINT ( 'NONE',  ( -0.9961134219653000610, -78.77545572834999632, -1.167706195293999993 ) ) ;
#27714=CARTESIAN_POINT ( 'NONE',  ( -1.250000000000000000, -80.09999999999999432, 0.000000000000000000 ) ) ;
#27736=CARTESIAN_POINT ( 'NONE',  ( -0.2566745418018999692, -79.91018296954999300, 1.326684981396999863 ) ) ;
#27738=CARTESIAN_POINT ( 'NONE',  ( 0.6295237254636211199, -82.83333333333334281, 1.092232985442824322 ) ) ;
#27765=CARTESIAN_POINT ( 'NONE',  ( -0.7940971814358512848, -81.53031153321056479, 0.9681523155726415863 ) ) ;
#27797=CARTESIAN_POINT ( 'NONE',  ( -1.472167250137000005, -78.80543922203000307, -0.6938203229310999642 ) ) ;
#27821=EDGE_CURVE ( 'NONE', #14217, #36091, #52040, .T. ) ;
#27831=AXIS2_PLACEMENT_3D ( 'NONE', #35367, #16811, #44538 ) ;
#27834=CARTESIAN_POINT ( 'NONE',  ( -0.4240539849974000464, -80.16587349533999429, 1.611036072322000079 ) ) ;
#27835=CARTESIAN_POINT ( 'NONE',  ( -1.265859449240000156, -77.99707259131000114, 0.3747096735211999929 ) ) ;
#27838=CARTESIAN_POINT ( 'NONE',  ( 0.8891700687157699790, -82.07588638577088602, 1.268013924794865188 ) ) ;
#27839=CARTESIAN_POINT ( 'NONE',  ( 1.510174625183769548, -83.09633900652015370, -0.05656285966305413943 ) ) ;
#27843=CARTESIAN_POINT ( 'NONE',  ( -1.095039581810170581, -81.64041251720371406, -0.6026378644521110939 ) ) ;
#27848=EDGE_LOOP ( 'NONE', ( #8836, #32129, #46265, #33662 ) ) ;
#27851=CARTESIAN_POINT ( 'NONE',  ( 0.000000000000000000, -80.69999999999998863, 0.000000000000000000 ) ) ;
#27858=LINE ( 'NONE', #41160, #52063 ) ;
#27871=CARTESIAN_POINT ( 'NONE',  ( -0.4670233199325999895, -80.54409703377000085, 1.392241846115000126 ) ) ;
#27900=DIRECTION ( 'NONE',  ( 1.000000000000000000, 0.000000000000000000, 0.000000000000000000 ) ) ;
#27906=CARTESIAN_POINT ( 'NONE',  ( 0.3271848554491016414, -82.64583333333331439, -1.217465845835393967 ) ) ;
#27927=AXIS2_PLACEMENT_3D ( 'NONE', #31272, #44887, #53155 ) ;
#27958=CARTESIAN_POINT ( 'NONE',  ( 1.250000000000000000, -80.74999999999998579, 0.000000000000000000 ) ) ;
#27966=AXIS2_PLACEMENT_3D ( 'NONE', #13275, #17135, #1194 ) ;
#27992=EDGE_CURVE ( 'NONE', #13108, #24608, #24795, .T. ) ;
#28002=CARTESIAN_POINT ( 'NONE',  ( -1.152121943227528034, -80.13187642228581353, -0.4845792447579237994 ) ) ;
#28009=CARTESIAN_POINT ( 'NONE',  ( -1.050373044531177857, -78.78472797553973805, 1.124121219058911159 ) ) ;
#28056=AXIS2_PLACEMENT_3D ( 'NONE', #55903, #33148, #50898 ) ;
#28060=CARTESIAN_POINT ( 'NONE',  ( 1.201541383778999883, -77.86234880411998915, 0.5167982821483999567 ) ) ;
#28086=CARTESIAN_POINT ( 'NONE',  ( -0.9536002873971000104, -79.25442653435999318, 1.318830682536000110 ) ) ;
#28123=CARTESIAN_POINT ( 'NONE',  ( -0.7048934085577001074, -80.80140853768000397, -1.509431780672999990 ) ) ;
#28124=CARTESIAN_POINT ( 'NONE',  ( 1.077250838572999969, -78.72093299843999148, -0.7630258981648999628 ) ) ;
#28126=CARTESIAN_POINT ( 'NONE',  ( 0.7766941700662266523, -81.41797789504143168, -1.295155736999946461 ) ) ;
#28129=CARTESIAN_POINT ( 'NONE',  ( 1.183919390960944007, -79.82443352179983265, -0.4012659760898111827 ) ) ;
#28133=CARTESIAN_POINT ( 'NONE',  ( 0.06645687873235063547, -81.72973678372032680, -1.248208688943512001 ) ) ;
#28135=CARTESIAN_POINT ( 'NONE',  ( -1.092232985442822102, -80.04166666666664298, -0.6295237254636245616 ) ) ;
#28137=VERTEX_POINT ( 'NONE', #23916 ) ;
#28149=ORIENTED_EDGE ( 'NONE', *, *, #50687, .F. ) ;
#28161=CARTESIAN_POINT ( 'NONE',  ( -1.425428639595999858, -80.67057293764999315, 0.6946581327067000711 ) ) ;
#28181=CARTESIAN_POINT ( 'NONE',  ( 1.250000000000000000, -79.25000000000000000, 0.000000000000000000 ) ) ;
#28201=ORIENTED_EDGE ( 'NONE', *, *, #13889, .T. ) ;
#28238=CARTESIAN_POINT ( 'NONE',  ( 1.087185650191391462, -82.89120236429288013, 0.6181942457068143604 ) ) ;
#28247=CARTESIAN_POINT ( 'NONE',  ( -0.6295237254636235624, -80.58333333333332860, -1.092232985442822990 ) ) ;
#28276=CARTESIAN_POINT ( 'NONE',  ( -1.239625094629522195, -80.61368471397051394, -0.2079133391517598850 ) ) ;
#28293=CARTESIAN_POINT ( 'NONE',  ( -0.9219487215672478309, -80.15967048775068804, -0.8452775506683704032 ) ) ;
#28296=CARTESIAN_POINT ( 'NONE',  ( 1.041440387436121107, -78.03515770762014370, -1.092726133770612229 ) ) ;
#28298=ORIENTED_EDGE ( 'NONE', *, *, #24662, .T. ) ;
#28315=CARTESIAN_POINT ( 'NONE',  ( 1.249999999999999778, -78.76041666666667140, 0.1636246173744711763 ) ) ;
#28325=EDGE_CURVE ( 'NONE', #26401, #40202, #4643, .T. ) ;
#28327=CARTESIAN_POINT ( 'NONE',  ( -1.250000000000000000, -79.10000000000000853, 0.000000000000000000 ) ) ;
#28343=CARTESIAN_POINT ( 'NONE',  ( -1.121649604080707796, -81.56336073363873140, 0.5583008101125926936 ) ) ;
#28350=CARTESIAN_POINT ( 'NONE',  ( 0.6336387951535999985, -77.91478037390000111, 1.144239716453000044 ) ) ;
#28379=CARTESIAN_POINT ( 'NONE',  ( 1.153380192234999990, -78.52349661904999323, 1.148206073167999941 ) ) ;
#28388=CARTESIAN_POINT ( 'NONE',  ( -0.5839839591423000575, -79.42548989939000137, -1.474617623361999863 ) ) ;
#28417=CARTESIAN_POINT ( 'NONE',  ( -0.8981901762082999952, -79.85007741978999718, -1.403037214508999986 ) ) ;
#28420=CARTESIAN_POINT ( 'NONE',  ( -1.135826688880000157, -81.30663953507000485, -0.9797437077257000748 ) ) ;
#28424=CARTESIAN_POINT ( 'NONE',  ( -0.6296721830724527624, -81.01735300594884848, 1.093406895717950800 ) ) ;
#28427=CARTESIAN_POINT ( 'NONE',  ( -1.153358918101035524, -81.63163289808623801, -0.4816960858994225880 ) ) ;
#28446=VERTEX_POINT ( 'NONE', #46931 ) ;
#28457=CARTESIAN_POINT ( 'NONE',  ( 0.5769282351073999893, -80.98621153953999396, 1.350407801515999928 ) ) ;
#28473=DIRECTION ( 'NONE',  ( 0.000000000000000000, 0.000000000000000000, -1.000000000000000000 ) ) ;
#28486=CARTESIAN_POINT ( 'NONE',  ( -0.1807450410261203788, -81.98705298514224182, 1.237523090201967157 ) ) ;
#28491=CARTESIAN_POINT ( 'NONE',  ( 1.250000000000000222, -82.73958333333331439, -0.1636246173744659582 ) ) ;
#28512=CARTESIAN_POINT ( 'NONE',  ( 0.8982459645321505537, -82.78945047064037510, -0.8686774761259995481 ) ) ;
#28517=AXIS2_PLACEMENT_3D ( 'NONE', #16561, #52289, #19835 ) ;
#28536=CARTESIAN_POINT ( 'NONE',  ( 0.09741388862448860375, -82.96925805188962499, 1.246036882942684887 ) ) ;
#28544=CARTESIAN_POINT ( 'NONE',  ( -1.301142965806426632, -79.80676480095245040, 0.7731589486237497866 ) ) ;
#28569=ORIENTED_EDGE ( 'NONE', *, *, #3092, .F. ) ;
#28581=CARTESIAN_POINT ( 'NONE',  ( -1.156113623258839818, -80.56903096784071749, 0.4752053836311996848 ) ) ;
#28588=ORIENTED_EDGE ( 'NONE', *, *, #13535, .T. ) ;
#28592=CARTESIAN_POINT ( 'NONE',  ( -1.135996409638392768, -80.13451362626204855, -0.5214161241409958070 ) ) ;
#28595=CARTESIAN_POINT ( 'NONE',  ( 1.321891224999238723, -78.64195268641222469, 0.7850651250095550537 ) ) ;
#28612=CARTESIAN_POINT ( 'NONE',  ( -1.167146675921293397, -81.19530117510119283, 0.9583584161384303135 ) ) ;
#28614=CARTESIAN_POINT ( 'NONE',  ( -1.250000000000000000, -79.50000000000000000, 0.000000000000000000 ) ) ;
#28621=CARTESIAN_POINT ( 'NONE',  ( -1.232656909444999949, -82.61361845526398895, -0.5536498640889000455 ) ) ;
#28623=EDGE_LOOP ( 'NONE', ( #19713, #21050, #35759, #40045 ) ) ;
#28640=CARTESIAN_POINT ( 'NONE',  ( -0.3912638815494142719, -81.50038330625253025, 1.190242956311802214 ) ) ;
#28646=CARTESIAN_POINT ( 'NONE',  ( 1.075065877797000136, -78.28180136235999953, -0.7449938779133999933 ) ) ;
#28673=CARTESIAN_POINT ( 'NONE',  ( -1.472167250137000005, -78.92387186976999658, -0.6938203229310999642 ) ) ;
#28708=CARTESIAN_POINT ( 'NONE',  ( -0.6859742521509630819, -80.02179400559481337, 1.045181947014915069 ) ) ;
#28712=CARTESIAN_POINT ( 'NONE',  ( -1.603789611582999930, -80.35140824942999416, -0.4506860216877000558 ) ) ;
#28713=CARTESIAN_POINT ( 'NONE',  ( 0.1259833764099000109, -78.82466101900999433, 1.429058429169000055 ) ) ;
#28715=CARTESIAN_POINT ( 'NONE',  ( -1.338255681671218333, -81.71150629859762660, 0.7046537140460734649 ) ) ;
#28721=CARTESIAN_POINT ( 'NONE',  ( -1.057559559974387886, -81.64527973143721340, -0.6673670114133440912 ) ) ;
#28722=( LENGTH_UNIT ( ) NAMED_UNIT ( * ) SI_UNIT ( .MILLI., .METRE. ) );
#28749=CARTESIAN_POINT ( 'NONE',  ( -0.3234604031741999952, -79.66018296954999300, 1.671883997359000062 ) ) ;
#28753=CARTESIAN_POINT ( 'NONE',  ( -1.300212205372666130, -79.70741581913885909, 0.7726441571383775297 ) ) ;
#28768=AXIS2_PLACEMENT_3D ( 'NONE', #58336, #791, #35288 ) ;
#28769=CARTESIAN_POINT ( 'NONE',  ( 1.226351938740054770, -78.36563631113473605, 0.2418696441422709953 ) ) ;
#28786=CARTESIAN_POINT ( 'NONE',  ( 0.1636246173744697330, -82.63541666666665719, -1.249999999999999778 ) ) ;
#28807=ORIENTED_EDGE ( 'NONE', *, *, #19715, .F. ) ;
#28809=CARTESIAN_POINT ( 'NONE',  ( -1.406533682220601156, -78.22053972881499817, 0.5448426528144166836 ) ) ;
#28826=CARTESIAN_POINT ( 'NONE',  ( 0.01044744366229730971, -82.97494249513464126, 1.249636124618067834 ) ) ;
#28852=EDGE_CURVE ( 'NONE', #15598, #42991, #48259, .T. ) ;
#28854=AXIS2_PLACEMENT_3D ( 'NONE', #34358, #47692, #34647 ) ;
#28872=CARTESIAN_POINT ( 'NONE',  ( -0.5074500732423817828, -80.50838598281532654, 1.142332835001032887 ) ) ;
#28883=CARTESIAN_POINT ( 'NONE',  ( -2.500000000000000000, -77.69999999999998863, 0.000000000000000000 ) ) ;
#28887=CARTESIAN_POINT ( 'NONE',  ( 1.407449402687491524, -79.07027855378979098, -0.5447420947246425227 ) ) ;
#28905=CARTESIAN_POINT ( 'NONE',  ( -1.225487488653999923, -83.53778917074799892, -0.2866612609456000160 ) ) ;
#28909=CARTESIAN_POINT ( 'NONE',  ( -0.7681833999686477066, -82.92708333333331439, 0.9995835529977223910 ) ) ;
#28922=CARTESIAN_POINT ( 'NONE',  ( -0.5750802367077204602, -79.18702307077883518, -1.109883865317614848 ) ) ;
#28934=CARTESIAN_POINT ( 'NONE',  ( -0.0008345804459809217030, -81.47557856639851082, 1.249685689776924624 ) ) ;
#28963=CARTESIAN_POINT ( 'NONE',  ( -1.500000000000000000, -83.34999999999999432, 0.000000000000000000 ) ) ;
#28965=UNCERTAINTY_MEASURE_WITH_UNIT (LENGTH_MEASURE( 1.000000000000000082E-05 ), #28722, 'distance_accuracy_value', 'NONE');
#28969=CARTESIAN_POINT ( 'NONE',  ( -0.9156221410628999635, -78.31137460220000435, 1.345473579290000110 ) ) ;
#28978=CARTESIAN_POINT ( 'NONE',  ( 1.676986109946000170, -79.59391447301999278, 0.2957349343760000138 ) ) ;
#28990=FACE_OUTER_BOUND ( 'NONE', #25929, .T. ) ;
#29007=CARTESIAN_POINT ( 'NONE',  ( -0.1123201243897108126, -79.98247754429688428, 1.245149161110058689 ) ) ;
#29015=CARTESIAN_POINT ( 'NONE',  ( 0.9655056220227854480, -81.56980293136361126, 1.162965503173076121 ) ) ;
#29017=CARTESIAN_POINT ( 'NONE',  ( 0.9433681713884025655, -79.79331829884100102, -0.8205418275783242787 ) ) ;
#29022=CARTESIAN_POINT ( 'NONE',  ( 0.0005350743312633779144, -81.72561961952891352, -1.249649688976135931 ) ) ;
#29024=CARTESIAN_POINT ( 'NONE',  ( -1.072417187047447484, -81.45601597663524274, -0.9250971790290343222 ) ) ;
#29046=CARTESIAN_POINT ( 'NONE',  ( 0.3271848554490964789, -79.85416666666667140, 1.217465845835395521 ) ) ;
#29049=CARTESIAN_POINT ( 'NONE',  ( 0.4542139134408000323, -80.35477686209999604, -1.519238769708999959 ) ) ;
#29051=CARTESIAN_POINT ( 'NONE',  ( -1.238772947848447270, -79.79851084093215263, -0.8634107199282021750 ) ) ;
#29065=CARTESIAN_POINT ( 'NONE',  ( 0.2047640445682097077, -78.46198029154169262, 1.235340249920343858 ) ) ;
#29070=ADVANCED_FACE ( 'NONE', ( #44658 ), #9264, .F. ) ;
#29105=CARTESIAN_POINT ( 'NONE',  ( -0.3822735262362919051, -79.14481419606127588, 1.483096551402029339 ) ) ;
#29112=CARTESIAN_POINT ( 'NONE',  ( 0.01010140970966217668, -81.22383189636278189, 1.534624794271530313 ) ) ;
#29122=CARTESIAN_POINT ( 'NONE',  ( 0.3322227578772471435, -82.95365193092793277, 1.205740489271630356 ) ) ;
#29124=CARTESIAN_POINT ( 'NONE',  ( -0.9995835529977281642, -80.44791666666664298, 0.7681833999686391579 ) ) ;
#29145=CARTESIAN_POINT ( 'NONE',  ( -0.6811744818814000624, -82.48030346844899441, -1.520282978132999840 ) ) ;
#29155=CARTESIAN_POINT ( 'NONE',  ( -0.4458096168708076679, -80.69702831834133860, -1.185855554560490965 ) ) ;
#29160=ORIENTED_EDGE ( 'NONE', *, *, #18038, .T. ) ;
#29163=CARTESIAN_POINT ( 'NONE',  ( 0.1941027164032131103, -80.46307531212140418, 1.234895603396590991 ) ) ;
#29167=ORIENTED_EDGE ( 'NONE', *, *, #15907, .T. ) ;
#29178=CARTESIAN_POINT ( 'NONE',  ( 1.467401882609930430, -78.62410577527140276, 0.4599864963736973733 ) ) ;
#29191=CARTESIAN_POINT ( 'NONE',  ( -1.545693644023152125, -80.25398594989877665, -0.08651074858955706826 ) ) ;
#29195=CARTESIAN_POINT ( 'NONE',  ( 0.000000000000000000, -77.50000000000000000, 0.000000000000000000 ) ) ;
#29202=CARTESIAN_POINT ( 'NONE',  ( 0.4274279416557000277, -82.92941453081499503, 1.281884980902999960 ) ) ;
#29213=VERTEX_POINT ( 'NONE', #18530 ) ;
#29218=CARTESIAN_POINT ( 'NONE',  ( 0.1243710621956479329, -81.46772713155802137, 1.245975140190170194 ) ) ;
#29224=CARTESIAN_POINT ( 'NONE',  ( -0.9051267565814000715, -79.01584333927000614, 0.9442094098902999999 ) ) ;
#29237=AXIS2_PLACEMENT_3D ( 'NONE', #41438, #157, #54444 ) ;
#29254=CARTESIAN_POINT ( 'NONE',  ( 0.3877229342594999961, -78.03296675330000198, -1.580612325761999948 ) ) ;
#29261=CARTESIAN_POINT ( 'NONE',  ( -0.4591954515747000420, -81.72675258327998904, 1.639803156192000122 ) ) ;
#29262=CARTESIAN_POINT ( 'NONE',  ( -1.666294527194000175, -79.84655133345999900, -0.3511123450079000063 ) ) ;
#29290=CARTESIAN_POINT ( 'NONE',  ( -0.9022118396650773420, -80.03964887368034908, 0.8648181855745056268 ) ) ;
#29297=CARTESIAN_POINT ( 'NONE',  ( -0.7635483339353790200, -81.93231960672001435, -1.306464905284852263 ) ) ;
#29298=CARTESIAN_POINT ( 'NONE',  ( 0.7731065358596024284, -79.77859623460356886, -0.9850382754349712444 ) ) ;
#29304=ADVANCED_FACE ( 'NONE', ( #5518 ), #5809, .F. ) ;
#29305=ORIENTED_EDGE ( 'NONE', *, *, #31790, .F. ) ;
#29330=CARTESIAN_POINT ( 'NONE',  ( -0.6472661464068000248, -81.17600413218998767, 1.575051776950999960 ) ) ;
#29333=CARTESIAN_POINT ( 'NONE',  ( 1.362698812343641652, -79.46449576102331491, -0.6541207564315330014 ) ) ;
#29349=CARTESIAN_POINT ( 'NONE',  ( 1.017054994240753851, -78.39947633289455098, 0.7277666091791081815 ) ) ;
#29357=CARTESIAN_POINT ( 'NONE',  ( -1.250000000000000000, -79.59999999999999432, 0.000000000000000000 ) ) ;
#29361=CARTESIAN_POINT ( 'NONE',  ( -1.017084552132891728, -82.05124430433711780, 0.7286258421704788768 ) ) ;
#29368=CARTESIAN_POINT ( 'NONE',  ( -1.250000000000000000, -76.75499999999999545, 0.000000000000000000 ) ) ;
#29385=CARTESIAN_POINT ( 'NONE',  ( 0.07626174556372275481, -82.73051772784693014, -1.247420650239736251 ) ) ;
#29391=CARTESIAN_POINT ( 'NONE',  ( 1.341660107401375646, -78.53983454477609882, 0.7399033773893253230 ) ) ;
#29409=CARTESIAN_POINT ( 'NONE',  ( -0.01036771288394258174, -82.97628653625926631, 1.249625640293676732 ) ) ;
#29412=CARTESIAN_POINT ( 'NONE',  ( -0.3271848554491046945, -80.39583333333331439, 1.217465845835393301 ) ) ;
#29432=CARTESIAN_POINT ( 'NONE',  ( 1.531359430757999851, -82.60662189866998517, -0.6558942768039000004 ) ) ;
#29445=CARTESIAN_POINT ( 'NONE',  ( -0.4867589087424958327, -80.50691733354545931, 1.151273400566878324 ) ) ;
#29474=CARTESIAN_POINT ( 'NONE',  ( -0.7681833999686432657, -78.57291666666668561, -0.9995835529977258327 ) ) ;
#29476=CARTESIAN_POINT ( 'NONE',  ( -1.319810957934479445, -80.70946105886535804, 0.7378495871194835631 ) ) ;
#29508=CARTESIAN_POINT ( 'NONE',  ( 0.2887706833722973876, -81.45697567580890563, 1.216636297542402767 ) ) ;
#29536=CARTESIAN_POINT ( 'NONE',  ( -0.2201363562291999698, -79.46327907014000402, -1.483758735329000045 ) ) ;
#29542=CARTESIAN_POINT ( 'NONE',  ( -1.481905647302000029, -78.42273774175998824, -0.6727694308694001091 ) ) ;
#29545=EDGE_CURVE ( 'NONE', #41153, #19814, #201, .T. ) ;
#29552=CARTESIAN_POINT ( 'NONE',  ( 1.447659443890000119, -81.10989310931999796, -0.6470525719642999940 ) ) ;
#29565=CYLINDRICAL_SURFACE ( 'NONE', #25537, 1.250000000000000000 ) ;
#29577=CARTESIAN_POINT ( 'NONE',  ( -0.05067031697304230642, -79.97863705871390039, 1.248890127844249243 ) ) ;
#29583=CARTESIAN_POINT ( 'NONE',  ( -1.431540077043731873, -82.82304749526281284, 0.4904972203789410012 ) ) ;
#29585=CARTESIAN_POINT ( 'NONE',  ( -0.07293566597372513893, -79.72091539213137423, -1.249663842961500571 ) ) ;
#29604=VECTOR ( 'NONE', #56985, 1000.000000000000114 ) ;
#29609=B_SPLINE_CURVE_WITH_KNOTS ( 'NONE', 3,
 ( #40728, #4117, #41019, #53722, #30959, #44863, #54016, #49293, #9143, #8844, #57845, #40127, #319, #5004, #23008, #49891, #26835, #27128, #12682, #4416, #35386, #13557, #45461, #22715, #9435, #17402, #35694, #8257, #611, #22418, #18592, #40430, #21827, #58140, #39832, #36291, #48711, #13260, #53133, #13853, #45166, #48997, #54313, #22118, #31251, #26256, #4716, #21, #18001, #31849, #44270, #53415, #12962, #8544, #26536, #44563, #24175, #6165, #19458, #23586, #37454, #1469, #18876, #10314, #37750, #55772, #42191, #1760, #33013, #14431, #46637, #5575, #19754, #37164, #14141, #894, #36870, #50180, #36582, #28293, #10024, #54604, #55473, #55177, #46345, #32426, #28592, #15319, #32141, #28002, #46051, #9726, #15019, #1180, #33313, #50472, #27714 ),
 .UNSPECIFIED., .F., .F.,
 ( 4, 2, 2, 2, 1, 1, 1, 2, 2, 2, 2, 2, 1, 1, 1, 2, 2, 2, 2, 2, 1, 1, 1, 2, 2, 2, 2, 2, 1, 1, 1, 2, 2, 2, 2, 2, 1, 1, 1, 2, 2, 2, 2, 2, 1, 1, 1, 2, 2, 2, 2, 2, 1, 1, 1, 2, 2, 2, 4 ),
 ( 0.000000000000000000, 0.06249999999989072630, 0.09374999999983574250, 0.1093749999998082506, 0.1171874999997942757, 0.1210937499997875449, 0.1230468749997841726, 0.1240234374997827155, 0.1249999999997812583, 0.1874999999996865008, 0.2187499999996390665, 0.2343749999996153355, 0.2421874999996037059, 0.2460937499995978495, 0.2480468749995949074, 0.2490234374995934641, 0.2499999999995919930, 0.3124999999994510502, 0.3437499999993806066, 0.3593749999993457456, 0.3671874999993280375, 0.3710937499993191557, 0.3730468749993147703, 0.3740234374993125499, 0.3749999999993103295, 0.4374999999993330890, 0.4687499999993448574, 0.4843749999993509636, 0.4921874999993540167, 0.4960937499993555710, 0.4980468749993561817, 0.4990234374993564592, 0.4999999999993567368, 0.5624999999993588462, 0.5937499999993598454, 0.6093749999993606226, 0.6171874999993607336, 0.6210937499993607336, 0.6230468749993607336, 0.6240234374993610666, 0.6249999999993612887, 0.6874999999994607647, 0.7187499999995101696, 0.7343749999995347055, 0.7421874999995472511, 0.7460937499995535793, 0.7480468749995566879, 0.7490234374995581312, 0.7499999999995596855, 0.8124999999996873612, 0.8437499999997515321, 0.8593749999997836175, 0.8671874999997996047, 0.8710937499998074873, 0.8730468749998111511, 0.8740234374998130384, 0.8749999999998148148, 0.9374999999999074074, 1.000000000000000000 ),
 .UNSPECIFIED. ) ;
#29616=CARTESIAN_POINT ( 'NONE',  ( 1.349451115848000038, -79.91266235632998871, -0.8326934693224998796 ) ) ;
#29621=CARTESIAN_POINT ( 'NONE',  ( -0.6605212418366763760, -79.83899751728472438, -1.359602850557828591 ) ) ;
#29633=CARTESIAN_POINT ( 'NONE',  ( -10.05000000000000071, -87.20000000000000284, 0.000000000000000000 ) ) ;
#29636=CARTESIAN_POINT ( 'NONE',  ( 0.5914329913499263291, -78.43615203708624506, 1.104891015251897368 ) ) ;
#29647=B_SPLINE_CURVE_WITH_KNOTS ( 'NONE', 3,
 ( #41819, #12961, #19389, #14941, #30958, #48996, #8543, #26535, #44562, #42118, #43280, #34396, #24399, #16123, #29105, #38256, #52427, #20831, #38548, #15242, #55693, #11411, #24689, #42700, #20552, #37675, #33532, #33234, #51279, #2265, #7260, #20265, #34101, #56853, #6680, #56279, #46856, #11986, #16412, #15829, #33817, #52141, #51856, #29391, #47438, #6968, #42993, #24972, #10833, #51569, #11127, #46566, #2549, #19978, #56562, #11700, #6090, #29676, #28809, #42413, #24099, #47726, #25261, #1685, #2834, #38838, #1983, #6385, #19675, #37964, #55990, #15537, #47149, #25836, #26697, #44429, #48581, #16702, #53287, #43864, #35556, #12833, #58306 ),
 .UNSPECIFIED., .F., .F.,
 ( 4, 2, 1, 2, 2, 2, 2, 2, 2, 2, 2, 2, 2, 2, 2, 2, 2, 1, 2, 2, 2, 2, 2, 2, 2, 2, 2, 2, 2, 1, 2, 2, 2, 2, 2, 2, 2, 2, 2, 2, 2, 2, 4 ),
 ( 0.000000000000000000, 0.01562499999999997918, 0.03124999999999995837, 0.04687499999999994449, 0.06249999999999993061, 0.07812499999999991673, 0.09374999999999991673, 0.1249999999999998890, 0.1562499999999998612, 0.1874999999999998612, 0.2187499999999998335, 0.2499999999999998335, 0.2812499999999998335, 0.3124999999999998335, 0.3281249999999998335, 0.3437499999999998335, 0.3593749999999997780, 0.3749999999999998335, 0.3906249999999998890, 0.4062499999999998890, 0.4374999999999998335, 0.4687499999999998335, 0.4999999999999997780, 0.5312499999999997780, 0.5624999999999996669, 0.5937499999999996669, 0.6249999999999995559, 0.6562499999999995559, 0.6718749999999995559, 0.6874999999999995559, 0.7031249999999995559, 0.7187499999999994449, 0.7343749999999994449, 0.7499999999999994449, 0.7812499999999995559, 0.8124999999999995559, 0.8437499999999996669, 0.8749999999999996669, 0.9062499999999997780, 0.9374999999999998890, 0.9687499999999998890, 0.9843749999999998890, 1.000000000000000000 ),
 .UNSPECIFIED. ) ;
#29648=CARTESIAN_POINT ( 'NONE',  ( -0.9121818130210588293, -82.04075852875078567, 0.8543134884758614156 ) ) ;
#29658=CARTESIAN_POINT ( 'NONE',  ( -0.7676956659902818281, -78.17301476101459912, -0.9990819215154366217 ) ) ;
#29671=CARTESIAN_POINT ( 'NONE',  ( -1.250000000000000000, -82.59999999999999432, 0.000000000000000000 ) ) ;
#29675=CARTESIAN_POINT ( 'NONE',  ( 0.2851276402532497700, -79.45731520756731925, 1.217241021790539390 ) ) ;
#29676=CARTESIAN_POINT ( 'NONE',  ( -1.489116662163645133, -78.23734471912871413, 0.2394897313045940002 ) ) ;
#29732=CARTESIAN_POINT ( 'NONE',  ( -0.8376080881386354093, -80.53392362615774402, 0.9306764106483600418 ) ) ;
#29756=CARTESIAN_POINT ( 'NONE',  ( -1.403374235224089883, -80.78031274248239413, -0.5631813226398475480 ) ) ;
#29758=CARTESIAN_POINT ( 'NONE',  ( 0.9995835529977233902, -79.30208333333332860, 0.7681833999686461523 ) ) ;
#29767=CARTESIAN_POINT ( 'NONE',  ( 1.358765745638999878, -82.42429828359199462, 0.5569594143531000352 ) ) ;
#29785=CARTESIAN_POINT ( 'NONE',  ( 0.2454699089725678463, -81.45983395354696199, 1.225829166526236191 ) ) ;
#29787=CARTESIAN_POINT ( 'NONE',  ( 1.520902128651999918, -81.10537593950999735, -0.6797894616744000196 ) ) ;
#29800=CARTESIAN_POINT ( 'NONE',  ( -1.414324776981999987, -78.13539177200999575, 0.1417646478728999959 ) ) ;
#29803=AXIS2_PLACEMENT_3D ( 'NONE', #17151, #47901, #17439 ) ;
#29819=ORIENTED_EDGE ( 'NONE', *, *, #25276, .T. ) ;
#29823=CARTESIAN_POINT ( 'NONE',  ( -0.6295237254636235624, -83.08333333333332860, -1.092232985442822990 ) ) ;
#29828=CARTESIAN_POINT ( 'NONE',  ( -0.9347040216968000026, -78.75329240633999461, 1.332288049216000081 ) ) ;
#29837=CARTESIAN_POINT ( 'NONE',  ( -0.8049692409160000839, -81.53111201704999189, -1.105758127848999850 ) ) ;
#29841=CARTESIAN_POINT ( 'NONE',  ( -0.6572886123566999972, -82.61845057239298740, 1.530761476772000140 ) ) ;
#29856=CARTESIAN_POINT ( 'NONE',  ( -1.508277812474833501, -79.34690567646997295, 0.05089315114023049147 ) ) ;
#29858=CARTESIAN_POINT ( 'NONE',  ( -1.250000000000000000, -80.49999999999998579, 0.000000000000000000 ) ) ;
#29862=VECTOR ( 'NONE', #42809, 1000.000000000000000 ) ;
#29864=CARTESIAN_POINT ( 'NONE',  ( -1.050857806474344569, -80.05454060933334404, 0.6785706715357363583 ) ) ;
#29872=CARTESIAN_POINT ( 'NONE',  ( 0.01078207265347602868, -82.97487611262788221, -1.511023810634444020 ) ) ;
#29873=CARTESIAN_POINT ( 'NONE',  ( -1.079840341978513862, -79.64263545050475557, -0.6301668656408577762 ) ) ;
#29883=CARTESIAN_POINT ( 'NONE',  ( -0.7284109703836757488, -77.80208333347505345, -1.265496004316788214 ) ) ;
#29921=CARTESIAN_POINT ( 'NONE',  ( 0.8677903656447200076, -78.41400833188230024, 0.8997504066187256289 ) ) ;
#29926=CARTESIAN_POINT ( 'NONE',  ( 9.950000000000001066, -86.20000000000000284, 0.000000000000000000 ) ) ;
#29933=CARTESIAN_POINT ( 'NONE',  ( 1.208156862686758704, -81.87077954161354398, 0.3220240808263279964 ) ) ;
#29960=EDGE_LOOP ( 'NONE', ( #4158, #4778, #25146, #44590 ) ) ;
#29963=CARTESIAN_POINT ( 'NONE',  ( 0.7373373228469349838, -79.42494015767908877, 1.010443065347468750 ) ) ;
#30010=ORIENTED_EDGE ( 'NONE', *, *, #31266, .F. ) ;
#30018=ORIENTED_EDGE ( 'NONE', *, *, #5513, .F. ) ;
#30020=CARTESIAN_POINT ( 'NONE',  ( 0.4217350494414291440, -80.44779469249306203, 1.176759651058753242 ) ) ;
#30034=CARTESIAN_POINT ( 'NONE',  ( -0.6235925192133262573, -77.75853058493544268, 1.374630246012743529 ) ) ;
#30045=CARTESIAN_POINT ( 'NONE',  ( 1.217465845835394855, -78.72916666666665719, -0.3271848554490981997 ) ) ;
#30046=PRODUCT_DEFINITION_FORMATION_WITH_SPECIFIED_SOURCE ( 'ANY', '', #49847, .NOT_KNOWN. ) ;
#30047=CARTESIAN_POINT ( 'NONE',  ( -1.510136601423560432, -80.74994773521794400, -0.0005225141870202556918 ) ) ;
#30051=EDGE_CURVE ( 'NONE', #5620, #34281, #7343, .T. ) ;
#30054=AXIS2_PLACEMENT_3D ( 'NONE', #38792, #3366, #16369 ) ;
#30057=CARTESIAN_POINT ( 'NONE',  ( -1.446479059201000172, -82.74025183280099327, -0.6496884318727998986 ) ) ;
#30071=DIRECTION ( 'NONE',  ( 0.000000000000000000, 1.000000000000000000, 0.000000000000000000 ) ) ;
#30076=CARTESIAN_POINT ( 'NONE',  ( -0.8906226101088000613, -79.34480369890998475, -1.206976125017999779 ) ) ;
#30080=CARTESIAN_POINT ( 'NONE',  ( -0.3279074862126110657, -82.20481765143225061, -1.218086081608457771 ) ) ;
#30090=CARTESIAN_POINT ( 'NONE',  ( -1.205073015186999941, -78.18782334179000770, -0.7537975966218000146 ) ) ;
#30095=VECTOR ( 'NONE', #8958, 1000.000000000000000 ) ;
#30109=CARTESIAN_POINT ( 'NONE',  ( -1.250000000000000000, -82.99999999999998579, 0.000000000000000000 ) ) ;
#30118=DIRECTION ( 'NONE',  ( -1.000000000000000000, 0.000000000000000000, 0.000000000000000000 ) ) ;
#30126=CARTESIAN_POINT ( 'NONE',  ( -0.6718767921597000869, -82.73730002504399295, 1.564735933714000105 ) ) ;
#30127=CARTESIAN_POINT ( 'NONE',  ( 1.340661125304000167, -81.17320979808999937, -0.5992281077721001159 ) ) ;
#30131=CARTESIAN_POINT ( 'NONE',  ( -0.8762103189736000219, -81.29210705507999535, -1.416501064863000092 ) ) ;
#30144=CARTESIAN_POINT ( 'NONE',  ( -0.4492251327744000156, -81.72633577836998597, 1.604198796042999753 ) ) ;
#30161=CARTESIAN_POINT ( 'NONE',  ( -0.1453150226336093476, -82.73195032484389344, 1.504369831130939472 ) ) ;
#30162=CARTESIAN_POINT ( 'NONE',  ( -0.3119967359391886408, -79.70551649949634054, -1.210739184258169399 ) ) ;
#30175=CARTESIAN_POINT ( 'NONE',  ( -0.3747936025892038003, -77.81510416683644848, -1.397875464054185501 ) ) ;
#30226=AXIS2_PLACEMENT_3D ( 'NONE', #15270, #2293, #10864 ) ;
#30229=CARTESIAN_POINT ( 'NONE',  ( 0.7437748020536760762, -81.92464731248038845, 1.006161971671994060 ) ) ;
#30230=CARTESIAN_POINT ( 'NONE',  ( 1.655661065614000060, -79.08779862992999199, 0.1622525715179000128 ) ) ;
#30244=EDGE_LOOP ( 'NONE', ( #36202, #37589, #39482 ) ) ;
#30266=AXIS2_PLACEMENT_3D ( 'NONE', #24081, #46840, #51840 ) ;
#30298=ORIENTED_EDGE ( 'NONE', *, *, #40266, .T. ) ;
#30301=ORIENTED_EDGE ( 'NONE', *, *, #21672, .F. ) ;
#30308=ORIENTED_EDGE ( 'NONE', *, *, #14364, .T. ) ;
#30310=CARTESIAN_POINT ( 'NONE',  ( 1.222648819026868727, -80.36782262874812943, 0.2742722701991916479 ) ) ;
#30335=CARTESIAN_POINT ( 'NONE',  ( -1.250000000000000000, -78.50000000000000000, 0.000000000000000000 ) ) ;
#30336=CARTESIAN_POINT ( 'NONE',  ( -0.1549237127504899669, -80.13252592084100456, 1.540935225050198198 ) ) ;
#30347=CARTESIAN_POINT ( 'NONE',  ( -1.368292558779000023, -82.61377592892299049, 0.5331262435804999811 ) ) ;
#30350=CARTESIAN_POINT ( 'NONE',  ( -0.6295237254636235624, -82.08333333333332860, -1.092232985442822990 ) ) ;
#30366=CARTESIAN_POINT ( 'NONE',  ( -0.5432945554243000519, -81.42511490629999571, -1.398152719143000100 ) ) ;
#30383=CARTESIAN_POINT ( 'NONE',  ( 0.0005244906250799999826, -77.76837078354999733, -1.421402001996999953 ) ) ;
#30402=AXIS2_PLACEMENT_3D ( 'NONE', #55850, #34544, #2706 ) ;
#30412=CARTESIAN_POINT ( 'NONE',  ( -1.158404848901380957, -83.06944763503472018, 0.4695662491237505565 ) ) ;
#30418=CARTESIAN_POINT ( 'NONE',  ( 0.7473949548134999343, -82.16886708904999637, 1.530103832088000049 ) ) ;
#30420=CARTESIAN_POINT ( 'NONE',  ( -0.7081060581029999801, -80.54161764699000514, -1.286481228505000018 ) ) ;
#30421=CARTESIAN_POINT ( 'NONE',  ( -1.250000000000000000, -78.00000000000000000, 2.658254822585999717E-14 ) ) ;
#30425=CARTESIAN_POINT ( 'NONE',  ( 1.484562552624000054, -81.92369920617998957, -0.7558657512595999828 ) ) ;
#30437=CARTESIAN_POINT ( 'NONE',  ( -0.5790013745696001024, -82.92636086546200147, -1.562055304842999925 ) ) ;
#30442=FACE_OUTER_BOUND ( 'NONE', #31163, .T. ) ;
#30445=CARTESIAN_POINT ( 'NONE',  ( 1.146533421241619388, -79.88288899934906340, 0.4975437065520775248 ) ) ;
#30451=CARTESIAN_POINT ( 'NONE',  ( 0.3513416744041613637, -81.99305105366586588, -1.471649999805617393 ) ) ;
#30484=CARTESIAN_POINT ( 'NONE',  ( 0.08338359222296000406, -79.34015964247998909, -1.538001148114999994 ) ) ;
#30509=CARTESIAN_POINT ( 'NONE',  ( 0.000000000000000000, -91.89999999999999147, 0.000000000000000000 ) ) ;
#30519=CARTESIAN_POINT ( 'NONE',  ( 1.096288133368404472, -81.89016418702514954, 0.6007765553674837555 ) ) ;
#30525=DIRECTION ( 'NONE',  ( 0.000000000000000000, 1.000000000000000000, 0.000000000000000000 ) ) ;
#30565=CARTESIAN_POINT ( 'NONE',  ( 1.249611939558153084, -82.85111090171837134, 0.007260609876616985064 ) ) ;
#30618=CARTESIAN_POINT ( 'NONE',  ( -0.03709510739890169162, -77.97269351862679798, -1.508447481417284575 ) ) ;
#30623=CARTESIAN_POINT ( 'NONE',  ( 1.249999999999999778, -83.26041666666665719, 0.1636246173744711763 ) ) ;
#30628=CARTESIAN_POINT ( 'NONE',  ( -0.3271848554491046945, -80.89583333333328596, 1.217465845835393301 ) ) ;
#30629=CARTESIAN_POINT ( 'NONE',  ( 0.4629760832825556838, -79.99908104961433253, -1.440305437130205313 ) ) ;
#30638=CARTESIAN_POINT ( 'NONE',  ( -1.289397738844999974, -81.16111398138998823, -0.2928510814055000355 ) ) ;
#30641=CARTESIAN_POINT ( 'NONE',  ( -1.333333333333333259, -83.14999999999999147, 0.000000000000000000 ) ) ;
#30656=CARTESIAN_POINT ( 'NONE',  ( 1.617840321509000034, -80.15798771285999180, 0.3973055507782000118 ) ) ;
#30670=CARTESIAN_POINT ( 'NONE',  ( 1.076318381221999854, -78.44998119068999642, 0.9284129100290999803 ) ) ;
#30681=EDGE_CURVE ( 'NONE', #26523, #30955, #2214, .T. ) ;
#30698=CARTESIAN_POINT ( 'NONE',  ( -1.168994172860275071, -83.07126995735822561, 0.4429671410178434576 ) ) ;
#30701=CARTESIAN_POINT ( 'NONE',  ( -0.8340143124269999708, -81.47427319649999333, -1.348286063383000055 ) ) ;
#30702=CARTESIAN_POINT ( 'NONE',  ( 0.5128916439544000117, -81.11005058297999426, -1.376005298375999830 ) ) ;
#30706=CARTESIAN_POINT ( 'NONE',  ( -1.588687380433000174, -83.24609983225398935, 0.5002921117598999601 ) ) ;
#30713=CARTESIAN_POINT ( 'NONE',  ( -0.1834469635243000107, -79.61327907013999550, -1.236465612773999911 ) ) ;
#30717=CARTESIAN_POINT ( 'NONE',  ( -1.462746796095000024, -81.28816416383999410, -0.3322225316158000097 ) ) ;
#30727=CARTESIAN_POINT ( 'NONE',  ( 0.4578503181340247696, -79.94544045178886904, 1.162965988986303767 ) ) ;
#30733=CARTESIAN_POINT ( 'NONE',  ( 0.9661584243600921384, -81.66915000328793894, 1.163803266013009097 ) ) ;
#30740=DIRECTION ( 'NONE',  ( 0.000000000000000000, -1.000000000000000000, 0.000000000000000000 ) ) ;
#30741=ORIENTED_EDGE ( 'NONE', *, *, #53680, .T. ) ;
#30763=CARTESIAN_POINT ( 'NONE',  ( -0.6794254437148999903, -78.80190446794000536, -1.478865823597000029 ) ) ;
#30766=CARTESIAN_POINT ( 'NONE',  ( -0.7681833999686432657, -78.07291666666668561, -0.9995835529977258327 ) ) ;
#30788=FACE_OUTER_BOUND ( 'NONE', #39467, .T. ) ;
#30802=CARTESIAN_POINT ( 'NONE',  ( 0.5036000104604843042, -81.94200777690970483, 1.144331684476223909 ) ) ;
#30803=CARTESIAN_POINT ( 'NONE',  ( -1.419508297042999967, -77.92612078354999028, -0.6202052238666999617 ) ) ;
#30805=CARTESIAN_POINT ( 'NONE',  ( -0.1451771616029145784, -82.63257818562124157, 1.503302264768924257 ) ) ;
#30811=CARTESIAN_POINT ( 'NONE',  ( 0.5288604877964585560, -81.75996230616158300, -1.132634026371601044 ) ) ;
#30885=B_SPLINE_CURVE_WITH_KNOTS ( 'NONE', 3,
 ( #23731, #41742, #1319, #19313, #14863, #16622, #29883, #30175, #47939, #38471 ),
 .UNSPECIFIED., .F., .F.,
 ( 4, 2, 2, 2, 4 ),
 ( 0.000000000000000000, 0.1250000001980599851, 0.2500000003961199702, 0.3750000005941799275, 0.5000000007922399403 ),
 .UNSPECIFIED. ) ;
#30899=FACE_OUTER_BOUND ( 'NONE', #26832, .T. ) ;
#30913=CARTESIAN_POINT ( 'NONE',  ( 1.480842118789938100, -80.57602979559986522, -0.4564364147450694631 ) ) ;
#30922=EDGE_LOOP ( 'NONE', ( #4561, #52704, #57603, #25535 ) ) ;
#30941=EDGE_CURVE ( 'NONE', #12936, #35380, #34272, .T. ) ;
#30950=ORIENTED_EDGE ( 'NONE', *, *, #13889, .F. ) ;
#30954=CARTESIAN_POINT ( 'NONE',  ( -0.07270704760602998695, -78.82788729812999406, -1.533131890934999797 ) ) ;
#30955=VERTEX_POINT ( 'NONE', #12142 ) ;
#30958=CARTESIAN_POINT ( 'NONE',  ( -1.072066298137815732, -79.31286409919876235, -1.082357936291675538 ) ) ;
#30959=CARTESIAN_POINT ( 'NONE',  ( 1.222783487291517757, -80.33365183381954466, -0.2622213962109313790 ) ) ;
#30961=PRODUCT_DEFINITION_CONTEXT ( 'detailed design', #54170, 'design' ) ;
#30985=CARTESIAN_POINT ( 'NONE',  ( 1.533821497824999991, -81.66375084183000865, 0.4022281561003999695 ) ) ;
#30987=CARTESIAN_POINT ( 'NONE',  ( 0.3265465218672000125, -80.09950314121999781, -1.431717670164000200 ) ) ;
#31005=CARTESIAN_POINT ( 'NONE',  ( -0.6811744818814000624, -82.42108714457998531, -1.520282978132999840 ) ) ;
#31013=CARTESIAN_POINT ( 'NONE',  ( 0.4724532946902580410, -79.94440778530983494, 1.157109430825660867 ) ) ;
#31019=CARTESIAN_POINT ( 'NONE',  ( -1.135826688880000157, -81.40663953506998496, -0.9797437077257000748 ) ) ;
#31039=CARTESIAN_POINT ( 'NONE',  ( -0.4018693904811616591, -79.50120578641283942, 1.186371210911240759 ) ) ;
#31049=CARTESIAN_POINT ( 'NONE',  ( -0.6580604922749000441, -79.30303859595998972, -1.488334326434000099 ) ) ;
#31050=B_SPLINE_CURVE_WITH_KNOTS ( 'NONE', 3,
 ( #35148, #8304, #26304, #3874 ),
 .UNSPECIFIED., .F., .F.,
 ( 4, 4 ),
 ( 0.000000000000000000, 1.000000000000000000 ),
 .UNSPECIFIED. ) ;
#31081=DIRECTION ( 'NONE',  ( 1.000000000000000000, 0.000000000000000000, 0.000000000000000000 ) ) ;
#31086=CARTESIAN_POINT ( 'NONE',  ( 0.1378349583326383687, -81.96685064740351834, 1.242146068417951499 ) ) ;
#31087=CARTESIAN_POINT ( 'NONE',  ( 0.1658659358825000096, -77.75907607421000023, 1.418096705561000093 ) ) ;
#31089=CARTESIAN_POINT ( 'NONE',  ( -0.1834284358448134977, -82.86537657464923257, -1.499716752024290889 ) ) ;
#31094=CARTESIAN_POINT ( 'NONE',  ( 1.166166863406513210, -81.82083417477375065, -0.4499332933408479729 ) ) ;
#31100=AXIS2_PLACEMENT_3D ( 'NONE', #27851, #5428, #55908 ) ;
#31102=VERTEX_POINT ( 'NONE', #49029 ) ;
#31112=ORIENTED_EDGE ( 'NONE', *, *, #56593, .T. ) ;
#31156=CARTESIAN_POINT ( 'NONE',  ( -1.092232985442824100, -82.45833333333330017, 0.6295237254636200097 ) ) ;
#31163=EDGE_LOOP ( 'NONE', ( #57066, #2607, #16976, #27115 ) ) ;
#31202=CARTESIAN_POINT ( 'NONE',  ( -1.092633038097045262, -80.78858985991051611, 1.044221283387572807 ) ) ;
#31203=CARTESIAN_POINT ( 'NONE',  ( -0.4442664572140017087, -78.50400959573080684, 1.174863755326367221 ) ) ;
#31212=CARTESIAN_POINT ( 'NONE',  ( -0.8340143124269999708, -81.28758988526999474, -1.348286063383000055 ) ) ;
#31213=B_SPLINE_CURVE_WITH_KNOTS ( 'NONE', 3,
 ( #17652, #9092, #31501, #48950, #13508, #49547, #49242, #27081, #31801, #4063, #4671, #40682, #54266, #22067, #35640, #31203, #49844, #9390, #22964, #40974, #18543, #36535, #54559, #11372, #6344, #10789, #15789, #47108, #11086, #42657, #1646, #29065, #56524, #6639, #6927, #15200, #42952, #11943, #42372, #29636, #24645, #24359, #19933, #19635, #16371, #1940, #16083, #2224, #38509, #20791, #29921, #34063, #34352, #47688, #33490, #29349, #52389, #37923, #38794, #52101, #20226, #42076, #20512, #55948, #51237, #51529, #47971, #38217, #15498, #28769, #7216, #56239, #33777, #7508, #11659, #56814, #51817, #47395 ),
 .UNSPECIFIED., .F., .F.,
 ( 4, 2, 2, 2, 2, 2, 2, 2, 2, 2, 2, 2, 1, 1, 1, 2, 2, 2, 2, 2, 1, 2, 2, 2, 2, 2, 2, 1, 2, 2, 2, 2, 2, 2, 2, 1, 2, 2, 2, 2, 2, 4 ),
 ( 0.000000000000000000, 0.1249999999998231415, 0.1874999999997343791, 0.2187499999996899980, 0.2343749999996676270, 0.2421874999996563860, 0.2499999999996451727, 0.3124999999995554667, 0.3749999999994657607, 0.4374999999993760547, 0.4687499999993312016, 0.4843749999993087196, 0.4921874999992975064, 0.4960937499992897348, 0.4980468749992857935, 0.4990234374992869038, 0.4999999999992880140, 0.5624999999993739452, 0.5937499999994173550, 0.6015624999994276800, 0.6093749999994378941, 0.6249999999994585442, 0.6874999999995418110, 0.7031249999995625721, 0.7187499999995833333, 0.7343749999996040945, 0.7382812499996094235, 0.7421874999996148636, 0.7499999999996260769, 0.7812499999996731503, 0.8124999999997201128, 0.8437499999997671862, 0.8749999999998142597, 0.8906249999998374633, 0.8945312499998431255, 0.8984374999998487876, 0.9062499999998611111, 0.9374999999999086286, 0.9453124999999201750, 0.9531249999999316103, 0.9687499999999545919, 1.000000000000000000 ),
 .UNSPECIFIED. ) ;
#31228=LINE ( 'NONE', #26232, #22943 ) ;
#31232=CARTESIAN_POINT ( 'NONE',  ( 0.4771943503223999850, -80.53694300351999402, -1.596102929133000004 ) ) ;
#31243=VERTEX_POINT ( 'NONE', #13584 ) ;
#31247=CARTESIAN_POINT ( 'NONE',  ( 0.8811371538135999160, -78.88031886790999181, -1.256732680173000105 ) ) ;
#31251=CARTESIAN_POINT ( 'NONE',  ( 0.1620520141055530050, -80.23568876084854651, -1.239762908316072387 ) ) ;
#31266=EDGE_CURVE ( 'NONE', #25387, #10013, #31536, .T. ) ;
#31272=CARTESIAN_POINT ( 'NONE',  ( 0.000000000000000000, -76.75499999999999545, 0.000000000000000000 ) ) ;
#31277=CARTESIAN_POINT ( 'NONE',  ( 0.3489451476548999787, -81.60074910037999985, -1.426530384489999914 ) ) ;
#31278=CARTESIAN_POINT ( 'NONE',  ( -0.7224186015757000368, -79.59438689399999589, -0.9790252285018000711 ) ) ;
#31305=CARTESIAN_POINT ( 'NONE',  ( 1.250000000000000000, -79.84999999999999432, 0.000000000000000000 ) ) ;
#31326=CARTESIAN_POINT ( 'NONE',  ( 0.1639602171826417543, -82.46524421910949343, 1.249637490365603343 ) ) ;
#31347=CARTESIAN_POINT ( 'NONE',  ( -1.250000000000000000, -78.00000000000000000, 2.658254822585999717E-14 ) ) ;
#31384=CARTESIAN_POINT ( 'NONE',  ( -1.514795774450999888, -78.36393822280000165, -0.6877011994091001279 ) ) ;
#31386=CARTESIAN_POINT ( 'NONE',  ( 1.347270232873278406, -82.54148316382753592, 0.7639118359693641835 ) ) ;
#31409=EDGE_CURVE ( 'NONE', #12786, #22441, #388, .T. ) ;
#31424=CARTESIAN_POINT ( 'NONE',  ( -0.7407245532275998912, -81.15447863951000329, -1.017507444502999903 ) ) ;
#31431=DIRECTION ( 'NONE',  ( -0.7071067811865474617, -0.7071067811865474617, -6.518272650013434745E-10 ) ) ;
#31491=CARTESIAN_POINT ( 'NONE',  ( 1.061928034666324239, -79.70442635671331288, -0.6832555422594198680 ) ) ;
#31499=CARTESIAN_POINT ( 'NONE',  ( -0.6252223470676733230, -80.94041847728219352, -1.378227358566912919 ) ) ;
#31501=CARTESIAN_POINT ( 'NONE',  ( -1.252361392338912749, -78.59141244381495994, 0.1411392993344418867 ) ) ;
#31511=CARTESIAN_POINT ( 'NONE',  ( -1.495211702480000016, -81.28774735892999104, -0.3395960383748000133 ) ) ;
#31532=CARTESIAN_POINT ( 'NONE',  ( 0.000000000000000000, -77.50000000000000000, 0.000000000000000000 ) ) ;
#31536=CIRCLE ( 'NONE', #46677, 9.000000000000000000 ) ;
#31546=CARTESIAN_POINT ( 'NONE',  ( -0.2514447808355999570, -78.15716200999000307, 1.629006369695999767 ) ) ;
#31571=ORIENTED_EDGE ( 'NONE', *, *, #21366, .T. ) ;
#31572=CARTESIAN_POINT ( 'NONE',  ( 0.5015714934020000237, -83.24273121958398747, 1.504246450876000063 ) ) ;
#31574=CARTESIAN_POINT ( 'NONE',  ( -1.214718215476999985, -80.98388962642000877, 0.5919720313516000365 ) ) ;
#31605=CARTESIAN_POINT ( 'NONE',  ( 9.000000000000000000, -92.39999999999999147, 0.000000000000000000 ) ) ;
#31625=CARTESIAN_POINT ( 'NONE',  ( -1.250000000000000000, -83.09999999999999432, 0.000000000000000000 ) ) ;
#31639=CARTESIAN_POINT ( 'NONE',  ( 0.1429208184976999974, -78.57917818882999939, 1.621183732314999792 ) ) ;
#31677=CARTESIAN_POINT ( 'NONE',  ( -0.8906226101088000613, -79.28558737503999509, -1.206976125017999779 ) ) ;
#31678=CARTESIAN_POINT ( 'NONE',  ( -0.9359438995330000566, -78.25257508323998934, 1.375335667459000044 ) ) ;
#31680=CARTESIAN_POINT ( 'NONE',  ( -1.508012578157784445, -82.75403821467907051, -0.07803458566731928669 ) ) ;
#31685=CARTESIAN_POINT ( 'NONE',  ( 1.249621047773330496, -81.84926137039978755, -0.02155140958586815314 ) ) ;
#31689=CARTESIAN_POINT ( 'NONE',  ( 0.000000000000000000, -76.75499999999999545, 0.000000000000000000 ) ) ;
#31697=CARTESIAN_POINT ( 'NONE',  ( 1.143767095131633660, -80.38318895732449221, 0.5041385401734318483 ) ) ;
#31750=CARTESIAN_POINT ( 'NONE',  ( 0.9995835529977233902, -82.30208333333331439, 0.7681833999686461523 ) ) ;
#31753=AXIS2_PLACEMENT_3D ( 'NONE', #33249, #1410, #46870 ) ;
#31759=CARTESIAN_POINT ( 'NONE',  ( -1.499999999971000086, -77.75000000002998490, -1.761798912373000190E-09 ) ) ;
#31790=EDGE_CURVE ( 'NONE', #7116, #13712, #613, .T. ) ;
#31800=CARTESIAN_POINT ( 'NONE',  ( 0.7543631752853537931, -80.51529834865404212, -1.353141125584138793 ) ) ;
#31801=CARTESIAN_POINT ( 'NONE',  ( -0.9772521179090640775, -78.54668683268188545, 0.7800898177333105421 ) ) ;
#31811=CARTESIAN_POINT ( 'NONE',  ( -0.7740797122817000275, -83.18252381223099690, 1.516913212488000040 ) ) ;
#31814=B_SPLINE_CURVE_WITH_KNOTS ( 'NONE', 3,
 ( #44524, #30641, #39514, #11795 ),
 .UNSPECIFIED., .F., .F.,
 ( 4, 4 ),
 ( 0.000000000000000000, 1.000000000000000000 ),
 .UNSPECIFIED. ) ;
#31845=CARTESIAN_POINT ( 'NONE',  ( -1.502510403038999964, -78.72302415856999858, -0.3134361142718999904 ) ) ;
#31849=CARTESIAN_POINT ( 'NONE',  ( 0.01540432062990471779, -80.22651900916568479, -1.249598698544762687 ) ) ;
#31856=VERTEX_POINT ( 'NONE', #28883 ) ;
#31871=CARTESIAN_POINT ( 'NONE',  ( -0.6004489902433000070, -82.54813732702999118, -1.340115349862999850 ) ) ;
#31873=CARTESIAN_POINT ( 'NONE',  ( -1.092232985442824100, -79.45833333333330017, 0.6295237254636200097 ) ) ;
#31889=CARTESIAN_POINT ( 'NONE',  ( -0.1834469635243000107, -79.21327907014000402, -1.236465612773999911 ) ) ;
#31898=CARTESIAN_POINT ( 'NONE',  ( -1.228243686087402642, -81.58562147598921399, 0.2329788977900838498 ) ) ;
#31918=CARTESIAN_POINT ( 'NONE',  ( -0.6297930565811739045, -82.51732734865008467, 1.093430612505388311 ) ) ;
#31932=CARTESIAN_POINT ( 'NONE',  ( -1.560595261880000084, -77.74748939621999000, 0.4619550309703999713 ) ) ;
#31934=ADVANCED_FACE ( 'NONE', ( #30899 ), #16478, .T. ) ;
#31956=DIRECTION ( 'NONE',  ( 0.000000000000000000, -1.000000000000000000, 0.000000000000000000 ) ) ;
#31970=CARTESIAN_POINT ( 'NONE',  ( -1.542698325316999908, -81.23958015220999584, 0.6290719308543000210 ) ) ;
#31971=CARTESIAN_POINT ( 'NONE',  ( 0.1781252944802999838, -77.69575938543998461, 1.522910005212999796 ) ) ;
#31973=CARTESIAN_POINT ( 'NONE',  ( 1.381772510957646194, -82.96659326553100300, -0.6148152531492157014 ) ) ;
#31984=CARTESIAN_POINT ( 'NONE',  ( 1.092232985442823212, -80.20833333333332860, -0.6295237254636224522 ) ) ;
#31987=DIRECTION ( 'NONE',  ( 0.000000000000000000, 1.000000000000000000, 0.000000000000000000 ) ) ;
#31990=ORIENTED_EDGE ( 'NONE', *, *, #46126, .F. ) ;
#32010=CARTESIAN_POINT ( 'NONE',  ( -1.468405992501000012, -81.17584665853000558, 0.5987774653158000060 ) ) ;
#32038=FACE_BOUND ( 'NONE', #3748, .T. ) ;
#32067=CARTESIAN_POINT ( 'NONE',  ( 1.234997842510089372, -82.83803313528682111, -0.1925883613549776718 ) ) ;
#32088=CARTESIAN_POINT ( 'NONE',  ( 1.250000000000000000, -79.73860658917831756, -0.1789672786810340421 ) ) ;
#32094=CARTESIAN_POINT ( 'NONE',  ( 0.6295237254636211199, -80.83333333333334281, 1.092232985442824322 ) ) ;
#32097=CARTESIAN_POINT ( 'NONE',  ( 0.7146743994145193790, -79.68530190706071892, 1.333844887466810292 ) ) ;
#32104=CARTESIAN_POINT ( 'NONE',  ( 1.413069887183999951, -81.91918203637000317, -0.7194652256120001033 ) ) ;
#32129=ORIENTED_EDGE ( 'NONE', *, *, #22513, .T. ) ;
#32130=CARTESIAN_POINT ( 'NONE',  ( -1.130640822228425435, -80.56483172200898935, 0.5346059543193828478 ) ) ;
#32136=CARTESIAN_POINT ( 'NONE',  ( -1.379901750132000116, -78.67059258879000083, 0.6720497516175000241 ) ) ;
#32141=CARTESIAN_POINT ( 'NONE',  ( -1.150140635162034908, -80.13221033398477289, -0.4892649414430590427 ) ) ;
#32164=CARTESIAN_POINT ( 'NONE',  ( 0.3271848554490964789, -82.85416666666665719, 1.217465845835395521 ) ) ;
#32182=EDGE_LOOP ( 'NONE', ( #58136, #19213, #47238, #53641, #39532, #50173, #23288, #33150, #53492, #24459, #47137 ) ) ;
#32187=CARTESIAN_POINT ( 'NONE',  ( -1.157498849743237246, -81.56938687382739772, 0.4716165995993014670 ) ) ;
#32220=LINE ( 'NONE', #5952, #20991 ) ;
#32222=CARTESIAN_POINT ( 'NONE',  ( -1.491326706514000122, -77.74395464212999229, -0.6515838025032999470 ) ) ;
#32236=CARTESIAN_POINT ( 'NONE',  ( -1.250013176831791695, -78.10006463709670754, 4.053087819277079897E-06 ) ) ;
#32257=CARTESIAN_POINT ( 'NONE',  ( -1.603789611582999930, -80.29219192556000451, -0.4506860216877000558 ) ) ;
#32258=CARTESIAN_POINT ( 'NONE',  ( -1.280656172315000063, -79.50047497536000662, 0.3202611811242000450 ) ) ;
#32260=CARTESIAN_POINT ( 'NONE',  ( 0.2394845634073196894, -81.38761288777696734, -1.493279160396979721 ) ) ;
#32262=CARTESIAN_POINT ( 'NONE',  ( 1.251175831454664156, -83.14694854564174875, 0.8506124265937500262 ) ) ;
#32268=CARTESIAN_POINT ( 'NONE',  ( -1.154629675336898531, -81.63141643927103530, -0.4786478767419468094 ) ) ;
#32271=FACE_OUTER_BOUND ( 'NONE', #26445, .T. ) ;
#32279=CARTESIAN_POINT ( 'NONE',  ( 9.500000000000000000, -91.89999999999999147, -7.290811810668999158E-14 ) ) ;
#32307=CARTESIAN_POINT ( 'NONE',  ( 1.092232985442823212, -79.20833333333331439, -0.6295237254636224522 ) ) ;
#32330=CARTESIAN_POINT ( 'NONE',  ( -1.249999999999999778, -82.51041666666662877, -0.1636246173744686228 ) ) ;
#32332=VERTEX_POINT ( 'NONE', #11416 ) ;
#32347=ADVANCED_FACE ( 'NONE', ( #38263 ), #38555, .F. ) ;
#32360=CARTESIAN_POINT ( 'NONE',  ( 1.250000000000000000, -83.24999999999998579, 0.000000000000000000 ) ) ;
#32364=VECTOR ( 'NONE', #13604, 1000.000000000000000 ) ;
#32403=ORIENTED_EDGE ( 'NONE', *, *, #45098, .T. ) ;
#32411=DIRECTION ( 'NONE',  ( 0.000000000000000000, 1.000000000000000000, 0.000000000000000000 ) ) ;
#32426=CARTESIAN_POINT ( 'NONE',  ( -1.127633102446787161, -80.13579083371682543, -0.5390502240130501388 ) ) ;
#32431=CARTESIAN_POINT ( 'NONE',  ( 0.5497657648701759214, -78.19577990788877742, 1.434553788796227858 ) ) ;
#32448=CARTESIAN_POINT ( 'NONE',  ( -1.183213148269000259, -81.97986186469999836, 0.6526699808710000328 ) ) ;
#32459=CARTESIAN_POINT ( 'NONE',  ( 0.000000000000000000, -76.75499999999999545, 0.000000000000000000 ) ) ;
#32466=CARTESIAN_POINT ( 'NONE',  ( 0.6799804141806697899, -79.27066170111446297, -1.062685189815249620 ) ) ;
#32476=ADVANCED_FACE ( 'NONE', ( #26705 ), #47532, .F. ) ;
#32478=CARTESIAN_POINT ( 'NONE',  ( -1.159531907918516458, -81.56974165474723293, 0.4665971513285117056 ) ) ;
#32487=ORIENTED_EDGE ( 'NONE', *, *, #9512, .T. ) ;
#32494=CARTESIAN_POINT ( 'NONE',  ( 1.093346996216985056, -82.39232783775085522, 0.6296573929790432178 ) ) ;
#32509=CARTESIAN_POINT ( 'NONE',  ( -0.1732310466989999687, -77.65468677991998447, 1.530487294790999986 ) ) ;
#32548=CARTESIAN_POINT ( 'NONE',  ( 1.417725061834000044, -79.91717952614000353, -0.8748226493128999914 ) ) ;
#32549=CARTESIAN_POINT ( 'NONE',  ( -0.8071124281214000495, -78.37920846078000636, 1.186022485533999804 ) ) ;
#32552=CARTESIAN_POINT ( 'NONE',  ( 1.394813767835870522, -81.46858624048219610, -0.5832741237438665571 ) ) ;
#32555=CARTESIAN_POINT ( 'NONE',  ( 1.159203040753797431, -79.81982044965684508, -0.4672302196274162878 ) ) ;
#32557=CARTESIAN_POINT ( 'NONE',  ( -1.134601249923181232, -81.63469519395181351, -0.5245280893132442390 ) ) ;
#32574=DIRECTION ( 'NONE',  ( 0.000000000000000000, 0.000000000000000000, -1.000000000000000000 ) ) ;
#32586=CARTESIAN_POINT ( 'NONE',  ( -1.494795747725999879, -80.73373215275999826, -0.5291335979940999801 ) ) ;
#32595=AXIS2_PLACEMENT_3D ( 'NONE', #15265, #32665, #50132 ) ;
#32603=EDGE_LOOP ( 'NONE', ( #57838, #55541, #186, #55874 ) ) ;
#32639=EDGE_LOOP ( 'NONE', ( #29305, #11056, #18283, #12886 ) ) ;
#32640=CARTESIAN_POINT ( 'NONE',  ( 1.249294810647472387, -82.84741769837783920, -0.04986753284709229822 ) ) ;
#32645=LINE ( 'NONE', #55694, #13302 ) ;
#32646=LINE ( 'NONE', #32360, #2911 ) ;
#32650=B_SPLINE_CURVE_WITH_KNOTS ( 'NONE', 3,
 ( #42308, #47044, #24585, #33429, #9847, #19285 ),
 .UNSPECIFIED., .F., .F.,
 ( 4, 2, 4 ),
 ( 0.000000000000000000, 0.4999999999999998890, 1.000000000000000000 ),
 .UNSPECIFIED. ) ;
#32662=CARTESIAN_POINT ( 'NONE',  ( 1.036004598597317639, -82.89747191575634133, 0.6991915507269829133 ) ) ;
#32664=DIRECTION ( 'NONE',  ( 0.000000000000000000, 1.000000000000000000, 0.000000000000000000 ) ) ;
#32665=DIRECTION ( 'NONE',  ( 0.000000000000000000, 1.000000000000000000, 0.000000000000000000 ) ) ;
#32668=DIRECTION ( 'NONE',  ( 0.000000000000000000, -1.000000000000000000, 0.000000000000000000 ) ) ;
#32669=CARTESIAN_POINT ( 'NONE',  ( 1.157527094954509117, -79.54359519752044605, -0.9749728451049136657 ) ) ;
#32679=ORIENTED_EDGE ( 'NONE', *, *, #41033, .F. ) ;
#32692=CARTESIAN_POINT ( 'NONE',  ( 1.571434226476000173, -83.11189561955099236, -0.5530452149683998675 ) ) ;
#32707=CARTESIAN_POINT ( 'NONE',  ( -0.9351132745867291041, -80.54278198314504777, 0.8292394773563549482 ) ) ;
#32722=CARTESIAN_POINT ( 'NONE',  ( 0.3846651997978238757, -79.20413038734237432, 1.459419617943195968 ) ) ;
#32740=CARTESIAN_POINT ( 'NONE',  ( -1.295013057735999951, -82.04302107981000347, -0.3858917059242000236 ) ) ;
#32769=CARTESIAN_POINT ( 'NONE',  ( -1.034407521427512133, -81.55267419125448214, 0.7041627674574237883 ) ) ;
#32799=CARTESIAN_POINT ( 'NONE',  ( -1.573065832928000063, -78.74975765224999691, 0.4172852021023999991 ) ) ;
#32811=CARTESIAN_POINT ( 'NONE',  ( -0.8211341099608999716, -80.41498426945000233, -1.491829658087999944 ) ) ;
#32827=EDGE_CURVE ( 'NONE', #28137, #48909, #35517, .T. ) ;
#32839=CARTESIAN_POINT ( 'NONE',  ( 1.551146335801999898, -81.16853515462000246, 0.6076261867840000441 ) ) ;
#32842=CARTESIAN_POINT ( 'NONE',  ( -0.8592827076548754661, -81.32688287324717180, -1.244672245808209787 ) ) ;
#32843=CARTESIAN_POINT ( 'NONE',  ( 0.3161824776153564498, -83.20767999258765713, 1.479864803184822497 ) ) ;
#32849=CARTESIAN_POINT ( 'NONE',  ( -0.6462729935705185946, -81.68201433982439141, -1.071111153078781353 ) ) ;
#32852=ORIENTED_EDGE ( 'NONE', *, *, #20823, .T. ) ;
#32878=CARTESIAN_POINT ( 'NONE',  ( -1.274573384913999963, -80.10198252799999352, 0.7293221697183999153 ) ) ;
#32884=CARTESIAN_POINT ( 'NONE',  ( 1.507312305499400207, -79.49486076828772241, -0.09857350602148712282 ) ) ;
#32887=DIRECTION ( 'NONE',  ( 0.000000000000000000, -1.000000000000000000, 1.134344766989000102E-14 ) ) ;
#32893=CARTESIAN_POINT ( 'NONE',  ( 0.7681833999686451531, -79.17708333333332860, -0.9995835529977240563 ) ) ;
#32917=VERTEX_POINT ( 'NONE', #35770 ) ;
#32925=VERTEX_POINT ( 'NONE', #49372 ) ;
#32931=EDGE_CURVE ( 'NONE', #34281, #7212, #7306, .T. ) ;
#32959=CARTESIAN_POINT ( 'NONE',  ( 1.148760496143379495, -82.88227549639147185, 0.4927867763867777029 ) ) ;
#32983=CARTESIAN_POINT ( 'NONE',  ( 1.431241028886999889, -81.53685813303999907, -0.8524881072380000591 ) ) ;
#32990=EDGE_CURVE ( 'NONE', #46203, #9574, #13681, .T. ) ;
#32995=DIRECTION ( 'NONE',  ( -1.000000000000000000, 0.000000000000000000, 0.000000000000000000 ) ) ;
#33013=CARTESIAN_POINT ( 'NONE',  ( -0.6633660878114170378, -80.18071131022675502, -1.060558990980815297 ) ) ;
#33017=CARTESIAN_POINT ( 'NONE',  ( 1.060894005001709495, -78.53487121956678152, -1.113722360277955792 ) ) ;
#33024=AXIS2_PLACEMENT_3D ( 'NONE', #4290, #54758, #35867 ) ;
#33034=CARTESIAN_POINT ( 'NONE',  ( 0.5930780265196999856, -82.35881715536000058, 1.214178601635999888 ) ) ;
#33037=CARTESIAN_POINT ( 'NONE',  ( -0.7681833999686477066, -78.92708333333332860, 0.9995835529977223910 ) ) ;
#33049=CIRCLE ( 'NONE', #30226, 10.14999999999999858 ) ;
#33069=CARTESIAN_POINT ( 'NONE',  ( -0.06195931011014999684, -78.70125392059999569, -1.306500503017999915 ) ) ;
#33084=CARTESIAN_POINT ( 'NONE',  ( 0.000000000000000000, -86.39999999999999147, 0.000000000000000000 ) ) ;
#33087=EDGE_CURVE ( 'NONE', #10113, #25256, #2328, .T. ) ;
#33098=CARTESIAN_POINT ( 'NONE',  ( 1.153380192234999990, -78.64192926678998674, 1.148206073167999941 ) ) ;
#33107=CARTESIAN_POINT ( 'NONE',  ( -0.5042965048037999498, -80.79409703377000085, 1.503356827960000031 ) ) ;
#33136=CARTESIAN_POINT ( 'NONE',  ( -0.4240539849974000464, -80.22508981920998394, 1.611036072322000079 ) ) ;
#33137=CARTESIAN_POINT ( 'NONE',  ( 1.429610420046000252, -78.71329787945998646, 0.1195568986375999954 ) ) ;
#33142=CARTESIAN_POINT ( 'NONE',  ( 1.033908640164241222, -79.80255683383327892, -0.7040647445706786911 ) ) ;
#33145=CARTESIAN_POINT ( 'NONE',  ( -0.8722640199205535794, -81.66406706422890238, -0.8949065950927366231 ) ) ;
#33148=DIRECTION ( 'NONE',  ( 0.000000000000000000, -1.000000000000000000, 0.000000000000000000 ) ) ;
#33150=ORIENTED_EDGE ( 'NONE', *, *, #11446, .F. ) ;
#33167=CARTESIAN_POINT ( 'NONE',  ( -0.9995835529977281642, -81.44791666666662877, 0.7681833999686391579 ) ) ;
#33173=CARTESIAN_POINT ( 'NONE',  ( 0.6904535216592000424, -79.91234740900999611, 1.161570125514999940 ) ) ;
#33176=CARTESIAN_POINT ( 'NONE',  ( -0.2201363562291999698, -79.36327907013999550, -1.483758735329000045 ) ) ;
#33179=EDGE_CURVE ( 'NONE', #48919, #54320, #11260, .T. ) ;
#33181=LINE ( 'NONE', #6628, #23092 ) ;
#33197=CARTESIAN_POINT ( 'NONE',  ( 0.000000000000000000, -76.75499999999999545, 0.000000000000000000 ) ) ;
#33201=CARTESIAN_POINT ( 'NONE',  ( -0.1437401157479178682, -81.98469811677230723, 1.242173127013889378 ) ) ;
#33228=CARTESIAN_POINT ( 'NONE',  ( 0.03738295792059419254, -82.72804728612686631, -1.249190724913706640 ) ) ;
#33234=CARTESIAN_POINT ( 'NONE',  ( -0.6025044293664234551, -78.84232437041447383, -1.382994520336419342 ) ) ;
#33237=CARTESIAN_POINT ( 'NONE',  ( 1.250000000000000000, -82.74999999999998579, 0.000000000000000000 ) ) ;
#33249=CARTESIAN_POINT ( 'NONE',  ( 0.000000000000000000, -76.75499999999999545, 0.000000000000000000 ) ) ;
#33255=CARTESIAN_POINT ( 'NONE',  ( 0.2897521468641586773, -82.95649998723895635, 1.216791426940023513 ) ) ;
#33280=CARTESIAN_POINT ( 'NONE',  ( -1.510823314100999903, -83.40663862339900447, -0.3534059060544000319 ) ) ;
#33300=CARTESIAN_POINT ( 'NONE',  ( 0.02072621771690125181, -80.47431364731653503, 1.249620385757917118 ) ) ;
#33313=CARTESIAN_POINT ( 'NONE',  ( -1.231052532977768843, -80.11508864318425083, -0.2330927567282044255 ) ) ;
#33317=CARTESIAN_POINT ( 'NONE',  ( 0.1356080529126781065, -78.48133048614386098, -1.532370771129643483 ) ) ;
#33332=ORIENTED_EDGE ( 'NONE', *, *, #43702, .F. ) ;
#33333=CARTESIAN_POINT ( 'NONE',  ( -1.115197308773999918, -81.55880043062998652, -0.5833774300368999022 ) ) ;
#33336=CARTESIAN_POINT ( 'NONE',  ( 0.3271848554490964789, -78.85416666666665719, 1.217465845835395521 ) ) ;
#33348=CARTESIAN_POINT ( 'NONE',  ( 0.7681833999686451531, -82.17708333333331439, -0.9995835529977240563 ) ) ;
#33352=CARTESIAN_POINT ( 'NONE',  ( -0.4021068579646576713, -79.19911756258647983, -1.186049746191630172 ) ) ;
#33368=CARTESIAN_POINT ( 'NONE',  ( 0.9904172874407001226, -78.38666450191999502, 0.8543161689128000447 ) ) ;
#33395=CARTESIAN_POINT ( 'NONE',  ( -0.7812014261399538029, -81.57275290714748905, -1.008111165206596160 ) ) ;
#33396=CARTESIAN_POINT ( 'NONE',  ( 0.1429208184976999974, -78.75682716043000653, 1.621183732314999792 ) ) ;
#33405=CARTESIAN_POINT ( 'NONE',  ( -0.4334656432294999862, -80.22550662411998701, 1.646792182271999971 ) ) ;
#33429=CARTESIAN_POINT ( 'NONE',  ( -1.223703478834903713, -81.11953203607674823, -0.2972330812242202080 ) ) ;
#33437=CARTESIAN_POINT ( 'NONE',  ( 0.1463366571038000052, -78.32352689100000021, 1.427117860474999889 ) ) ;
#33439=CARTESIAN_POINT ( 'NONE',  ( 1.541569372070112909, -81.99491303306574252, -0.1072605994430432114 ) ) ;
#33440=CARTESIAN_POINT ( 'NONE',  ( -0.7946115520685833600, -83.26841143953370761, 1.288064595800165524 ) ) ;
#33441=CARTESIAN_POINT ( 'NONE',  ( 0.8868842948722143182, -79.78821287788076688, -0.8805106682841317145 ) ) ;
#33442=CARTESIAN_POINT ( 'NONE',  ( 0.7678017030685237998, -80.92358540104676479, 0.9995472151052681165 ) ) ;
#33444=CARTESIAN_POINT ( 'NONE',  ( -1.107453414133191094, -81.63871445155162121, -0.5797266078115248522 ) ) ;
#33447=EDGE_LOOP ( 'NONE', ( #6726, #51621, #37428 ) ) ;
#33453=EDGE_LOOP ( 'NONE', ( #13695, #4075, #20261, #16051 ) ) ;
#33471=CARTESIAN_POINT ( 'NONE',  ( 0.2675321060165000153, -79.40754610911000100, -1.681415376183999832 ) ) ;
#33474=CARTESIAN_POINT ( 'NONE',  ( -1.064988270483648414, -79.68717248096253059, 1.072152466623225386 ) ) ;
#33490=CARTESIAN_POINT ( 'NONE',  ( 0.9905026783004660107, -78.40226506858486744, 0.7633233902531472159 ) ) ;
#33508=CARTESIAN_POINT ( 'NONE',  ( 1.250000000000000000, -78.85000000000000853, 0.000000000000000000 ) ) ;
#33516=CYLINDRICAL_SURFACE ( 'NONE', #30266, 1.250000000000000000 ) ;
#33532=CARTESIAN_POINT ( 'NONE',  ( -0.4522900895953318456, -78.85072686557104760, -1.438476364793949802 ) ) ;
#33550=CARTESIAN_POINT ( 'NONE',  ( 0.9737724313953866062, -82.90436024173828855, 0.7837087735941486999 ) ) ;
#33553=CARTESIAN_POINT ( 'NONE',  ( -1.250000000000001332, -80.48958333333332860, 0.1636246173744632659 ) ) ;
#33575=CARTESIAN_POINT ( 'NONE',  ( -0.7803569495551999635, -81.97502974756999095, -1.471836271561000054 ) ) ;
#33586=CYLINDRICAL_SURFACE ( 'NONE', #19995, 1.250000000000000000 ) ;
#33594=CARTESIAN_POINT ( 'NONE',  ( -0.4825602083052458746, -80.50662037162305751, 1.153044462113711033 ) ) ;
#33595=DIRECTION ( 'NONE',  ( 0.000000000000000000, -1.000000000000000000, 0.000000000000000000 ) ) ;
#33608=CARTESIAN_POINT ( 'NONE',  ( -1.530868492697737393, -78.85611562010234366, -0.1310416657043483035 ) ) ;
#33622=CARTESIAN_POINT ( 'NONE',  ( 1.237362355298573968, -80.05155256813580422, 0.9256756271965481675 ) ) ;
#33641=CARTESIAN_POINT ( 'NONE',  ( -0.5925039872731914237, -79.18577407509000921, -1.100617820668964741 ) ) ;
#33651=CARTESIAN_POINT ( 'NONE',  ( 1.152279072913166447, -81.38189058625292205, 0.4841459733426476952 ) ) ;
#33656=CARTESIAN_POINT ( 'NONE',  ( 0.6875379384163999852, -78.91098019970999644, 1.112687622202999771 ) ) ;
#33658=CARTESIAN_POINT ( 'NONE',  ( 1.217465845835393967, -78.27083333333332860, 0.3271848554491025851 ) ) ;
#33660=ORIENTED_EDGE ( 'NONE', *, *, #23091, .F. ) ;
#33662=ORIENTED_EDGE ( 'NONE', *, *, #30051, .F. ) ;
#33686=CARTESIAN_POINT ( 'NONE',  ( 0.1198033158700999995, -79.25796128845000510, 1.623056241665000066 ) ) ;
#33694=CARTESIAN_POINT ( 'NONE',  ( -0.8692139286044998636, -81.46779532827999049, -1.194008811194000153 ) ) ;
#33710=AXIS2_PLACEMENT_3D ( 'NONE', #31689, #45003, #4560 ) ;
#33730=CARTESIAN_POINT ( 'NONE',  ( 1.546414444450387116, -82.60036552312749336, 0.02810878433797979817 ) ) ;
#33731=CARTESIAN_POINT ( 'NONE',  ( -0.7497356048005754392, -79.67399901261697437, -1.001289280827892370 ) ) ;
#33733=CARTESIAN_POINT ( 'NONE',  ( -1.250000000000000000, -81.09999999999999432, 0.000000000000000000 ) ) ;
#33760=CARTESIAN_POINT ( 'NONE',  ( -0.9181250412607999678, -79.84966061487999411, -1.434176897702999831 ) ) ;
#33761=CARTESIAN_POINT ( 'NONE',  ( -0.6295237254636235624, -81.08333333333332860, -1.092232985442822990 ) ) ;
#33777=CARTESIAN_POINT ( 'NONE',  ( 1.235246655398537730, -78.36231938546748665, 0.1914569952463864855 ) ) ;
#33784=CARTESIAN_POINT ( 'NONE',  ( 0.000000000000000000, -76.75499999999999545, 0.000000000000000000 ) ) ;
#33790=CARTESIAN_POINT ( 'NONE',  ( 0.08523424779968000187, -79.45900909512999988, -1.572136285807000045 ) ) ;
#33802=ORIENTED_EDGE ( 'NONE', *, *, #30941, .T. ) ;
#33813=ORIENTED_EDGE ( 'NONE', *, *, #58046, .F. ) ;
#33817=CARTESIAN_POINT ( 'NONE',  ( 0.02654131748702290294, -78.62385949634384019, 1.533359335126560863 ) ) ;
#33826=ADVANCED_FACE ( 'NONE', ( #39845 ), #17415, .F. ) ;
#33837=CARTESIAN_POINT ( 'NONE',  ( 0.2140083157829042182, -82.96156039968620632, 1.231433140267152115 ) ) ;
#33861=DIRECTION ( 'NONE',  ( -1.000000000000000000, 0.000000000000000000, 0.000000000000000000 ) ) ;
#33875=CARTESIAN_POINT ( 'NONE',  ( -0.8843139287876815580, -80.53818017118156547, 0.8829188658367019826 ) ) ;
#33899=SHAPE_REPRESENTATION ( 'Push Button', ( #43526 ), #52000 ) ;
#33904=CARTESIAN_POINT ( 'NONE',  ( 0.9943715457052075823, -80.93213777880458792, -1.136342727594208402 ) ) ;
#33919=DIRECTION ( 'NONE',  ( 1.000000000000000000, 0.000000000000000000, 0.000000000000000000 ) ) ;
#33923=CARTESIAN_POINT ( 'NONE',  ( -0.5050702100269550687, -79.19199393167497192, -1.144170159917196727 ) ) ;
#33924=CARTESIAN_POINT ( 'NONE',  ( 3.000000000000000000, -86.20000000000000284, 0.000000000000000000 ) ) ;
#33935=CARTESIAN_POINT ( 'NONE',  ( 1.172672253443726609, -81.37839855359489150, 0.4351029964937788708 ) ) ;
#33967=CARTESIAN_POINT ( 'NONE',  ( 0.7681833999686451531, -83.17708333333330017, -0.9995835529977240563 ) ) ;
#33972=CARTESIAN_POINT ( 'NONE',  ( -1.491326706514000122, -77.86238728987000002, -0.6515838025032999470 ) ) ;
#33980=CARTESIAN_POINT ( 'NONE',  ( -1.354012292646000093, -83.36889217614600511, -0.7194680089321999761 ) ) ;
#33981=CARTESIAN_POINT ( 'NONE',  ( 0.7712594847575999779, -80.66762112988999434, 1.518214662813999860 ) ) ;
#33995=DIRECTION ( 'NONE',  ( 1.000000000000000000, 0.000000000000000000, 0.000000000000000000 ) ) ;
#34009=CARTESIAN_POINT ( 'NONE',  ( -1.163537450530989892, -80.07049513950991582, 0.4564699256384350257 ) ) ;
#34011=ADVANCED_FACE ( 'NONE', ( #39287 ), #53188, .F. ) ;
#34016=CARTESIAN_POINT ( 'NONE',  ( -1.455028237381281730, -81.87158815977416282, -0.4162487262828510892 ) ) ;
#34026=ORIENTED_EDGE ( 'NONE', *, *, #34300, .F. ) ;
#34045=CARTESIAN_POINT ( 'NONE',  ( 0.7181780477660000273, -80.54425450742999715, 1.413724517075999998 ) ) ;
#34057=DIRECTION ( 'NONE',  ( 0.000000000000000000, 1.000000000000000000, 0.000000000000000000 ) ) ;
#34063=CARTESIAN_POINT ( 'NONE',  ( 0.8798274126591324462, -78.41291895153544544, 0.8879370300962265983 ) ) ;
#34064=( GEOMETRIC_REPRESENTATION_CONTEXT ( 3 ) GLOBAL_UNCERTAINTY_ASSIGNED_CONTEXT ( ( #28965 ) ) GLOBAL_UNIT_ASSIGNED_CONTEXT ( ( #28722, #15454, #38168 ) ) REPRESENTATION_CONTEXT ( 'NONE', 'WORKASPACE' ) );
#34070=EDGE_CURVE ( 'NONE', #23434, #38752, #950, .T. ) ;
#34077=CARTESIAN_POINT ( 'NONE',  ( 0.000000000000000000, -87.15000000002500258, -10.09999999997999964 ) ) ;
#34087=CARTESIAN_POINT ( 'NONE',  ( -0.1636246173744726473, -81.88541666666664298, 1.249999999999999112 ) ) ;
#34100=CARTESIAN_POINT ( 'NONE',  ( 0.08254163500371779205, -79.47024897342303973, 1.249696854227522635 ) ) ;
#34101=CARTESIAN_POINT ( 'NONE',  ( -1.433418477799210056, -78.77510440916314849, -0.4689554305704703996 ) ) ;
#34108=CARTESIAN_POINT ( 'NONE',  ( -0.3725602292220764333, -81.24407571201139433, 1.466352916892600167 ) ) ;
#34130=CIRCLE ( 'NONE', #15404, 10.05000000000000071 ) ;
#34147=FACE_OUTER_BOUND ( 'NONE', #2611, .T. ) ;
#34154=CARTESIAN_POINT ( 'NONE',  ( 0.000000000000000000, -76.75499999999999545, 0.000000000000000000 ) ) ;
#34161=CARTESIAN_POINT ( 'NONE',  ( -0.4115157024871364810, -80.50168328157944586, 1.181061143696242599 ) ) ;
#34188=CARTESIAN_POINT ( 'NONE',  ( 0.9648153198142549458, -79.93009253907807476, -1.161834974252261121 ) ) ;
#34192=DIRECTION ( 'NONE',  ( 0.000000000000000000, -1.000000000000000000, 0.000000000000000000 ) ) ;
#34198=CARTESIAN_POINT ( 'NONE',  ( -1.285835855790000037, -81.60322848715999555, 0.7092774996876000104 ) ) ;
#34218=CARTESIAN_POINT ( 'NONE',  ( -0.05495261879129516996, -81.47894154460885829, 1.248718060273657837 ) ) ;
#34219=CARTESIAN_POINT ( 'NONE',  ( -1.630114970985000022, -79.84613452854999593, -0.3434887894992000312 ) ) ;
#34233=CARTESIAN_POINT ( 'NONE',  ( -0.6293846543609998845, -78.55484433024999191, 1.274475086505999943 ) ) ;
#34235=ADVANCED_FACE ( 'NONE', ( #1852 ), #19376, .F. ) ;
#34258=CARTESIAN_POINT ( 'NONE',  ( -0.9156221410628999635, -78.25215827833000048, 1.345473579290000110 ) ) ;
#34263=DIRECTION ( 'NONE',  ( 0.000000000000000000, -1.000000000000000000, 0.000000000000000000 ) ) ;
#34269=CARTESIAN_POINT ( 'NONE',  ( -0.5581707956298000983, -81.36268744342000048, 1.358247929972999701 ) ) ;
#34272=LINE ( 'NONE', #16575, #38175 ) ;
#34281=VERTEX_POINT ( 'NONE', #13581 ) ;
#34300=EDGE_CURVE ( 'NONE', #22489, #19275, #37507, .T. ) ;
#34306=CARTESIAN_POINT ( 'NONE',  ( -1.442836895039729894, -82.87365703438442210, -0.4541944958676946142 ) ) ;
#34307=CARTESIAN_POINT ( 'NONE',  ( -0.8673235339713729619, -79.66431752189797066, -0.8999146696370381449 ) ) ;
#34322=AXIS2_PLACEMENT_3D ( 'NONE', #6525, #21255, #11550 ) ;
#34352=CARTESIAN_POINT ( 'NONE',  ( 0.9185483849010980251, -78.40937492225079097, 0.8489402260638932995 ) ) ;
#34358=CARTESIAN_POINT ( 'NONE',  ( 0.000000000000000000, -91.89999999999999147, 0.000000000000000000 ) ) ;
#34367=CARTESIAN_POINT ( 'NONE',  ( 0.9318330740823052016, -81.90881483467170199, 0.8363232822795773069 ) ) ;
#34368=CARTESIAN_POINT ( 'NONE',  ( 1.371113636630000077, -79.03211706016000448, -0.9421181051954000685 ) ) ;
#34391=CARTESIAN_POINT ( 'NONE',  ( -1.249311940503775809, -82.61097515347459819, -0.1638495906064939833 ) ) ;
#34396=CARTESIAN_POINT ( 'NONE',  ( -1.405018988616864251, -79.22043665247308297, 0.5474336264918724382 ) ) ;
#34403=EDGE_CURVE ( 'NONE', #35472, #12675, #16788, .T. ) ;
#34416=CARTESIAN_POINT ( 'NONE',  ( 0.3271848554490964789, -80.35416666666665719, 1.217465845835395521 ) ) ;
#34448=B_SPLINE_CURVE_WITH_KNOTS ( 'NONE', 3,
 ( #12128, #7695, #11563, #24549, #25696, #56720, #1843, #20701, #33395, #51433 ),
 .UNSPECIFIED., .F., .F.,
 ( 4, 2, 2, 2, 4 ),
 ( 0.000000000000000000, 0.2500000000000000000, 0.5000000000000000000, 0.7500000000000000000, 1.000000000000000000 ),
 .UNSPECIFIED. ) ;
#34451=CARTESIAN_POINT ( 'NONE',  ( 0.4497712132741803481, -80.44584343092967060, 1.166231044311930365 ) ) ;
#34452=EDGE_CURVE ( 'NONE', #19275, #39544, #31213, .T. ) ;
#34465=FACE_OUTER_BOUND ( 'NONE', #21524, .T. ) ;
#34479=CARTESIAN_POINT ( 'NONE',  ( 1.447876981061720691, -81.02323280059788146, 0.4369728999075917497 ) ) ;
#34482=FACE_BOUND ( 'NONE', #20327, .T. ) ;
#34489=CARTESIAN_POINT ( 'NONE',  ( -1.331776743724000234, -83.16115579321099460, -0.3115240295706999674 ) ) ;
#34492=ORIENTED_EDGE ( 'NONE', *, *, #45175, .T. ) ;
#34507=CARTESIAN_POINT ( 'NONE',  ( 1.587978134902999994, -80.66326143374000424, 0.5035716945827000135 ) ) ;
#34520=CARTESIAN_POINT ( 'NONE',  ( -0.2168337308465000113, -78.03052863245000026, 1.404775742570000041 ) ) ;
#34544=DIRECTION ( 'NONE',  ( 0.000000000000000000, -1.000000000000000000, 0.000000000000000000 ) ) ;
#34555=ORIENTED_EDGE ( 'NONE', *, *, #45187, .F. ) ;
#34556=CARTESIAN_POINT ( 'NONE',  ( -1.260823269212999920, -83.43220886491398858, -0.6699510868867000202 ) ) ;
#34557=CARTESIAN_POINT ( 'NONE',  ( -0.7850755733694999572, -79.53107020522999449, -1.063938263677999929 ) ) ;
#34561=CARTESIAN_POINT ( 'NONE',  ( 1.541440768196999933, -82.49213214217199663, 0.6318380856084999664 ) ) ;
#34565=CARTESIAN_POINT ( 'NONE',  ( 0.6812374851801442643, -81.27140723383548959, -1.049688098706359041 ) ) ;
#34574=CARTESIAN_POINT ( 'NONE',  ( -0.7572724432162000197, -83.24215694101300755, 1.483977110291999857 ) ) ;
#34580=CYLINDRICAL_SURFACE ( 'NONE', #39643, 2.500000000000000000 ) ;
#34581=CARTESIAN_POINT ( 'NONE',  ( 1.250000000000000000, -78.75000000000000000, 0.000000000000000000 ) ) ;
#34585=CARTESIAN_POINT ( 'NONE',  ( -0.9789787176784884304, -80.04688031827949146, 0.7776048570041739216 ) ) ;
#34594=CARTESIAN_POINT ( 'NONE',  ( 1.291202636478971044, -83.05585137522281514, -0.7864065562573873125 ) ) ;
#34595=CARTESIAN_POINT ( 'NONE',  ( 0.8323279321850197698, -79.78345157011268896, -0.9349414125349536642 ) ) ;
#34624=ADVANCED_FACE ( 'NONE', ( #30788 ), #39096, .T. ) ;
#34647=DIRECTION ( 'NONE',  ( 0.9999873237594404385, 0.000000000000000000, 0.005035108780572202306 ) ) ;
#34655=CARTESIAN_POINT ( 'NONE',  ( 0.4596630180541980693, -81.94513611944643117, 1.162390080072868592 ) ) ;
#34656=FACE_OUTER_BOUND ( 'NONE', #19453, .T. ) ;
#34694=ADVANCED_FACE ( 'NONE', ( #5399 ), #10131, .T. ) ;
#34704=CARTESIAN_POINT ( 'NONE',  ( 1.250000000000000000, -81.24999999999998579, 0.000000000000000000 ) ) ;
#34710=CARTESIAN_POINT ( 'NONE',  ( 1.250000000000000000, -81.84999999999999432, 0.000000000000000000 ) ) ;
#34739=CARTESIAN_POINT ( 'NONE',  ( 1.176455637918473185, -80.37807892517056985, 0.4310529391067065008 ) ) ;
#34767=CARTESIAN_POINT ( 'NONE',  ( 1.250000000000000000, -78.75000000000000000, 0.000000000000000000 ) ) ;
#34768=B_SPLINE_CURVE_WITH_KNOTS ( 'NONE', 3,
 ( #22667, #40678, #54263, #35340, #13796, #9386, #27375, #30628, #21777, #48947, #8491, #32094, #14096, #36822, #27665, #50134, #45709, #5246 ),
 .UNSPECIFIED., .F., .F.,
 ( 4, 2, 2, 2, 2, 2, 2, 2, 4 ),
 ( 0.000000000000000000, 0.1249999999999999722, 0.2500000000000000000, 0.3750000000000000000, 0.5000000000000001110, 0.6250000000000001110, 0.7500000000000000000, 0.8750000000000000000, 1.000000000000000000 ),
 .UNSPECIFIED. ) ;
#34770=CARTESIAN_POINT ( 'NONE',  ( 1.479781043334260859, -80.47666266983802075, -0.4561458805849814557 ) ) ;
#34771=DIRECTION ( 'NONE',  ( 8.423204520001998884E-11, 1.000000000000000000, -1.870146057550999887E-10 ) ) ;
#34781=CARTESIAN_POINT ( 'NONE',  ( 0.3210957952920999725, -81.22411572283999703, -1.312678830453999801 ) ) ;
#34789=CIRCLE ( 'NONE', #9364, 9.950000000000001066 ) ;
#34799=ADVANCED_FACE ( 'NONE', ( #4381 ), #22096, .T. ) ;
#34801=CARTESIAN_POINT ( 'NONE',  ( -1.529754383668999962, -81.42117201505999446, -0.6588408878327000062 ) ) ;
#34807=CARTESIAN_POINT ( 'NONE',  ( 0.3271848554490964789, -78.35416666666665719, 1.217465845835395521 ) ) ;
#34838=CARTESIAN_POINT ( 'NONE',  ( -0.9038093657317438634, -83.04000885484705918, 0.8629080614449039510 ) ) ;
#34843=CARTESIAN_POINT ( 'NONE',  ( 1.298035947816999824, -80.66793607721000114, -0.6866955795318000488 ) ) ;
#34847=CARTESIAN_POINT ( 'NONE',  ( -0.7803569495551999635, -81.79738077595999357, -1.471836271561000054 ) ) ;
#34861=CARTESIAN_POINT ( 'NONE',  ( 1.531359430757999851, -82.54740557480100449, -0.6558942768039000004 ) ) ;
#34866=CARTESIAN_POINT ( 'NONE',  ( 0.000000000000000000, -76.75499999999999545, 0.000000000000000000 ) ) ;
#34875=CARTESIAN_POINT ( 'NONE',  ( 0.3270994294228949939, -78.95440165101413754, 1.217085255381527009 ) ) ;
#34877=CARTESIAN_POINT ( 'NONE',  ( -0.3126037839058401491, -82.45865881358655258, -1.517344252390254722 ) ) ;
#34903=ADVANCED_BREP_SHAPE_REPRESENTATION ( '', ( #36811, #43526 ), #52000 ) ;
#34940=CARTESIAN_POINT ( 'NONE',  ( 0.4751859727251985799, -81.94403392660923657, 1.156120668747460334 ) ) ;
#34947=CARTESIAN_POINT ( 'NONE',  ( -1.135826688880000157, -81.40663953506998496, -0.9797437077257000748 ) ) ;
#34977=CARTESIAN_POINT ( 'NONE',  ( -1.300896064473999969, -80.10182505433999722, -0.3655689422679000433 ) ) ;
#35020=MECHANICAL_DESIGN_GEOMETRIC_PRESENTATION_REPRESENTATION('',(#48261),#34064);
#35021=B_SPLINE_CURVE_WITH_KNOTS ( 'NONE', 3,
 ( #46382, #5906, #33352, #33923, #51099, #37200, #28922, #10650, #33641, #46679, #35866, #27002, #50849, #10395, #45037, #4590, #55259, #9306, #19252, #23958, #18172, #37535, #6244, #24261, #42277, #16854, #43728, #24842, #24551, #21272, #25416, #25699, #57290, #56723, #3280 ),
 .UNSPECIFIED., .F., .F.,
 ( 4, 2, 2, 2, 1, 1, 2, 2, 2, 2, 1, 1, 2, 2, 2, 2, 1, 2, 2, 4 ),
 ( 0.000000000000000000, 0.1250000000000194011, 0.1875000000000297817, 0.2187500000000348055, 0.2343750000000359990, 0.2421875000000349443, 0.2460937500000344447, 0.2500000000000339173, 0.3750000000000124900, 0.4375000000000017764, 0.4687499999999963918, 0.4843749999999936162, 0.4921874999999931721, 0.4999999999999927280, 0.6249999999999864553, 0.6874999999999840128, 0.7187499999999836797, 0.7343749999999844569, 0.7499999999999851230, 1.000000000000000000 ),
 .UNSPECIFIED. ) ;
#35036=CARTESIAN_POINT ( 'NONE',  ( -1.436413824931296546, -77.87453550735162366, -0.4659587443401291829 ) ) ;
#35040=ADVANCED_FACE ( 'NONE', ( #23196, #58037 ), #41201, .T. ) ;
#35048=CARTESIAN_POINT ( 'NONE',  ( -0.9492059026655267351, -80.77846795208610331, 1.175833850632304278 ) ) ;
#35053=B_SPLINE_CURVE_WITH_KNOTS ( 'NONE', 3,
 ( #28614, #50201, #46659, #31873, #9462, #45483, #23030, #41045, #634, #18616, #9751, #45784, #41334, #29758, #16499, #42793, #56083, #7346 ),
 .UNSPECIFIED., .F., .F.,
 ( 4, 2, 2, 2, 2, 2, 2, 2, 4 ),
 ( 0.000000000000000000, 0.1249999999999999722, 0.2500000000000000000, 0.3750000000000000000, 0.5000000000000001110, 0.6250000000000001110, 0.7500000000000000000, 0.8750000000000000000, 1.000000000000000000 ),
 .UNSPECIFIED. ) ;
#35058=CARTESIAN_POINT ( 'NONE',  ( -1.211920851286000023, -81.18216705308998371, -0.6339750518301998650 ) ) ;
#35077=CARTESIAN_POINT ( 'NONE',  ( 1.356773869401999955, -79.58955477686998847, -0.9668579442890000708 ) ) ;
#35127=CARTESIAN_POINT ( 'NONE',  ( 0.6444261930239000291, -82.67414080993400205, 1.576239777183000124 ) ) ;
#35128=CARTESIAN_POINT ( 'NONE',  ( -1.251342548660999920, -81.48916334729999278, 0.5102646838515999539 ) ) ;
#35133=CARTESIAN_POINT ( 'NONE',  ( -0.6811744818814000624, -82.30265449683999179, -1.520282978132999840 ) ) ;
#35148=CARTESIAN_POINT ( 'NONE',  ( -0.2201363562291999698, -79.46327907014000402, -1.483758735329000045 ) ) ;
#35152=CARTESIAN_POINT ( 'NONE',  ( 1.050086718088998339, -79.89624094074886784, 0.6784569047000227338 ) ) ;
#35204=CARTESIAN_POINT ( 'NONE',  ( 1.250000000000000000, -83.24999999999998579, 0.000000000000000000 ) ) ;
#35208=AXIS2_PLACEMENT_3D ( 'NONE', #57896, #26885, #17453 ) ;
#35216=CLOSED_SHELL ( 'NONE', ( #39444, #5306, #34799, #9788, #45973, #44762, #51066, #1016, #57746, #31934, #35674, #20356, #32476, #26147, #37896, #29070, #57109, #34235, #34011, #35669, #57866, #51435, #35279, #8052, #3316, #37159, #20923, #17983, #49839, #6435, #47898, #52208, #45048, #16202, #33826, #2342, #49581, #1651, #14943, #47789, #16587, #29304, #32347, #15289, #38475, #20748, #1791, #42642, #22976, #52482, #37564, #34624, #34694, #39216, #39646, #50757, #44829, #13761, #51985, #35040, #40090, #27501, #10228, #19593 ) ) ;
#35224=CARTESIAN_POINT ( 'NONE',  ( 0.1696949479679999984, -78.19689351345999739, 1.654914741598999983 ) ) ;
#35226=CARTESIAN_POINT ( 'NONE',  ( -1.441818230322603700, -82.77428155285538480, -0.4538374300033769515 ) ) ;
#35234=CARTESIAN_POINT ( 'NONE',  ( -1.092316917947570243, -78.14177812212517438, -0.6297690996598702684 ) ) ;
#35265=CARTESIAN_POINT ( 'NONE',  ( -0.4297501350614000293, -80.48078034499999944, 1.281126864269000132 ) ) ;
#35276=EDGE_LOOP ( 'NONE', ( #54859, #22335, #28588, #3691 ) ) ;
#35279=ADVANCED_FACE ( 'NONE', ( #24655 ), #9916, .F. ) ;
#35288=DIRECTION ( 'NONE',  ( 1.000000000000000000, 0.000000000000000000, 0.000000000000000000 ) ) ;
#35334=CARTESIAN_POINT ( 'NONE',  ( -1.250000000000000000, -83.49999999999998579, 0.000000000000000000 ) ) ;
#35340=CARTESIAN_POINT ( 'NONE',  ( -1.092232985442824100, -80.95833333333330017, 0.6295237254636200097 ) ) ;
#35342=CARTESIAN_POINT ( 'NONE',  ( -0.1550674183001617967, -80.23188492957339690, 1.542021311756852864 ) ) ;
#35351=CARTESIAN_POINT ( 'NONE',  ( 0.7304821784857000733, -81.47691005693999955, 1.273910602969000161 ) ) ;
#35367=CARTESIAN_POINT ( 'NONE',  ( 0.000000000000000000, -76.75499999999999545, 0.000000000000000000 ) ) ;
#35380=VERTEX_POINT ( 'NONE', #29357 ) ;
#35386=CARTESIAN_POINT ( 'NONE',  ( 0.9442298177897724409, -80.29360019353696032, -0.8189497213649101770 ) ) ;
#35415=CARTESIAN_POINT ( 'NONE',  ( 1.385204701026000018, -83.17972947813200335, -0.4875042294149000144 ) ) ;
#35416=CARTESIAN_POINT ( 'NONE',  ( -0.7646200840319000713, -80.47830095821998952, -1.389155443296000048 ) ) ;
#35420=FACE_OUTER_BOUND ( 'NONE', #15005, .T. ) ;
#35433=CARTESIAN_POINT ( 'NONE',  ( -0.8762103189736000219, -81.35132337894999921, -1.416501064863000092 ) ) ;
#35442=CARTESIAN_POINT ( 'NONE',  ( 1.154033295362816514, -79.88162843165144977, 0.4798940756958068876 ) ) ;
#35448=CARTESIAN_POINT ( 'NONE',  ( -1.339212577895066758, -81.81085671282828287, 0.7051202410463707215 ) ) ;
#35470=CARTESIAN_POINT ( 'NONE',  ( 0.8568216711331626545, -79.41513557398620549, 0.9100032604084061783 ) ) ;
#35472=VERTEX_POINT ( 'NONE', #15796 ) ;
#35516=FACE_OUTER_BOUND ( 'NONE', #1598, .T. ) ;
#35517=B_SPLINE_CURVE_WITH_KNOTS ( 'NONE', 3,
 ( #43575, #3138, #56287, #2558, #20559, #19985, #15543, #25269, #38557, #56572, #16131, #34108, #29112, #6688, #42707, #2274, #20271, #49546, #4366, #49842, #40074, #58091, #27079, #53667, #22669, #40681, #9091, #45120, #17950, #57796, #31499, #36244, #21495, #17353, #17651, #45414, #22368, #40380, #13507, #58388, #31202, #35048, #35942, #22066, #273, #26488, #39782, #4670, #18252, #30913, #3774, #31800, #35639, #54265, #13207, #13798, #9389, #27377, #39501, #53969, #35342, #44512, #8492, #57505, #17067, #53365, #53082, #48949, #4062, #12916, #12637, #49241, #30629, #48662, #8792, #26784, #44813, #8207, #26209, #44226, #21778, #9679, #565, #6119, #23537, #28544, #55127, #51011, #19121, #848, #41263, #36534, #14672, #32097, #27667, #41550, #46004, #5528, #45713, #37112, #9976, #32669, #14970, #40973, #5249, #1133, #10561, #50136 ),
 .UNSPECIFIED., .F., .F.,
 ( 4, 2, 2, 2, 2, 2, 1, 2, 2, 2, 2, 2, 2, 2, 2, 2, 2, 2, 2, 2, 2, 2, 2, 2, 2, 2, 2, 2, 2, 2, 2, 2, 2, 2, 2, 2, 2, 2, 2, 2, 2, 2, 2, 2, 2, 2, 2, 2, 1, 2, 2, 2, 2, 2, 4 ),
 ( 0.000000000000000000, 0.01562500000000001041, 0.03125000000000001388, 0.04687500000000002082, 0.06250000000000002776, 0.07812500000000004163, 0.09375000000000004163, 0.1093750000000000416, 0.1250000000000000278, 0.1406250000000000278, 0.1562500000000000555, 0.1718750000000000555, 0.1875000000000000555, 0.2031250000000000833, 0.2187500000000000833, 0.2343750000000001110, 0.2500000000000001110, 0.2656250000000001110, 0.2812500000000001110, 0.2968750000000001665, 0.3125000000000001665, 0.3281250000000001665, 0.3437500000000001665, 0.3750000000000001110, 0.4062500000000001110, 0.4375000000000000555, 0.4687500000000000555, 0.5000000000000000000, 0.5312499999999998890, 0.5624999999999997780, 0.5937499999999998890, 0.6249999999999998890, 0.6562499999999998890, 0.6718749999999998890, 0.6874999999999998890, 0.7031249999999998890, 0.7187499999999998890, 0.7343749999999998890, 0.7499999999999998890, 0.7656250000000000000, 0.7812500000000000000, 0.7968750000000000000, 0.8125000000000000000, 0.8281250000000000000, 0.8437500000000000000, 0.8593750000000000000, 0.8750000000000000000, 0.8906250000000000000, 0.9062500000000000000, 0.9218750000000001110, 0.9375000000000001110, 0.9531250000000001110, 0.9687500000000001110, 0.9843750000000001110, 1.000000000000000000 ),
 .UNSPECIFIED. ) ;
#35521=CARTESIAN_POINT ( 'NONE',  ( 0.8752045112715043373, -81.91385899954191530, 0.8919628724664445674 ) ) ;
#35522=CARTESIAN_POINT ( 'NONE',  ( -0.6667013398134999935, -78.48293648134999501, -1.398288081058000065 ) ) ;
#35524=CARTESIAN_POINT ( 'NONE',  ( 1.051432699053240105, -82.93622825826652445, -1.083844963264632977 ) ) ;
#35531=CARTESIAN_POINT ( 'NONE',  ( 0.9143116702203477608, -81.79083299997489576, -0.8519700409851096445 ) ) ;
#35534=CARTESIAN_POINT ( 'NONE',  ( 0.7681833999686451531, -80.17708333333334281, -0.9995835529977240563 ) ) ;
#35537=CARTESIAN_POINT ( 'NONE',  ( 0.000000000000000000, -77.70312499986998489, 0.000000000000000000 ) ) ;
#35554=ORIENTED_EDGE ( 'NONE', *, *, #31409, .F. ) ;
#35556=CARTESIAN_POINT ( 'NONE',  ( -1.473982314889778600, -77.76680499034375771, -0.3169618534076995564 ) ) ;
#35587=VECTOR ( 'NONE', #19588, 1000.000000000000000 ) ;
#35598=VECTOR ( 'NONE', #57248, 1000.000000000000000 ) ;
#35639=CARTESIAN_POINT ( 'NONE',  ( 0.01771975371708433070, -80.47481071735674618, -1.547929127693172147 ) ) ;
#35640=CARTESIAN_POINT ( 'NONE',  ( -0.6573153308273406159, -78.51914022995057962, 1.070387359618083956 ) ) ;
#35650=CARTESIAN_POINT ( 'NONE',  ( 0.7887820451556000201, -81.54022674571000096, 1.375581554690999964 ) ) ;
#35669=ADVANCED_FACE ( 'NONE', ( #7656 ), #22090, .F. ) ;
#35670=CARTESIAN_POINT ( 'NONE',  ( 1.250000000000000000, -81.74999999999998579, 0.000000000000000000 ) ) ;
#35671=CARTESIAN_POINT ( 'NONE',  ( 1.640574411872000038, -79.65271399197999358, 0.2893137654249999802 ) ) ;
#35674=ADVANCED_FACE ( 'NONE', ( #48976 ), #41076, .F. ) ;
#35690=CARTESIAN_POINT ( 'NONE',  ( 1.466105194966000003, -78.93275043768998955, -0.4542193573542999685 ) ) ;
#35694=CARTESIAN_POINT ( 'NONE',  ( 0.8841121778318057345, -80.28811247499398007, -0.8831609924660611677 ) ) ;
#35695=CARTESIAN_POINT ( 'NONE',  ( 0.1861230080285300181, -77.83463541685786424, -1.415364582351019918 ) ) ;
#35708=AXIS2_PLACEMENT_3D ( 'NONE', #27439, #5307, #5017 ) ;
#35719=CARTESIAN_POINT ( 'NONE',  ( 0.5557217581696000108, -82.80077418747099216, 1.359272403504999893 ) ) ;
#35720=CARTESIAN_POINT ( 'NONE',  ( 1.312293141192999890, -80.28913826020999522, 0.3222699683723999620 ) ) ;
#35735=CARTESIAN_POINT ( 'NONE',  ( 1.611423453808999984, -81.54080102427998611, 0.4225784326546000447 ) ) ;
#35750=CARTESIAN_POINT ( 'NONE',  ( 0.2396844382371944027, -81.48695566245035593, -1.494320044138283565 ) ) ;
#35759=ORIENTED_EDGE ( 'NONE', *, *, #20823, .F. ) ;
#35770=CARTESIAN_POINT ( 'NONE',  ( -0.9465222407332000154, -81.15663953506998496, -0.8164530897714000757 ) ) ;
#35773=CARTESIAN_POINT ( 'NONE',  ( 1.147151915388343157, -79.38294062387207362, 0.4959029880282930791 ) ) ;
#35781=CARTESIAN_POINT ( 'NONE',  ( -0.9536002873971000104, -79.13599388661999967, 1.318830682536000110 ) ) ;
#35822=CARTESIAN_POINT ( 'NONE',  ( -0.9131908197385000259, -81.34484551072999636, -1.254418330386999791 ) ) ;
#35823=CARTESIAN_POINT ( 'NONE',  ( -0.8405898119991999096, -79.38147671680999906, 1.162537019067000132 ) ) ;
#35825=CARTESIAN_POINT ( 'NONE',  ( -0.5174486800468990344, -82.65282152379752745, 1.420763823235222212 ) ) ;
#35830=CARTESIAN_POINT ( 'NONE',  ( 1.045316320065775351, -81.80395334762980042, -0.6852794371750267066 ) ) ;
#35831=DIRECTION ( 'NONE',  ( 0.000000000000000000, 1.000000000000000000, 0.000000000000000000 ) ) ;
#35834=EDGE_LOOP ( 'NONE', ( #31990, #4789, #22926, #37224, #55620 ) ) ;
#35864=CARTESIAN_POINT ( 'NONE',  ( 1.233662806718999860, -80.79657642056000100, -0.5514036435800000469 ) ) ;
#35866=CARTESIAN_POINT ( 'NONE',  ( -0.6000517156062694646, -79.18523342396193243, -1.096500065134945912 ) ) ;
#35867=DIRECTION ( 'NONE',  ( 1.000000000000000000, 0.000000000000000000, 0.000000000000000000 ) ) ;
#35903=CARTESIAN_POINT ( 'NONE',  ( -0.7623087083147439547, -77.75000000000001421, 1.329504222413994574 ) ) ;
#35904=FACE_OUTER_BOUND ( 'NONE', #38014, .T. ) ;
#35911=CARTESIAN_POINT ( 'NONE',  ( -1.500000000000000000, -83.24999999999998579, 0.000000000000000000 ) ) ;
#35912=DIRECTION ( 'NONE',  ( 0.000000000000000000, 1.000000000000000000, 0.000000000000000000 ) ) ;
#35942=CARTESIAN_POINT ( 'NONE',  ( -0.6250699663053016497, -80.75822413643739139, 1.377587401609168705 ) ) ;
#35952=CARTESIAN_POINT ( 'NONE',  ( -1.491081270832000039, -81.72986186469999836, 0.8224925373206000145 ) ) ;
#35955=DIRECTION ( 'NONE',  ( 0.000000000000000000, 0.000000000000000000, -1.000000000000000000 ) ) ;
#35971=CARTESIAN_POINT ( 'NONE',  ( 0.000000000000000000, -77.50000000000000000, -1.749999999999931166 ) ) ;
#35988=CARTESIAN_POINT ( 'NONE',  ( -1.437605742302000111, -79.31065654513999164, -0.8064262874623000510 ) ) ;
#36016=CARTESIAN_POINT ( 'NONE',  ( -0.4887637738901999818, -82.35865968170000428, 1.384759226041999858 ) ) ;
#36017=CARTESIAN_POINT ( 'NONE',  ( 1.233662806718999860, -81.23652648686000077, -0.5514036435800000469 ) ) ;
#36021=CARTESIAN_POINT ( 'NONE',  ( 1.579899301681999990, -82.04607474515999854, 0.5283722218587000308 ) ) ;
#36043=CONICAL_SURFACE ( 'NONE', #27564, 10.09999999997999964, 0.7853981633972997312 ) ;
#36047=CARTESIAN_POINT ( 'NONE',  ( -0.9232088357456459393, -81.54158477673213667, 0.8426130859076562674 ) ) ;
#36083=CARTESIAN_POINT ( 'NONE',  ( 1.153380192234999990, -78.58271294291999709, 1.148206073167999941 ) ) ;
#36091=VERTEX_POINT ( 'NONE', #50936 ) ;
#36123=CARTESIAN_POINT ( 'NONE',  ( 0.7545134501129999727, -80.54877167723999776, 1.485250302772000097 ) ) ;
#36124=CARTESIAN_POINT ( 'NONE',  ( -0.5989072293159000138, -79.04738729812999054, -1.303606512140000007 ) ) ;
#36126=CARTESIAN_POINT ( 'NONE',  ( -0.2578204775944251126, -83.13866164002989478, 1.488022452193133116 ) ) ;
#36133=CARTESIAN_POINT ( 'NONE',  ( 1.161390734570817651, -81.81998499750356757, -0.4620521855202992523 ) ) ;
#36140=ORIENTED_EDGE ( 'NONE', *, *, #29545, .F. ) ;
#36145=CARTESIAN_POINT ( 'NONE',  ( 1.154746208549590092, -80.38136168085064526, 0.4784273033405310183 ) ) ;
#36189=ORIENTED_EDGE ( 'NONE', *, *, #46191, .T. ) ;
#36197=CARTESIAN_POINT ( 'NONE',  ( -1.250000000000001332, -82.48958333333335702, 0.1636246173744632659 ) ) ;
#36202=ORIENTED_EDGE ( 'NONE', *, *, #23435, .T. ) ;
#36244=CARTESIAN_POINT ( 'NONE',  ( -0.7958789691180911952, -80.93029656945788020, -1.286331066359134745 ) ) ;
#36254=CARTESIAN_POINT ( 'NONE',  ( 1.362316189135000188, -81.41390831549000495, -0.8114345006153000917 ) ) ;
#36273=AXIS2_PLACEMENT_3D ( 'NONE', #8363, #21935, #39946 ) ;
#36283=CIRCLE ( 'NONE', #20246, 2.500000000000000000 ) ;
#36288=CARTESIAN_POINT ( 'NONE',  ( 1.354794440577000048, -78.47175142865999931, -0.9388388050506000226 ) ) ;
#36291=CARTESIAN_POINT ( 'NONE',  ( 0.5018392586016090506, -80.25806588323808910, -1.144748121017402198 ) ) ;
#36312=CARTESIAN_POINT ( 'NONE',  ( 1.358765745638999878, -82.73761497235999229, 0.5569594143531000352 ) ) ;
#36316=CARTESIAN_POINT ( 'NONE',  ( -1.092232985442824100, -78.95833333333330017, 0.6295237254636200097 ) ) ;
#36342=CARTESIAN_POINT ( 'NONE',  ( 1.395804191767038516, -81.56793092504486253, -0.5836528581437869789 ) ) ;
#36373=CARTESIAN_POINT ( 'NONE',  ( 0.1742577344548000007, -77.63612625665999190, 1.489843697164999980 ) ) ;
#36411=CARTESIAN_POINT ( 'NONE',  ( 1.640574411872000038, -79.47506502036999620, 0.2893137654249999802 ) ) ;
#36412=CARTESIAN_POINT ( 'NONE',  ( 0.3991026885628000120, -79.54088630715999386, -1.370848940981999942 ) ) ;
#36420=CARTESIAN_POINT ( 'NONE',  ( 0.8175227547224469538, -81.78223890415932829, -0.9484037626542538568 ) ) ;
#36448=CARTESIAN_POINT ( 'NONE',  ( -0.6213570041975999825, -80.73357467910000196, -1.330550119908999962 ) ) ;
#36487=FACE_OUTER_BOUND ( 'NONE', #43054, .T. ) ;
#36491=CARTESIAN_POINT ( 'NONE',  ( -1.398183675150702632, -77.75000000000000000, 0.6275176927634855684 ) ) ;
#36506=CARTESIAN_POINT ( 'NONE',  ( 1.018183232918382863, -82.80095525923850630, -0.7285541732893786593 ) ) ;
#36514=DIRECTION ( 'NONE',  ( 0.000000000000000000, 1.000000000000000000, 0.000000000000000000 ) ) ;
#36534=CARTESIAN_POINT ( 'NONE',  ( 0.1656092252224484473, -79.71566763053364468, 1.502111356206679460 ) ) ;
#36535=CARTESIAN_POINT ( 'NONE',  ( -0.01915452949074002847, -78.47644932240093851, 1.249713897098126747 ) ) ;
#36539=CARTESIAN_POINT ( 'NONE',  ( 0.3271848554491016414, -80.64583333333330017, -1.217465845835393967 ) ) ;
#36546=CARTESIAN_POINT ( 'NONE',  ( 0.6959559787155999988, -82.04550046658999918, 1.424795421937999906 ) ) ;
#36547=VERTEX_POINT ( 'NONE', #27672 ) ;
#36559=EDGE_LOOP ( 'NONE', ( #49951, #5222, #25465 ) ) ;
#36577=CARTESIAN_POINT ( 'NONE',  ( 0.9462631019772999030, -78.94363555667999321, -1.349619363059000099 ) ) ;
#36582=CARTESIAN_POINT ( 'NONE',  ( -0.8830740761637451142, -80.16309161040983611, -0.8842243533770794972 ) ) ;
#36603=CARTESIAN_POINT ( 'NONE',  ( -1.436129866501999919, -82.35850220804000799, 0.6722556991877999266 ) ) ;
#36604=CARTESIAN_POINT ( 'NONE',  ( 1.149971879181999945, -80.22597904509999012, -0.7096026395132000175 ) ) ;
#36609=CARTESIAN_POINT ( 'NONE',  ( 1.571434226476000173, -82.99346297181298837, -0.5530452149683998675 ) ) ;
#36630=LINE ( 'NONE', #1225, #32364 ) ;
#36633=CARTESIAN_POINT ( 'NONE',  ( -1.247161917481749205, -81.59353255999356236, 0.1116756905574352032 ) ) ;
#36656=ORIENTED_EDGE ( 'NONE', *, *, #7817, .T. ) ;
#36666=CARTESIAN_POINT ( 'NONE',  ( 0.1742577344548000007, -77.57690993279000224, 1.489843697164999980 ) ) ;
#36703=CARTESIAN_POINT ( 'NONE',  ( 1.472546342128999930, -80.48166957088999141, -0.7790162248558000213 ) ) ;
#36704=CARTESIAN_POINT ( 'NONE',  ( -1.202031245603000009, -78.55388828911000587, -0.5457094238513999773 ) ) ;
#36706=CARTESIAN_POINT ( 'NONE',  ( 1.519135534786491659, -82.01515637124201419, 0.3015387213458061155 ) ) ;
#36710=CARTESIAN_POINT ( 'NONE',  ( 1.169986272277216299, -79.82176322311053696, -0.4396409049908809319 ) ) ;
#36713=CARTESIAN_POINT ( 'NONE',  ( 0.5491531115358451176, -81.76143395608764308, -1.122793678249770055 ) ) ;
#36716=CARTESIAN_POINT ( 'NONE',  ( 0.6295237254636258939, -80.16666666666664298, -1.092232985442821658 ) ) ;
#36730=ORIENTED_EDGE ( 'NONE', *, *, #20861, .T. ) ;
#36738=CARTESIAN_POINT ( 'NONE',  ( -0.7917463127232999831, -79.72302723733999130, -1.236764296276999797 ) ) ;
#36772=CARTESIAN_POINT ( 'NONE',  ( 1.249999999999999778, -82.26041666666665719, 0.1636246173744711763 ) ) ;
#36775=CARTESIAN_POINT ( 'NONE',  ( -1.250000000000000000, -82.09999999999999432, 0.000000000000000000 ) ) ;
#36811=MANIFOLD_SOLID_BREP ( 'Stock-MAS-694-1', #35216 ) ;
#36822=CARTESIAN_POINT ( 'NONE',  ( 0.9995835529977233902, -80.80208333333332860, 0.7681833999686461523 ) ) ;
#36833=CARTESIAN_POINT ( 'NONE',  ( 0.6444261930239000291, -82.61409087623900405, 1.576239777183000124 ) ) ;
#36852=CARTESIAN_POINT ( 'NONE',  ( 1.218242831762920586, -80.82990848825727426, -0.3279570865790462642 ) ) ;
#36858=VERTEX_POINT ( 'NONE', #34710 ) ;
#36860=CARTESIAN_POINT ( 'NONE',  ( -1.158645246675607199, -80.56947091650550874, 0.4690212617335481893 ) ) ;
#36870=CARTESIAN_POINT ( 'NONE',  ( -0.8777456576965628754, -80.16355898801532476, -0.8895264229757680052 ) ) ;
#36875=CARTESIAN_POINT ( 'NONE',  ( -1.531361644451373349, -78.35640210815725482, -0.1250911378582522659 ) ) ;
#36892=CARTESIAN_POINT ( 'NONE',  ( -1.172849536488999922, -80.47861590553999633, 0.6711148834816000885 ) ) ;
#36894=CARTESIAN_POINT ( 'NONE',  ( 1.250000000000000000, -82.74999999999998579, 0.000000000000000000 ) ) ;
#36896=CARTESIAN_POINT ( 'NONE',  ( 0.6062141276560999437, -82.42503003582099552, -1.551696954864999922 ) ) ;
#36955=CARTESIAN_POINT ( 'NONE',  ( 1.314530797355000225, -77.97021567534000042, -0.9595159925157999981 ) ) ;
#36992=CARTESIAN_POINT ( 'NONE',  ( -0.7426966924155999905, -78.44252514954999356, 1.091365894571999950 ) ) ;
#36994=CARTESIAN_POINT ( 'NONE',  ( 0.08823669215798200793, -81.62041127680433306, 1.507463071252419962 ) ) ;
#37000=CARTESIAN_POINT ( 'NONE',  ( -0.3656892198172155273, -81.70169265833098393, -1.195345686084333225 ) ) ;
#37024=CARTESIAN_POINT ( 'NONE',  ( 0.6295237254636211199, -81.33333333333334281, 1.092232985442824322 ) ) ;
#37030=CARTESIAN_POINT ( 'NONE',  ( 0.5538255850406000880, -80.86005058297999426, -1.485824439479999981 ) ) ;
#37061=CARTESIAN_POINT ( 'NONE',  ( 0.000000000000000000, -87.15000000002500258, 0.000000000000000000 ) ) ;
#37070=FACE_OUTER_BOUND ( 'NONE', #27345, .T. ) ;
#37104=CARTESIAN_POINT ( 'NONE',  ( -0.1834469635243000107, -79.61327907013999550, -1.236465612773999911 ) ) ;
#37105=CARTESIAN_POINT ( 'NONE',  ( 0.1782616899984783287, -82.96393278609434674, 1.237108939223909410 ) ) ;
#37112=CARTESIAN_POINT ( 'NONE',  ( 1.435088794311236482, -79.57396092099332918, -0.4737081478796364431 ) ) ;
#37113=CARTESIAN_POINT ( 'NONE',  ( -1.250000000000000000, -81.49999999999998579, 0.000000000000000000 ) ) ;
#37117=CARTESIAN_POINT ( 'NONE',  ( 0.9995835529977264988, -80.69791666666664298, -0.7681833999686417114 ) ) ;
#37145=DIRECTION ( 'NONE',  ( -1.000000000000000000, 0.000000000000000000, 0.000000000000000000 ) ) ;
#37159=ADVANCED_FACE ( 'NONE', ( #46314 ), #14983, .F. ) ;
#37164=CARTESIAN_POINT ( 'NONE',  ( -0.8423982081441719894, -80.16660507476834141, -0.9234063250311906890 ) ) ;
#37171=CARTESIAN_POINT ( 'NONE',  ( 1.508773389166936818, -79.09704892049856539, -0.04912781361764535087 ) ) ;
#37184=CARTESIAN_POINT ( 'NONE',  ( -0.7723712723579000405, -81.53758988526999474, -1.248632555533999877 ) ) ;
#37187=CARTESIAN_POINT ( 'NONE',  ( 0.7681833999686413783, -82.82291666666667140, 0.9995835529977274980 ) ) ;
#37200=CARTESIAN_POINT ( 'NONE',  ( -0.5656538306440472841, -79.18769777830807755, -1.114770703783219963 ) ) ;
#37205=VERTEX_POINT ( 'NONE', #27684 ) ;
#37212=CARTESIAN_POINT ( 'NONE',  ( -1.192707094028399473, -81.57616841835279331, 0.3740703197376714639 ) ) ;
#37215=CARTESIAN_POINT ( 'NONE',  ( -0.4521203515703999809, -78.17693822280000404, -1.227342538824000018 ) ) ;
#37219=ORIENTED_EDGE ( 'NONE', *, *, #9566, .F. ) ;
#37224=ORIENTED_EDGE ( 'NONE', *, *, #24317, .F. ) ;
#37245=CARTESIAN_POINT ( 'NONE',  ( 1.314530797355000225, -77.91099935146999655, -0.9595159925157999981 ) ) ;
#37254=CARTESIAN_POINT ( 'NONE',  ( 0.6690176526880000640, -81.17289485077999700, 1.565960205386000004 ) ) ;
#37283=CARTESIAN_POINT ( 'NONE',  ( 0.6544915521845998674, -81.23169436972999335, 1.531959166345999934 ) ) ;
#37286=CARTESIAN_POINT ( 'NONE',  ( 0.4637052088425716589, -81.60016793862807560, 1.437828183278014649 ) ) ;
#37292=CARTESIAN_POINT ( 'NONE',  ( -0.2634504916890236803, -81.70857297640610284, -1.222512182397711200 ) ) ;
#37322=CARTESIAN_POINT ( 'NONE',  ( -0.8049692409160000839, -81.21779532827999049, -1.105758127848999850 ) ) ;
#37363=FACE_OUTER_BOUND ( 'NONE', #46375, .T. ) ;
#37376=CARTESIAN_POINT ( 'NONE',  ( 1.160213112257555412, -82.81967442626978482, -0.4651854077409782739 ) ) ;
#37382=DIRECTION ( 'NONE',  ( 0.000000000000000000, 0.7071067811866525998, -0.7071067811864425456 ) ) ;
#37397=CARTESIAN_POINT ( 'NONE',  ( 0.2409842076378775344, -82.95976104365308856, 1.226430088683852615 ) ) ;
#37407=CARTESIAN_POINT ( 'NONE',  ( -1.217465845835394411, -80.52083333333330017, -0.3271848554491003647 ) ) ;
#37428=ORIENTED_EDGE ( 'NONE', *, *, #6956, .T. ) ;
#37436=CARTESIAN_POINT ( 'NONE',  ( 0.3244733924317961260, -80.74656484181741689, -1.210953765918606706 ) ) ;
#37437=ORIENTED_EDGE ( 'NONE', *, *, #34403, .F. ) ;
#37450=CARTESIAN_POINT ( 'NONE',  ( -1.595587217727999940, -77.79014102152999044, -0.4130859425818000363 ) ) ;
#37454=CARTESIAN_POINT ( 'NONE',  ( -0.4317206087502349354, -80.19718752668565287, -1.173039634006793452 ) ) ;
#37458=CARTESIAN_POINT ( 'NONE',  ( 1.375849008456478506, -78.13331571889540328, 0.6192971689456351347 ) ) ;
#37461=CYLINDRICAL_SURFACE ( 'NONE', #44588, 1.250000000000000000 ) ;
#37471=CARTESIAN_POINT ( 'NONE',  ( -1.505598529332060842, -81.25603118963000782, -0.1141384907295430601 ) ) ;
#37474=CARTESIAN_POINT ( 'NONE',  ( 0.9995835529977233902, -78.80208333333334281, 0.7681833999686461523 ) ) ;
#37480=CARTESIAN_POINT ( 'NONE',  ( -1.225487488653999923, -83.09783910444198796, -0.2866612609456000160 ) ) ;
#37499=CARTESIAN_POINT ( 'NONE',  ( 1.234146787099059228, -81.36395189309098441, 0.2159370409434396010 ) ) ;
#37507=B_SPLINE_CURVE_WITH_KNOTS ( 'NONE', 3,
 ( #13286, #14457, #49321, #40457, #4147, #41333, #4739, #23029, #22738, #45482, #5318, #54904, #18900, #22147 ),
 .UNSPECIFIED., .F., .F.,
 ( 4, 2, 2, 2, 2, 2, 4 ),
 ( 0.000000000000000000, 0.1249999999999997502, 0.2499999999999995004, 0.4999999999999996669, 0.7499999999999997780, 0.8749999999999998890, 1.000000000000000000 ),
 .UNSPECIFIED. ) ;
#37534=CARTESIAN_POINT ( 'NONE',  ( -1.566959183383000109, -78.30783984810999243, 0.4396611996733000294 ) ) ;
#37535=CARTESIAN_POINT ( 'NONE',  ( -0.9416178767894587409, -79.15734073197442910, -0.8218901853645335098 ) ) ;
#37544=CARTESIAN_POINT ( 'NONE',  ( 1.585573224116000102, -81.10973563566999189, 0.6211121348122999875 ) ) ;
#37564=ADVANCED_FACE ( 'NONE', ( #32038, #9919 ), #27615, .F. ) ;
#37575=CARTESIAN_POINT ( 'NONE',  ( 0.3704480504712000521, -79.91323663489998808, -1.624200486671999899 ) ) ;
#37576=CARTESIAN_POINT ( 'NONE',  ( -1.271021473223000076, -78.49820671932999971, 0.3566262807950000280 ) ) ;
#37585=CARTESIAN_POINT ( 'NONE',  ( 0.09314403347896584029, -81.73140747789805971, -1.246441406727125223 ) ) ;
#37589=ORIENTED_EDGE ( 'NONE', *, *, #1881, .T. ) ;
#37595=ORIENTED_EDGE ( 'NONE', *, *, #20636, .T. ) ;
#37614=CARTESIAN_POINT ( 'NONE',  ( -1.413725673013999984, -80.16514174310999863, -0.3972755495651000279 ) ) ;
#37617=CARTESIAN_POINT ( 'NONE',  ( -1.473604374833289654, -79.76814583366768829, -0.3405220590759504007 ) ) ;
#37655=CARTESIAN_POINT ( 'NONE',  ( 0.000000000000000000, -86.20000000000000284, 0.000000000000000000 ) ) ;
#37663=ORIENTED_EDGE ( 'NONE', *, *, #17692, .T. ) ;
#37670=CARTESIAN_POINT ( 'NONE',  ( 1.237861236329913295, -82.83936588051422234, -0.1724589212497519564 ) ) ;
#37674=CARTESIAN_POINT ( 'NONE',  ( -1.209088188845623968, -79.58012613440236294, 0.3181738888800063059 ) ) ;
#37675=CARTESIAN_POINT ( 'NONE',  ( 0.01373196070286510778, -78.87593435104115258, -1.531465514063894640 ) ) ;
#37685=CARTESIAN_POINT ( 'NONE',  ( 0.7681833999686451531, -81.17708333333334281, -0.9995835529977240563 ) ) ;
#37696=CARTESIAN_POINT ( 'NONE',  ( -0.03211217802971453456, -82.97766872073640343, 1.249454676527944397 ) ) ;
#37698=CARTESIAN_POINT ( 'NONE',  ( -0.1636246173744726473, -80.38541666666664298, 1.249999999999999112 ) ) ;
#37701=CARTESIAN_POINT ( 'NONE',  ( -2.500000000000000000, -80.69999999999998863, 0.000000000000000000 ) ) ;
#37711=ORIENTED_EDGE ( 'NONE', *, *, #6505, .T. ) ;
#37731=ORIENTED_EDGE ( 'NONE', *, *, #10642, .F. ) ;
#37738=CARTESIAN_POINT ( 'NONE',  ( -0.9065758875347766921, -80.54017105660118148, 0.8601027002304681979 ) ) ;
#37750=CARTESIAN_POINT ( 'NONE',  ( -0.4749605806518016893, -80.19414814864481400, -1.156137223762152111 ) ) ;
#37755=CARTESIAN_POINT ( 'NONE',  ( 1.479639340215956889, -78.11546880775445345, 0.2990852677476950605 ) ) ;
#37762=EDGE_CURVE ( 'NONE', #19162, #8320, #47121, .T. ) ;
#37768=EDGE_CURVE ( 'NONE', #44932, #36858, #43686, .T. ) ;
#37773=CARTESIAN_POINT ( 'NONE',  ( -1.250000000000001332, -82.98958333333332860, 0.1636246173744632659 ) ) ;
#37779=CARTESIAN_POINT ( 'NONE',  ( -1.223837560276999969, -82.04518551926999237, 0.5728811815464999180 ) ) ;
#37782=CARTESIAN_POINT ( 'NONE',  ( 1.217465845835394855, -82.22916666666667140, -0.3271848554490981997 ) ) ;
#37783=CARTESIAN_POINT ( 'NONE',  ( 10.14999999999999858, -87.09999999999999432, 0.000000000000000000 ) ) ;
#37797=CARTESIAN_POINT ( 'NONE',  ( -0.2267887403928895707, -81.48972645057914121, 1.230552019311672574 ) ) ;
#37803=CARTESIAN_POINT ( 'NONE',  ( 1.266435358863000182, -77.80991723433999141, -0.3269927860501000150 ) ) ;
#37827=UNCERTAINTY_MEASURE_WITH_UNIT (LENGTH_MEASURE( 1.000000000000000082E-05 ), #56019, 'distance_accuracy_value', 'NONE');
#37831=CARTESIAN_POINT ( 'NONE',  ( -1.481905647302000029, -78.36352141788999859, -0.6727694308694001091 ) ) ;
#37841=CARTESIAN_POINT ( 'NONE',  ( -0.5415696896749999656, -80.73078034499999944, 1.614471809804999936 ) ) ;
#37866=CARTESIAN_POINT ( 'NONE',  ( -0.2572323282450250659, -79.99163916602751101, 1.224162942274605426 ) ) ;
#37871=CARTESIAN_POINT ( 'NONE',  ( -0.7735022424363000582, -79.44479340558000047, 1.069754805883999849 ) ) ;
#37873=CARTESIAN_POINT ( 'NONE',  ( -0.02829167690231079030, -81.87345300400795622, -1.509943273689894339 ) ) ;
#37874=CARTESIAN_POINT ( 'NONE',  ( -0.4474063622920959604, -83.24816762388498148, 1.444966699100387997 ) ) ;
#37878=CARTESIAN_POINT ( 'NONE',  ( -0.7818257270255812852, -81.67163890709370833, -0.9757561653316191297 ) ) ;
#37881=CYLINDRICAL_SURFACE ( 'NONE', #28056, 1.250000000000000000 ) ;
#37887=VECTOR ( 'NONE', #1966, 1000.000000000000000 ) ;
#37896=ADVANCED_FACE ( 'NONE', ( #13975 ), #54754, .F. ) ;
#37905=CARTESIAN_POINT ( 'NONE',  ( 0.8987165921316000450, -79.53370706566998649, 1.306408957324000086 ) ) ;
#37909=CARTESIAN_POINT ( 'NONE',  ( 1.156695879979905417, -79.44425242284700062, -0.9743152201541099844 ) ) ;
#37919=ORIENTED_EDGE ( 'NONE', *, *, #23091, .T. ) ;
#37923=CARTESIAN_POINT ( 'NONE',  ( 1.084783777416393535, -78.39160765235115491, 0.6217191435999254168 ) ) ;
#37948=CARTESIAN_POINT ( 'NONE',  ( 0.1637460699175452006, -78.23548803879329228, -1.249514800815695104 ) ) ;
#37959=CARTESIAN_POINT ( 'NONE',  ( 0.7772493032054257345, -82.77886188811029911, -0.9788881955388119005 ) ) ;
#37964=CARTESIAN_POINT ( 'NONE',  ( 1.491636372696257151, -78.01887984504998030, 0.3555933071290897640 ) ) ;
#37965=AXIS2_PLACEMENT_3D ( 'NONE', #46355, #14444, #27437 ) ;
#37983=CARTESIAN_POINT ( 'NONE',  ( 0.2351644692787993596, -82.96014985781650353, 1.227555708270977819 ) ) ;
#37993=FILL_AREA_STYLE_COLOUR ( '', #4327 ) ;
#38001=FACE_OUTER_BOUND ( 'NONE', #33447, .T. ) ;
#38006=CARTESIAN_POINT ( 'NONE',  ( -1.458706046781999888, -81.84871131734999494, 0.8046341008317999810 ) ) ;
#38014=EDGE_LOOP ( 'NONE', ( #52700, #30298, #54731, #44409, #24753 ) ) ;
#38015=EDGE_CURVE ( 'NONE', #43389, #7477, #16912, .T. ) ;
#38027=ORIENTED_EDGE ( 'NONE', *, *, #47448, .F. ) ;
#38030=CARTESIAN_POINT ( 'NONE',  ( 0.8712539910064536208, -80.41418404898685424, 0.8959414737579669552 ) ) ;
#38045=CARTESIAN_POINT ( 'NONE',  ( -0.1208381380149903539, -78.73118724211690278, 1.533608188374127712 ) ) ;
#38060=CARTESIAN_POINT ( 'NONE',  ( -1.403176326237301152, -80.71958272795352229, 0.5630851912215953936 ) ) ;
#38074=CARTESIAN_POINT ( 'NONE',  ( 1.250000000000000000, -82.24999999999998579, 0.000000000000000000 ) ) ;
#38085=EDGE_CURVE ( 'NONE', #7670, #31856, #36630, .T. ) ;
#38087=CARTESIAN_POINT ( 'NONE',  ( 0.8783140891125981176, -81.41347531358452727, 0.8889992555315535672 ) ) ;
#38090=CARTESIAN_POINT ( 'NONE',  ( 0.7676033376664712637, -82.27773949277477072, -0.9994747690136148721 ) ) ;
#38093=CARTESIAN_POINT ( 'NONE',  ( 1.357743527867999900, -78.86943374892000236, -0.4206474370307000110 ) ) ;
#38119=CARTESIAN_POINT ( 'NONE',  ( -0.9347040216968000026, -78.81250873020999848, 1.332288049216000081 ) ) ;
#38149=CARTESIAN_POINT ( 'NONE',  ( -0.2201363562291999698, -79.46327907014000402, -1.483758735329000045 ) ) ;
#38153=CARTESIAN_POINT ( 'NONE',  ( 1.343749999883000035, -77.90625000011999646, 3.156563468101999814E-09 ) ) ;
#38161=CARTESIAN_POINT ( 'NONE',  ( -1.250754810632284109, -79.07932702254176149, 0.3272114123015318898 ) ) ;
#38162=CARTESIAN_POINT ( 'NONE',  ( 1.542660238577055365, -82.09427013190894229, -0.1073020398081418886 ) ) ;
#38163=CARTESIAN_POINT ( 'NONE',  ( 0.1190605478174616982, -79.73281567795952185, -1.244496223888971187 ) ) ;
#38168=( NAMED_UNIT ( * ) SI_UNIT ( $, .STERADIAN. ) SOLID_ANGLE_UNIT ( ) );
#38175=VECTOR ( 'NONE', #52307, 1000.000000000000000 ) ;
#38197=CARTESIAN_POINT ( 'NONE',  ( -0.5437916395094000155, -79.30212327692998997, -1.373128015768000143 ) ) ;
#38204=CARTESIAN_POINT ( 'NONE',  ( 1.250000000000000000, -81.24999999999998579, 0.000000000000000000 ) ) ;
#38217=CARTESIAN_POINT ( 'NONE',  ( 1.201809672664051476, -78.37247684905804590, 0.3447628147767792806 ) ) ;
#38233=CARTESIAN_POINT ( 'NONE',  ( -1.217465845835394411, -82.52083333333331439, -0.3271848554491003647 ) ) ;
#38235=LINE ( 'NONE', #56256, #8936 ) ;
#38251=CARTESIAN_POINT ( 'NONE',  ( -0.3277207512123008204, -82.70464360152637084, -1.218374181744829698 ) ) ;
#38255=CARTESIAN_POINT ( 'NONE',  ( -1.184592955636749378, -79.57468984537729284, 0.3985202767571495164 ) ) ;
#38256=CARTESIAN_POINT ( 'NONE',  ( -0.05333894232729029239, -79.12800920574750307, 1.532713344806896361 ) ) ;
#38263=FACE_OUTER_BOUND ( 'NONE', #30922, .T. ) ;
#38266=CARTESIAN_POINT ( 'NONE',  ( 1.250000000000000222, -81.23958333333334281, -0.1636246173744659582 ) ) ;
#38275=CARTESIAN_POINT ( 'NONE',  ( -0.5301937742937986586, -83.00996881353496804, 1.132399620896593850 ) ) ;
#38299=CARTESIAN_POINT ( 'NONE',  ( 1.541440768196999933, -82.66978111377999028, 0.6318380856084999664 ) ) ;
#38317=CARTESIAN_POINT ( 'NONE',  ( 0.9476663237611181456, -80.40730976135888852, 0.8183754900101951613 ) ) ;
#38342=EDGE_CURVE ( 'NONE', #54925, #57688, #11667, .T. ) ;
#38347=CARTESIAN_POINT ( 'NONE',  ( -1.316334517949519833, -80.29447262625133419, -0.8125667813490581315 ) ) ;
#38361=EDGE_CURVE ( 'NONE', #19814, #19162, #34130, .T. ) ;
#38373=CARTESIAN_POINT ( 'NONE',  ( 0.7987623000872553503, -81.42017824848964835, 0.9617713037012455279 ) ) ;
#38382=CARTESIAN_POINT ( 'NONE',  ( 0.6295237254636211199, -78.33333333333334281, 1.092232985442824322 ) ) ;
#38393=EDGE_CURVE ( 'NONE', #12955, #10981, #31228, .T. ) ;
#38401=ORIENTED_EDGE ( 'NONE', *, *, #22513, .F. ) ;
#38411=CARTESIAN_POINT ( 'NONE',  ( 0.1660104325307999729, -78.19647670854999433, 1.618982269915999916 ) ) ;
#38420=CARTESIAN_POINT ( 'NONE',  ( -0.7205381521189000438, -80.92025799034000499, -1.542932836074000003 ) ) ;
#38455=CARTESIAN_POINT ( 'NONE',  ( -1.503028869898288322, -81.84122243630122284, 0.1554063332427757516 ) ) ;
#38458=CARTESIAN_POINT ( 'NONE',  ( 0.6359605339382402578, -79.76804382808089144, -1.076489120615609307 ) ) ;
#38467=ORIENTED_EDGE ( 'NONE', *, *, #52233, .T. ) ;
#38471=CARTESIAN_POINT ( 'NONE',  ( 3.425937024882473377E-06, -77.82827182887865547, -1.422119424801547627 ) ) ;
#38475=ADVANCED_FACE ( 'NONE', ( #49267 ), #14468, .F. ) ;
#38489=CARTESIAN_POINT ( 'NONE',  ( 0.8701072296501000114, -80.10229747532000033, 1.463806805601000072 ) ) ;
#38496=CARTESIAN_POINT ( 'NONE',  ( -10.14999999999999858, -86.39999999999999147, 0.000000000000000000 ) ) ;
#38509=CARTESIAN_POINT ( 'NONE',  ( 0.8464868648045736910, -78.41589811855170922, 0.9196883286881438746 ) ) ;
#38522=CARTESIAN_POINT ( 'NONE',  ( -0.9747649511251000876, -79.25484333926999625, 1.348101445433000034 ) ) ;
#38527=DIRECTION ( 'NONE',  ( -1.000000000000000000, 0.000000000000000000, 0.000000000000000000 ) ) ;
#38548=CARTESIAN_POINT ( 'NONE',  ( 1.301538823741287043, -79.04398425417873852, 0.8091645586960490855 ) ) ;
#38555=CYLINDRICAL_SURFACE ( 'NONE', #42954, 1.250000000000000000 ) ;
#38557=CARTESIAN_POINT ( 'NONE',  ( -1.168006160022410755, -81.29468525113304622, 0.9590183425694498442 ) ) ;
#38601=CARTESIAN_POINT ( 'NONE',  ( -1.112403273011567162, -80.63938135327609302, -0.5932074133774921654 ) ) ;
#38609=CARTESIAN_POINT ( 'NONE',  ( -0.2479305816249914307, -80.49105691730132150, 1.225069668416682855 ) ) ;
#38612=EDGE_LOOP ( 'NONE', ( #21675, #37919, #52941, #15971, #21976, #16656, #28149, #38401, #1683, #6380, #9202 ) ) ;
#38638=CARTESIAN_POINT ( 'NONE',  ( -1.216363293580657867, -80.80055608065869421, -0.8954020866757705921 ) ) ;
#38662=CARTESIAN_POINT ( 'NONE',  ( 0.8729495473840620523, -81.41394231601826448, 0.8942802001960106217 ) ) ;
#38663=CARTESIAN_POINT ( 'NONE',  ( -1.445929428138999828, -80.28824903432000326, 0.8273736140038000508 ) ) ;
#38667=CARTESIAN_POINT ( 'NONE',  ( 1.218263462486750326, -82.32982652230532494, -0.3278909641266472552 ) ) ;
#38700=CARTESIAN_POINT ( 'NONE',  ( 1.169626569868999821, -78.14079513876998817, 1.131652196797999999 ) ) ;
#38703=CARTESIAN_POINT ( 'NONE',  ( -9.000000000000000000, -92.39999999999999147, 0.000000000000000000 ) ) ;
#38710=CARTESIAN_POINT ( 'NONE',  ( -1.436931233250000162, -79.97318471100000181, -0.3027821832741999786 ) ) ;
#38715=CARTESIAN_POINT ( 'NONE',  ( 1.611423453808999984, -81.48158470040999646, 0.4225784326546000447 ) ) ;
#38744=CARTESIAN_POINT ( 'NONE',  ( -0.2342375876246420574, -82.23597684144930042, 1.531779633465825130 ) ) ;
#38745=CARTESIAN_POINT ( 'NONE',  ( 0.3485046458849904161, -79.74754369683780908, -1.203412226622470049 ) ) ;
#38752=VERTEX_POINT ( 'NONE', #51325 ) ;
#38770=AXIS2_PLACEMENT_3D ( 'NONE', #37061, #10804, #51253 ) ;
#38777=CARTESIAN_POINT ( 'NONE',  ( 2.500000000000000000, -77.69999999999998863, 0.000000000000000000 ) ) ;
#38778=CARTESIAN_POINT ( 'NONE',  ( -0.5880095755872802865, -79.65680747369806625, 1.391623923462375068 ) ) ;
#38792=CARTESIAN_POINT ( 'NONE',  ( 0.000000000000000000, -80.79999999999999716, 0.000000000000000000 ) ) ;
#38794=CARTESIAN_POINT ( 'NONE',  ( 1.116474234542908839, -78.38743099930486835, 0.5628238750089364917 ) ) ;
#38810=CARTESIAN_POINT ( 'NONE',  ( -1.250000000000000000, -82.09999999999999432, 0.000000000000000000 ) ) ;
#38811=CARTESIAN_POINT ( 'NONE',  ( -0.7159780689917000229, -78.41961979257999360, -1.501637300520000107 ) ) ;
#38820=CARTESIAN_POINT ( 'NONE',  ( -1.216845017716923438, -78.12095369619891017, -0.3271854394012499445 ) ) ;
#38824=B_SPLINE_CURVE_WITH_KNOTS ( 'NONE', 3,
 ( #27268, #45304, #22258, #31984, #741, #35534, #36716, #40273, #8391, #53562, #13101, #58284, #17847, #24013, #28135, #42327, #1896, #50316 ),
 .UNSPECIFIED., .F., .F.,
 ( 4, 2, 2, 2, 2, 2, 2, 2, 4 ),
 ( 0.000000000000000000, 0.1250000000000000833, 0.2500000000000001110, 0.3750000000000000000, 0.4999999999999999445, 0.6249999999999998890, 0.7499999999999997780, 0.8749999999999998890, 1.000000000000000000 ),
 .UNSPECIFIED. ) ;
#38837=CARTESIAN_POINT ( 'NONE',  ( 1.127238840805811826, -79.38609853011139705, 0.5400240268550191569 ) ) ;
#38838=CARTESIAN_POINT ( 'NONE',  ( 0.1063340454544151326, -78.11970978693250345, 1.529732311428813274 ) ) ;
#38856=CARTESIAN_POINT ( 'NONE',  ( 1.250000000000000000, -80.25000000000000000, 0.000000000000000000 ) ) ;
#38892=CARTESIAN_POINT ( 'NONE',  ( -0.002548132935883858086, -80.47577112694141022, 1.249635788585080176 ) ) ;
#38913=CARTESIAN_POINT ( 'NONE',  ( -1.250000000000000000, -83.49999999999998579, 0.000000000000000000 ) ) ;
#38920=CARTESIAN_POINT ( 'NONE',  ( 0.8406634254895485325, -80.92201610971640946, -1.255420779031111822 ) ) ;
#38924=PLANE ( 'NONE',  #45510 ) ;
#38930=CARTESIAN_POINT ( 'NONE',  ( 0.5557217581696000108, -82.48745749870199973, 1.359272403504999893 ) ) ;
#38952=CARTESIAN_POINT ( 'NONE',  ( -0.5298108134926000634, -80.78957986396000024, 1.579417458585999912 ) ) ;
#38966=CARTESIAN_POINT ( 'NONE',  ( -0.4913337550651999952, -78.24025491156999124, -1.333792686520999915 ) ) ;
#39000=CARTESIAN_POINT ( 'NONE',  ( 0.5132697287564000899, -81.97938944371999526, -1.623690596030999744 ) ) ;
#39001=CARTESIAN_POINT ( 'NONE',  ( -0.4036326496859999891, -80.28882331289000263, 1.533452771621000021 ) ) ;
#39006=CARTESIAN_POINT ( 'NONE',  ( -1.324613189995999862, -83.25004272349499956, -0.7038465009425000085 ) ) ;
#39018=CARTESIAN_POINT ( 'NONE',  ( -0.7803569495551999635, -81.91581342370000129, -1.471836271561000054 ) ) ;
#39034=CARTESIAN_POINT ( 'NONE',  ( 1.250000000000000000, -78.25000000000000000, 0.000000000000000000 ) ) ;
#39035=DIRECTION ( 'NONE',  ( 1.000000000000000000, 0.000000000000000000, 0.000000000000000000 ) ) ;
#39036=CARTESIAN_POINT ( 'NONE',  ( 0.8726123492689907835, -82.02341677713879164, -1.234002077154575883 ) ) ;
#39037=CARTESIAN_POINT ( 'NONE',  ( 0.08452963021239402741, -79.73065581606381613, -1.247426360802352141 ) ) ;
#39044=ORIENTED_EDGE ( 'NONE', *, *, #9490, .F. ) ;
#39062=CARTESIAN_POINT ( 'NONE',  ( 1.623222485893000000, -80.54441198108999345, 0.5147482071316000773 ) ) ;
#39096=CONICAL_SURFACE ( 'NONE', #36273, 2.949999999500999781, 0.7853981633972997312 ) ;
#39110=CARTESIAN_POINT ( 'NONE',  ( 1.250000000000000000, -81.74999999999998579, 0.000000000000000000 ) ) ;
#39124=CARTESIAN_POINT ( 'NONE',  ( 0.2746856994466179147, -82.74303240917123503, -1.219238289928273211 ) ) ;
#39135=AXIS2_PLACEMENT_3D ( 'NONE', #33197, #46533, #10498 ) ;
#39179=CARTESIAN_POINT ( 'NONE',  ( 1.250000000000000000, -80.34999999999999432, 0.000000000000000000 ) ) ;
#39197=DIRECTION ( 'NONE',  ( 1.000000000000000000, 0.000000000000000000, 0.000000000000000000 ) ) ;
#39206=B_SPLINE_CURVE_WITH_KNOTS ( 'NONE', 3,
 ( #27379, #45416, #27668, #37113 ),
 .UNSPECIFIED., .F., .F.,
 ( 4, 4 ),
 ( 0.000000000000000000, 1.000000000000000000 ),
 .UNSPECIFIED. ) ;
#39207=CARTESIAN_POINT ( 'NONE',  ( 0.7440580446819816673, -81.08396281512723647, 1.316460893200364746 ) ) ;
#39216=ADVANCED_FACE ( 'NONE', ( #2528, #19653 ), #20531, .F. ) ;
#39219=CARTESIAN_POINT ( 'NONE',  ( 1.467208996055999748, -82.48761497235999229, 0.6014104092625999209 ) ) ;
#39236=CARTESIAN_POINT ( 'NONE',  ( 1.250000000000000000, -79.75000000000000000, 0.000000000000000000 ) ) ;
#39238=CARTESIAN_POINT ( 'NONE',  ( 1.356773869401999955, -79.47112212912999496, -0.9668579442890000708 ) ) ;
#39243=CARTESIAN_POINT ( 'NONE',  ( -0.6295237254636286695, -78.41666666666665719, 1.092232985442819881 ) ) ;
#39250=CARTESIAN_POINT ( 'NONE',  ( 0.4280957282384999507, -78.29268648134998898, -1.355413529770999936 ) ) ;
#39281=EDGE_CURVE ( 'NONE', #23434, #28137, #194, .T. ) ;
#39287=FACE_OUTER_BOUND ( 'NONE', #38612, .T. ) ;
#39288=CARTESIAN_POINT ( 'NONE',  ( -1.551612880221999946, -79.90986802222998620, -0.3269472641410000047 ) ) ;
#39306=CARTESIAN_POINT ( 'NONE',  ( -1.374853770045000090, -81.30921723553998959, -0.7192078502473999713 ) ) ;
#39316=CARTESIAN_POINT ( 'NONE',  ( 0.8664535991523154568, -79.91447041001134721, 0.9006602674240518080 ) ) ;
#39322=CARTESIAN_POINT ( 'NONE',  ( 0.000000000000000000, -92.39999999999999147, 0.000000000000000000 ) ) ;
#39324=CARTESIAN_POINT ( 'NONE',  ( -1.389164232317718017, -81.88171006759844772, -0.5985393350652561395 ) ) ;
#39326=CARTESIAN_POINT ( 'NONE',  ( -0.4417226670687336432, -79.69665877900507667, -1.169169109811868612 ) ) ;
#39330=ORIENTED_EDGE ( 'NONE', *, *, #9210, .F. ) ;
#39341=B_SPLINE_CURVE_WITH_KNOTS ( 'NONE', 3,
 ( #10928, #37773, #55794, #15344, #10050, #28909, #9752, #20073, #56084, #18902, #32164, #27738, #37187, #45785, #5320, #41919, #23328, #36894 ),
 .UNSPECIFIED., .F., .F.,
 ( 4, 2, 2, 2, 2, 2, 2, 2, 4 ),
 ( 0.000000000000000000, 0.1249999999999999722, 0.2500000000000000000, 0.3750000000000000000, 0.5000000000000001110, 0.6250000000000001110, 0.7500000000000000000, 0.8750000000000000000, 1.000000000000000000 ),
 .UNSPECIFIED. ) ;
#39361=ORIENTED_EDGE ( 'NONE', *, *, #32827, .T. ) ;
#39393=CARTESIAN_POINT ( 'NONE',  ( -0.01871105017136468623, -81.97680572310699176, 1.249633071440004350 ) ) ;
#39402=CARTESIAN_POINT ( 'NONE',  ( 0.000000000000000000, -77.50000000000000000, 0.000000000000000000 ) ) ;
#39406=EDGE_LOOP ( 'NONE', ( #32487, #56149, #11111, #49688 ) ) ;
#39423=CARTESIAN_POINT ( 'NONE',  ( 0.000000000000000000, -80.69999999999998863, 0.000000000000000000 ) ) ;
#39429=CARTESIAN_POINT ( 'NONE',  ( -0.3439666625990999704, -79.97550662411998701, 1.306773950318999900 ) ) ;
#39431=CARTESIAN_POINT ( 'NONE',  ( -1.250000000000000000, -82.49999999999998579, 0.000000000000000000 ) ) ;
#39444=ADVANCED_FACE ( 'NONE', ( #51976 ), #36043, .T. ) ;
#39467=EDGE_LOOP ( 'NONE', ( #46845, #44703, #45893, #39044 ) ) ;
#39475=CARTESIAN_POINT ( 'NONE',  ( 1.149310424350558080, -80.38227707828973223, 0.4913328182984957326 ) ) ;
#39482=ORIENTED_EDGE ( 'NONE', *, *, #41797, .T. ) ;
#39490=CARTESIAN_POINT ( 'NONE',  ( -1.508524907456192610, -77.84776514064024866, 0.03467181534751852950 ) ) ;
#39500=CARTESIAN_POINT ( 'NONE',  ( -1.249999999999999778, -78.51041666666664298, -0.1636246173744686228 ) ) ;
#39501=CARTESIAN_POINT ( 'NONE',  ( -1.177869840716120997, -80.29261637651916317, 1.006895591056990558 ) ) ;
#39511=CARTESIAN_POINT ( 'NONE',  ( -1.186490757027999887, -81.09779729262000103, -0.2694786029208000033 ) ) ;
#39514=CARTESIAN_POINT ( 'NONE',  ( -1.416666666666666741, -83.20000000000000284, 0.000000000000000000 ) ) ;
#39532=ORIENTED_EDGE ( 'NONE', *, *, #43576, .F. ) ;
#39543=CARTESIAN_POINT ( 'NONE',  ( -1.329574456303999952, -77.62855326413999535, 0.2546955586738999799 ) ) ;
#39544=VERTEX_POINT ( 'NONE', #58123 ) ;
#39572=CARTESIAN_POINT ( 'NONE',  ( -0.9269137457058925778, -83.04216970360333505, 0.8380920112027951951 ) ) ;
#39577=CARTESIAN_POINT ( 'NONE',  ( 0.2491193812340000147, -79.53091273156999819, -1.565693046525999943 ) ) ;
#39581=CARTESIAN_POINT ( 'NONE',  ( -0.7572724432162000197, -83.18294061714399845, 1.483977110291999857 ) ) ;
#39593=CARTESIAN_POINT ( 'NONE',  ( 0.6062141276560999437, -82.48424635968999041, -1.551696954864999922 ) ) ;
#39602=CARTESIAN_POINT ( 'NONE',  ( 0.3635088733166961794, -79.95197095518092567, 1.195828664671276576 ) ) ;
#39629=EDGE_LOOP ( 'NONE', ( #11396, #2332, #24449, #51957 ) ) ;
#39643=AXIS2_PLACEMENT_3D ( 'NONE', #34866, #52896, #8015 ) ;
#39646=ADVANCED_FACE ( 'NONE', ( #14898 ), #20053, .T. ) ;
#39672=CARTESIAN_POINT ( 'NONE',  ( 1.142430001277040308, -81.88337218985522270, 0.5072272210963466588 ) ) ;
#39673=CARTESIAN_POINT ( 'NONE',  ( 1.659612711100000082, -78.08553037389999929, 0.1150004796074000080 ) ) ;
#39679=CARTESIAN_POINT ( 'NONE',  ( -1.134730520616228144, -81.37330620173663931, -0.9788030900385257249 ) ) ;
#39713=AXIS2_PLACEMENT_3D ( 'NONE', #39402, #35831, #23140 ) ;
#39775=PRODUCT_DEFINITION ( 'UNKNOWN', '', #30046, #30961 ) ;
#39782=CARTESIAN_POINT ( 'NONE',  ( 1.152612928993206332, -80.65700505819430077, 1.031344352619617766 ) ) ;
#39785=DIRECTION ( 'NONE',  ( 0.000000000000000000, -1.000000000000000000, 2.812564995716999917E-14 ) ) ;
#39792=CARTESIAN_POINT ( 'NONE',  ( 0.4426188121580000301, -81.79270613248999666, -1.400191678299000042 ) ) ;
#39832=CARTESIAN_POINT ( 'NONE',  ( 0.5247358252921234811, -80.25970768809875722, -1.134507553617768671 ) ) ;
#39845=FACE_OUTER_BOUND ( 'NONE', #19889, .T. ) ;
#39854=CARTESIAN_POINT ( 'NONE',  ( -1.160500472347511636, -83.06980021841565076, 0.4644083125726469197 ) ) ;
#39859=CARTESIAN_POINT ( 'NONE',  ( 0.5343721329914999929, -82.61129654213999629, -1.367806479096000061 ) ) ;
#39860=CARTESIAN_POINT ( 'NONE',  ( -0.5035993198763999423, -79.55212327692998997, -1.271638408173999979 ) ) ;
#39861=CARTESIAN_POINT ( 'NONE',  ( -0.4635254915624000271, -77.75000000000000000, 1.426584774443000025 ) ) ;
#39878=CARTESIAN_POINT ( 'NONE',  ( -1.510823314100999903, -83.34742229952999537, -0.3534059060544000319 ) ) ;
#39912=CARTESIAN_POINT ( 'NONE',  ( 1.150218351780601056, -79.38243505016826873, 0.4888114725149512174 ) ) ;
#39922=CARTESIAN_POINT ( 'NONE',  ( -1.472167250137000005, -78.74622289817000365, -0.6938203229310999642 ) ) ;
#39941=ORIENTED_EDGE ( 'NONE', *, *, #26975, .F. ) ;
#39946=DIRECTION ( 'NONE',  ( 0.000000000000000000, 0.000000000000000000, -1.000000000000000000 ) ) ;
#39961=CARTESIAN_POINT ( 'NONE',  ( 0.8603538941506917448, -81.91514795278682470, 0.9063378267799424570 ) ) ;
#39962=CARTESIAN_POINT ( 'NONE',  ( 1.113300400990999917, -78.20452863244999264, 1.077154774809000015 ) ) ;
#39970=CARTESIAN_POINT ( 'NONE',  ( 1.049808574365361347, -81.80446097931094585, -0.6784272128118777889 ) ) ;
#40030=CARTESIAN_POINT ( 'NONE',  ( 1.092232985442820992, -82.29166666666665719, 0.6295237254636267821 ) ) ;
#40038=CARTESIAN_POINT ( 'NONE',  ( -1.500000000366989328, -77.74999999999998579, 0.3141592638904139312 ) ) ;
#40045=ORIENTED_EDGE ( 'NONE', *, *, #24662, .F. ) ;
#40066=CARTESIAN_POINT ( 'NONE',  ( -1.500000000000000000, -83.34999999999999432, 0.000000000000000000 ) ) ;
#40074=CARTESIAN_POINT ( 'NONE',  ( 1.505169111093489498, -81.09224709464676550, -0.1340111490899882907 ) ) ;
#40084=CARTESIAN_POINT ( 'NONE',  ( 0.5132697287564000899, -81.91933951002999947, -1.623690596030999744 ) ) ;
#40086=CARTESIAN_POINT ( 'NONE',  ( -0.7681833999686432657, -82.07291666666665719, -0.9995835529977258327 ) ) ;
#40090=ADVANCED_FACE ( 'NONE', ( #4749 ), #27457, .T. ) ;
#40102=ORIENTED_EDGE ( 'NONE', *, *, #8548, .F. ) ;
#40107=CARTESIAN_POINT ( 'NONE',  ( -0.8981901762082999952, -79.96851006753000490, -1.403037214508999986 ) ) ;
#40122=CARTESIAN_POINT ( 'NONE',  ( 0.9401231181983999985, -77.88411904209999648, -1.213240629208000243 ) ) ;
#40127=CARTESIAN_POINT ( 'NONE',  ( 1.157786043506160212, -80.31939170094496205, -0.4709745549768553086 ) ) ;
#40153=CARTESIAN_POINT ( 'NONE',  ( 1.261625697157999992, -81.66390831549000495, -0.7514603626543999715 ) ) ;
#40171=CARTESIAN_POINT ( 'NONE',  ( -1.519662023741000123, -82.86320165035199636, -0.6825586799200999977 ) ) ;
#40202=VERTEX_POINT ( 'NONE', #1212 ) ;
#40210=CARTESIAN_POINT ( 'NONE',  ( 1.114061420507061140, -79.38800613273430429, 0.5663899713086829601 ) ) ;
#40223=CARTESIAN_POINT ( 'NONE',  ( 1.250000000000000222, -78.23958333333328596, -0.1636246173744659582 ) ) ;
#40258=CARTESIAN_POINT ( 'NONE',  ( 0.6820633866021539315, -81.92923038876949704, 1.047497107621460088 ) ) ;
#40259=CARTESIAN_POINT ( 'NONE',  ( 1.343706126530000100, -78.02984880411999313, -0.9808119522502999343 ) ) ;
#40261=CARTESIAN_POINT ( 'NONE',  ( 1.097245158776866569, -82.56172650200396390, 1.088114895880704092 ) ) ;
#40266=EDGE_CURVE ( 'NONE', #13108, #35472, #49326, .T. ) ;
#40269=CARTESIAN_POINT ( 'NONE',  ( 0.4820398299941640596, -81.75661953861411746, -1.153239258334429751 ) ) ;
#40273=CARTESIAN_POINT ( 'NONE',  ( 0.3271848554491016414, -80.14583333333330017, -1.217465845835393967 ) ) ;
#40275=ORIENTED_EDGE ( 'NONE', *, *, #53583, .T. ) ;
#40279=VECTOR ( 'NONE', #31431, 1000.000000000000114 ) ;
#40343=ORIENTED_EDGE ( 'NONE', *, *, #8548, .T. ) ;
#40352=EDGE_CURVE ( 'NONE', #36547, #57912, #57849, .T. ) ;
#40362=DIRECTION ( 'NONE',  ( 0.000000000000000000, 0.000000000000000000, -1.000000000000000000 ) ) ;
#40368=CARTESIAN_POINT ( 'NONE',  ( 0.000000000000000000, -87.20000000000000284, 0.000000000000000000 ) ) ;
#40380=CARTESIAN_POINT ( 'NONE',  ( -1.498818208256021745, -80.83919939903495333, 0.1937138382002916992 ) ) ;
#40383=EDGE_CURVE ( 'NONE', #12786, #53705, #31814, .T. ) ;
#40390=CARTESIAN_POINT ( 'NONE',  ( -1.388458563311000038, -81.66654517592999696, 0.7658850185041000680 ) ) ;
#40427=CARTESIAN_POINT ( 'NONE',  ( -1.196135072002999955, -78.20959357977000082, 1.134084288239000093 ) ) ;
#40430=CARTESIAN_POINT ( 'NONE',  ( 0.6031251352556811218, -80.26544605463739401, -1.094772290821791838 ) ) ;
#40446=VECTOR ( 'NONE', #41324, 1000.000000000000000 ) ;
#40452=CARTESIAN_POINT ( 'NONE',  ( -1.165193207555734078, -83.07060353884618564, 0.4526761131825299822 ) ) ;
#40456=CARTESIAN_POINT ( 'NONE',  ( -0.5277720668919000380, -82.29534299292998867, 1.495277019118000039 ) ) ;
#40457=CARTESIAN_POINT ( 'NONE',  ( 1.092255414008205028, -78.80861679417924393, -0.6293616401131961746 ) ) ;
#40458=CARTESIAN_POINT ( 'NONE',  ( 1.250000000000000000, -79.84999999999999432, 0.000000000000000000 ) ) ;
#40486=CARTESIAN_POINT ( 'NONE',  ( 0.6050660503295083315, -81.50719947809898258, -1.386332957043676428 ) ) ;
#40514=EDGE_CURVE ( 'NONE', #48338, #19028, #21781, .T. ) ;
#40522=CARTESIAN_POINT ( 'NONE',  ( 0.9995835529977264988, -78.19791666666665719, -0.7681833999686417114 ) ) ;
#40541=LINE ( 'NONE', #44975, #30095 ) ;
#40553=CIRCLE ( 'NONE', #49960, 1.750000000000000000 ) ;
#40559=CARTESIAN_POINT ( 'NONE',  ( 1.356773869401999955, -79.41190580526000531, -0.9668579442890000708 ) ) ;
#40560=CARTESIAN_POINT ( 'NONE',  ( 0.3904537433033999916, -78.53861805112998695, -1.499081755109000103 ) ) ;
#40562=CARTESIAN_POINT ( 'NONE',  ( -1.214616973637322683, -83.19939165455916452, 0.8969727609832535142 ) ) ;
#40563=CARTESIAN_POINT ( 'NONE',  ( 0.000000000000000000, -87.09999999999999432, 0.000000000000000000 ) ) ;
#40678=CARTESIAN_POINT ( 'NONE',  ( -1.250000000000001332, -80.98958333333331439, 0.1636246173744632659 ) ) ;
#40681=CARTESIAN_POINT ( 'NONE',  ( 0.8412929767025426608, -81.02139373987667170, -1.256298128065854725 ) ) ;
#40682=CARTESIAN_POINT ( 'NONE',  ( -0.9088528845057587402, -78.54008175705185124, 0.8581086277074990720 ) ) ;
#40724=CARTESIAN_POINT ( 'NONE',  ( -1.527202200078999983, -78.19870846077999715, 0.1530789007224999942 ) ) ;
#40728=CARTESIAN_POINT ( 'NONE',  ( 1.250000000000000000, -80.34999999999999432, 0.000000000000000000 ) ) ;
#40747=CARTESIAN_POINT ( 'NONE',  ( -1.167634245779999969, -83.49552555368299522, -0.6204341648412000643 ) ) ;
#40768=CARTESIAN_POINT ( 'NONE',  ( 0.3980000373821807047, -77.96875000003851142, 1.234183929323941831 ) ) ;
#40775=CARTESIAN_POINT ( 'NONE',  ( -0.8449747453178998446, -81.53464264722271082, 0.9222519907885509127 ) ) ;
#40810=CARTESIAN_POINT ( 'NONE',  ( -1.573065832928000063, -78.69054132838999749, 0.4172852021023999991 ) ) ;
#40815=CARTESIAN_POINT ( 'NONE',  ( -0.6295237254636235624, -78.08333333333331439, -1.092232985442822990 ) ) ;
#40850=CARTESIAN_POINT ( 'NONE',  ( -1.529754383668999962, -81.30273936731998674, -0.6588408878327000062 ) ) ;
#40851=CARTESIAN_POINT ( 'NONE',  ( -1.524425929186000062, -77.86280409478000308, -0.6660453670107999713 ) ) ;
#40853=CARTESIAN_POINT ( 'NONE',  ( 0.3892601172833429768, -82.89574158191382480, -1.460010013733279433 ) ) ;
#40887=CARTESIAN_POINT ( 'NONE',  ( 0.2307066564514000107, -79.28091273156999819, -1.449970716867000187 ) ) ;
#40925=CARTESIAN_POINT ( 'NONE',  ( -1.250000000000000000, -82.49999999999998579, 0.000000000000000000 ) ) ;
#40954=B_SPLINE_CURVE_WITH_KNOTS ( 'NONE', 3,
 ( #57978, #9562, #26665, #23133, #40562, #48838, #18131, #45590, #36126, #5135, #4253, #3949, #54142, #13683, #50016, #4844, #13092, #17533, #31973, #27546, #35524, #17239, #13978, #40853, #445, #31089, #22551, #12806, #58274, #41141, #54442, #35226, #31680, #49126, #26378, #22250, #53257, #17837, #53553, #35825, #30805, #18424, #53854, #4549, #40261, #31386, #49427, #8978, #26963, #9269, #44993, #27254, #15445, #5415, #9856, #18712, #24304, #47054, #50600, #27838, #19579, #36706, #33439, #50306, #55302, #19880, #23713, #55893, #41435, #37873, #19002, #10435, #45883, #54721, #6583, #55010, #51475, #15144, #19294, #46767, #28715, #14558, #23423, #10149, #24595, #1301, #36994, #37286, #11032, #29015, #42318, #732, #51182, #14264, #5702, #32552, #6289, #1886, #28126, #1021, #32260, #46176, #41723, #14848, #32842, #50889, #28420 ),
 .UNSPECIFIED., .F., .F.,
 ( 4, 2, 2, 2, 2, 2, 1, 2, 2, 2, 2, 2, 2, 2, 2, 2, 2, 2, 2, 2, 2, 2, 2, 2, 2, 2, 2, 1, 2, 2, 2, 2, 2, 2, 2, 2, 2, 2, 2, 2, 2, 2, 2, 2, 2, 2, 2, 2, 1, 2, 2, 2, 2, 2, 4 ),
 ( 0.000000000000000000, 0.01562499999999999653, 0.03125000000000000000, 0.04687500000000000694, 0.06250000000000001388, 0.07812500000000002776, 0.09375000000000002776, 0.1093750000000000416, 0.1250000000000000555, 0.1406250000000000555, 0.1562500000000000555, 0.1718750000000000555, 0.1875000000000000278, 0.2031250000000000278, 0.2187500000000000278, 0.2343750000000000278, 0.2500000000000000555, 0.2656250000000000555, 0.2812500000000000555, 0.2968750000000000555, 0.3125000000000000555, 0.3281250000000000555, 0.3437500000000000555, 0.3750000000000000000, 0.4062500000000000000, 0.4375000000000000000, 0.4687500000000000000, 0.5000000000000000000, 0.5312500000000000000, 0.5625000000000000000, 0.5937500000000000000, 0.6250000000000000000, 0.6562500000000000000, 0.6718750000000000000, 0.6875000000000000000, 0.7031250000000000000, 0.7187500000000000000, 0.7343750000000000000, 0.7499999999999998890, 0.7656249999999998890, 0.7812499999999998890, 0.7968749999999998890, 0.8124999999999998890, 0.8281249999999998890, 0.8437499999999998890, 0.8593749999999998890, 0.8749999999999998890, 0.8906249999999998890, 0.9062499999999998890, 0.9218749999999998890, 0.9374999999999998890, 0.9531249999999998890, 0.9687499999999998890, 0.9843749999999998890, 1.000000000000000000 ),
 .UNSPECIFIED. ) ;
#40973=CARTESIAN_POINT ( 'NONE',  ( 0.7095316881522687469, -79.51322947404737818, -1.334021238738027249 ) ) ;
#40974=CARTESIAN_POINT ( 'NONE',  ( -0.05678956088018663473, -78.47885428363976246, 1.248697955453646147 ) ) ;
#40977=CARTESIAN_POINT ( 'NONE',  ( -1.250000000000000000, -80.49999999999998579, 0.000000000000000000 ) ) ;
#40982=CARTESIAN_POINT ( 'NONE',  ( 0.5386432692752000095, -83.11936459712099179, 1.615427185862999826 ) ) ;
#41009=CARTESIAN_POINT ( 'NONE',  ( -1.167939344301158755, -80.57113232371381173, 0.4455473596557876781 ) ) ;
#41015=CARTESIAN_POINT ( 'NONE',  ( -0.5305471585600000095, -78.30357160033999264, -1.440242834216999945 ) ) ;
#41019=CARTESIAN_POINT ( 'NONE',  ( 1.248546286058870969, -80.34460560522650496, -0.09467261385860081813 ) ) ;
#41033=EDGE_CURVE ( 'NONE', #38752, #48909, #4954, .T. ) ;
#41042=CARTESIAN_POINT ( 'NONE',  ( 1.318896022268000179, -83.24288869324199425, 0.6457249424517998992 ) ) ;
#41044=CARTESIAN_POINT ( 'NONE',  ( -1.125831293927000099, -79.97334218465999811, 0.7473110439769999891 ) ) ;
#41045=CARTESIAN_POINT ( 'NONE',  ( -0.3271848554491046945, -79.39583333333331439, 1.217465845835393301 ) ) ;
#41076=CONICAL_SURFACE ( 'NONE', #50528, 1.546875000130000011, 0.7853981633972997312 ) ;
#41101=CARTESIAN_POINT ( 'NONE',  ( -0.9156221410628999635, -78.19294195445999662, 1.345473579290000110 ) ) ;
#41139=CARTESIAN_POINT ( 'NONE',  ( -0.5337784322849999930, -79.61183811491999052, -1.207245797014000255 ) ) ;
#41141=CARTESIAN_POINT ( 'NONE',  ( -1.168951575717731561, -82.80464656011996283, -0.9568345469043921803 ) ) ;
#41146=CARTESIAN_POINT ( 'NONE',  ( 1.206984821263439533, -81.82940592443240746, -0.3247830993265489186 ) ) ;
#41150=ORIENTED_EDGE ( 'NONE', *, *, #9566, .T. ) ;
#41153=VERTEX_POINT ( 'NONE', #37783 ) ;
#41160=CARTESIAN_POINT ( 'NONE',  ( -1.250000000000000000, -79.00000000000000000, 0.000000000000000000 ) ) ;
#41164=VERTEX_POINT ( 'NONE', #28327 ) ;
#41171=DIRECTION ( 'NONE',  ( 0.000000000000000000, 1.000000000000000000, 0.000000000000000000 ) ) ;
#41175=CARTESIAN_POINT ( 'NONE',  ( -0.7081060581029999801, -80.22830095821998952, -1.286481228505000018 ) ) ;
#41201=PLANE ( 'NONE',  #28768 ) ;
#41217=DIRECTION ( 'NONE',  ( 0.000000000000000000, -1.000000000000000000, 0.000000000000000000 ) ) ;
#41223=AXIS2_PLACEMENT_3D ( 'NONE', #40563, #9563, #22552 ) ;
#41230=CARTESIAN_POINT ( 'NONE',  ( 0.8836238660468611616, -82.78814780667313755, -0.8835844391709938295 ) ) ;
#41231=ORIENTED_EDGE ( 'NONE', *, *, #13476, .T. ) ;
#41257=CARTESIAN_POINT ( 'NONE',  ( -0.6349925544693003632, -78.01682879507401935, 1.107199314832773451 ) ) ;
#41263=CARTESIAN_POINT ( 'NONE',  ( -0.02856026855508699350, -79.72578953835795801, 1.512310964717682449 ) ) ;
#41272=CARTESIAN_POINT ( 'NONE',  ( -1.436129866501999919, -82.17181889680999518, 0.6722556991877999266 ) ) ;
#41299=CARTESIAN_POINT ( 'NONE',  ( -1.144396127583604317, -80.56701752473904321, 0.5034462585138648194 ) ) ;
#41304=CARTESIAN_POINT ( 'NONE',  ( 1.532709587175000054, -78.46086630968000009, 0.08112354839639000781 ) ) ;
#41313=CARTESIAN_POINT ( 'NONE',  ( -1.407839100258019949, -79.32013530975854110, 0.5457514781034552565 ) ) ;
#41320=B_SPLINE_CURVE_WITH_KNOTS ( 'NONE', 3,
 ( #27177, #46103, #36633, #31898, #10359, #50521, #37212, #54651, #945, #14190, #32478, #32187, #4764, #50229, #1229, #28343, #46394, #32769, #49646, #9776, #22765, #36047, #18927, #10074, #50816, #19219, #5919, #40775, #27765, #13609, #23925, #45808, #78, #5342, #368, #18055, #18349, #49941, #27473, #24515, #16239, #28640, #6798, #37797, #47561, #51399, #46979, #34218, #20380, #11241, #42530, #2099, #28934, #20098, #29218, #29785, #29508, #46691, #7089, #11529, #24806, #52253, #24225, #42818, #42242, #15655, #43110, #2670, #25088, #20665, #38373, #19803, #51973, #10953, #38662, #38087, #19505, #6210, #1808, #55520, #41944, #56682, #15946, #1515, #2384, #56110, #33651, #55818, #33935, #11811, #37499, #15372, #6506 ),
 .UNSPECIFIED., .F., .F.,
 ( 4, 2, 2, 2, 1, 1, 1, 2, 2, 2, 2, 2, 1, 1, 1, 2, 2, 2, 2, 2, 1, 1, 1, 2, 2, 2, 2, 2, 1, 1, 1, 2, 2, 2, 2, 2, 1, 1, 2, 2, 2, 2, 2, 1, 1, 2, 2, 2, 2, 1, 1, 1, 2, 2, 2, 4 ),
 ( 0.000000000000000000, 0.06249999999995189959, 0.09374999999992783550, 0.1093749999999160671, 0.1171874999999104328, 0.1210937499999074074, 0.1230468749999059086, 0.1240234374999054229, 0.1249999999999049372, 0.1874999999999221179, 0.2187499999999307221, 0.2343749999999348022, 0.2421874999999368283, 0.2460937499999380496, 0.2480468749999386879, 0.2490234374999390210, 0.2499999999999393818, 0.3124999999999485412, 0.3437499999999534261, 0.3593749999999558686, 0.3671874999999573119, 0.3710937499999578115, 0.3730468749999580336, 0.3740234374999581446, 0.3749999999999582001, 0.4375000000000022204, 0.4687500000000242584, 0.4843750000000353051, 0.4921875000000405787, 0.4960937500000432432, 0.4980468750000443534, 0.4990234375000447420, 0.5000000000000450751, 0.5625000000000640599, 0.5937500000000734968, 0.6093750000000782707, 0.6171875000000806022, 0.6210937500000814904, 0.6230468750000819345, 0.6250000000000823785, 0.6875000000000668354, 0.7187500000000590639, 0.7343750000000549560, 0.7421875000000529576, 0.7460937500000521805, 0.7480468750000518474, 0.7500000000000514033, 0.8125000000000446310, 0.8437500000000413003, 0.8593750000000397460, 0.8671875000000386358, 0.8710937500000378586, 0.8730468750000374145, 0.8750000000000368594, 0.9375000000000184297, 1.000000000000000000 ),
 .UNSPECIFIED. ) ;
#41324=DIRECTION ( 'NONE',  ( 0.000000000000000000, -1.000000000000000000, 0.000000000000000000 ) ) ;
#41332=CARTESIAN_POINT ( 'NONE',  ( 1.204186364734999959, -82.23249872513999037, -0.6131120777826000179 ) ) ;
#41333=CARTESIAN_POINT ( 'NONE',  ( 0.6528909987539758264, -78.76693641361094933, -1.116013679407363401 ) ) ;
#41334=CARTESIAN_POINT ( 'NONE',  ( 0.7681833999686413783, -79.32291666666668561, 0.9995835529977274980 ) ) ;
#41335=CARTESIAN_POINT ( 'NONE',  ( 0.1636246173744642929, -78.86458333333332860, 1.250000000000000888 ) ) ;
#41337=CARTESIAN_POINT ( 'NONE',  ( 0.6304340365998000184, -82.61450768115200560, 1.542015542100000136 ) ) ;
#41364=B_SPLINE_CURVE_WITH_KNOTS ( 'NONE', 3,
 ( #38149, #56171, #20446, #51752, #11302, #47627, #25152, #2733, #11878, #29856, #47911, #41313, #46936, #14724, #55776, #19174, #23590, #51651, #10911, #32722, #10614, #51352, #18879, #5873, #56069, #42488, #1764, #37171, #19462, #28887, #46642, #23306, #6461, #898, #50476, #24474, #23882, #55182, #33608, #15324, #2058, #28009, #20059, #38045, #6170, #41604, #28595, #29178, #51065, #24180, #33017, #1473, #33317, #15613, #11202, #47225, #42195, #36875, #46349, #19758, #1184, #54886, #14436, #32431, #41898, #55477, #50773, #37458, #37755, #15024, #10027, #46056, #5579, #10318, #28296, #21483, #21192, #47519, #20335, #30618, #16487, #7618, #17055, #12053, #48366, #35036, #2341, #39490, #11490, #53071, #57491, #12621, #56927, #7048, #30034, #43348 ),
 .UNSPECIFIED., .F., .F.,
 ( 4, 2, 2, 2, 2, 2, 1, 2, 2, 2, 2, 2, 2, 2, 2, 2, 2, 2, 2, 2, 2, 2, 2, 2, 2, 2, 2, 2, 2, 2, 2, 2, 2, 2, 2, 2, 2, 2, 2, 2, 2, 2, 1, 2, 2, 2, 2, 2, 4 ),
 ( 0.000000000000000000, 0.01562499999999996531, 0.03124999999999993061, 0.04687499999999990979, 0.06249999999999988898, 0.07812499999999986122, 0.09374999999999984734, 0.1093749999999998196, 0.1249999999999998335, 0.1406249999999998335, 0.1562499999999998057, 0.1718749999999998057, 0.1874999999999998057, 0.2031249999999998057, 0.2187499999999997780, 0.2343749999999997780, 0.2499999999999997780, 0.2812499999999998335, 0.3124999999999998335, 0.3437499999999998890, 0.3749999999999999445, 0.4062500000000000000, 0.4375000000000000000, 0.4687500000000000555, 0.5000000000000001110, 0.5312500000000001110, 0.5625000000000002220, 0.5937500000000002220, 0.6250000000000002220, 0.6562500000000003331, 0.6875000000000003331, 0.7187500000000004441, 0.7500000000000004441, 0.7656250000000005551, 0.7812500000000004441, 0.7968750000000004441, 0.8125000000000004441, 0.8281250000000003331, 0.8437500000000003331, 0.8593750000000003331, 0.8750000000000002220, 0.8906250000000002220, 0.9062500000000002220, 0.9218750000000002220, 0.9375000000000001110, 0.9531250000000001110, 0.9687500000000001110, 0.9843750000000000000, 1.000000000000000000 ),
 .UNSPECIFIED. ) ;
#41395=CARTESIAN_POINT ( 'NONE',  ( -1.566959183383000109, -78.24862352424000278, 0.4396611996733000294 ) ) ;
#41416=ORIENTED_EDGE ( 'NONE', *, *, #27992, .T. ) ;
#41432=CARTESIAN_POINT ( 'NONE',  ( -0.4240539849974000464, -80.10665717147000464, 1.611036072322000079 ) ) ;
#41433=CARTESIAN_POINT ( 'NONE',  ( -0.1527015615469000109, -77.84095328623999421, 1.349110360386999830 ) ) ;
#41435=CARTESIAN_POINT ( 'NONE',  ( 0.3510616317362846295, -81.89369634218427052, -1.470620435669331760 ) ) ;
#41437=DIRECTION ( 'NONE',  ( 0.000000000000000000, -1.000000000000000000, -1.767388436867000098E-14 ) ) ;
#41438=CARTESIAN_POINT ( 'NONE',  ( 0.000000000000000000, -86.29999999996098836, 0.000000000000000000 ) ) ;
#41449=ORIENTED_EDGE ( 'NONE', *, *, #20861, .F. ) ;
#41460=CARTESIAN_POINT ( 'NONE',  ( -1.250000000000000000, -78.60000000000000853, 0.000000000000000000 ) ) ;
#41467=CARTESIAN_POINT ( 'NONE',  ( 1.446151133417000079, -79.40723116178999419, 0.2550274018384999786 ) ) ;
#41469=B_SPLINE_CURVE_WITH_KNOTS ( 'NONE', 3,
 ( #18214, #35903, #54223, #36491, #40038, #31759 ),
 .UNSPECIFIED., .F., .F.,
 ( 4, 2, 4 ),
 ( 0.000000000000000000, 0.5000000000000001110, 1.000000000000000000 ),
 .UNSPECIFIED. ) ;
#41523=CARTESIAN_POINT ( 'NONE',  ( 1.249623181998916532, -82.84938247290897095, -0.01959429098678184752 ) ) ;
#41544=CARTESIAN_POINT ( 'NONE',  ( 1.009560447666660865, -82.90050067395594624, 0.7369711323571810357 ) ) ;
#41550=CARTESIAN_POINT ( 'NONE',  ( 1.291106326275375693, -79.64481427576352246, 0.8295474976191916650 ) ) ;
#41555=CARTESIAN_POINT ( 'NONE',  ( 0.1636246173744697330, -80.63541666666665719, -1.249999999999999778 ) ) ;
#41604=CARTESIAN_POINT ( 'NONE',  ( 0.8611387563286860836, -78.67764650869405330, 1.274486801945468262 ) ) ;
#41621=CARTESIAN_POINT ( 'NONE',  ( 0.5113695407423999306, -82.86409087623900405, 1.250788716666000111 ) ) ;
#41629=CARTESIAN_POINT ( 'NONE',  ( -1.074445222347000017, -83.11889217614600511, -0.5709172427956999973 ) ) ;
#41640=CARTESIAN_POINT ( 'NONE',  ( -0.006340012436140875923, -79.22516103717930491, -1.262873609533169628 ) ) ;
#41655=CARTESIAN_POINT ( 'NONE',  ( -0.5543002251722001228, -79.23645473738000078, -1.308779764949999924 ) ) ;
#41679=CIRCLE ( 'NONE', #20817, 3.000000000000000000 ) ;
#41683=CARTESIAN_POINT ( 'NONE',  ( 1.619712389308999967, -79.02816550114999927, 0.1587296492880999887 ) ) ;
#41688=B_SPLINE_CURVE_WITH_KNOTS ( 'NONE', 3,
 ( #47592, #43721, #52285, #3274, #25976, #33967, #16557, #52857, #11842, #16847, #48437, #29823, #12123, #12411, #56995, #7403, #17127, #30109 ),
 .UNSPECIFIED., .F., .F.,
 ( 4, 2, 2, 2, 2, 2, 2, 2, 4 ),
 ( 0.000000000000000000, 0.1250000000000000833, 0.2500000000000001110, 0.3750000000000000000, 0.4999999999999999445, 0.6249999999999998890, 0.7499999999999997780, 0.8749999999999998890, 1.000000000000000000 ),
 .UNSPECIFIED. ) ;
#41720=CARTESIAN_POINT ( 'NONE',  ( -1.387963714323000142, -79.66454266569999731, 0.9213108730841000904 ) ) ;
#41723=CARTESIAN_POINT ( 'NONE',  ( -0.3338606378991729740, -81.35724788051247458, -1.472545958893958673 ) ) ;
#41727=CARTESIAN_POINT ( 'NONE',  ( 1.131032139596482189, -79.81496092797256381, -0.5356056669552815563 ) ) ;
#41728=CARTESIAN_POINT ( 'NONE',  ( 1.249734714957977388, -80.86107366444541356, 0.1638716315211910246 ) ) ;
#41729=ORIENTED_EDGE ( 'NONE', *, *, #45605, .T. ) ;
#41730=CARTESIAN_POINT ( 'NONE',  ( 0.4310498522562998258, -81.75308031528319930, -1.176456706122102069 ) ) ;
#41742=CARTESIAN_POINT ( 'NONE',  ( -1.493489583059197878, -77.75651041671019925, -0.1963495429841721485 ) ) ;
#41797=EDGE_CURVE ( 'NONE', #37205, #27512, #57861, .T. ) ;
#41808=ORIENTED_EDGE ( 'NONE', *, *, #28852, .F. ) ;
#41815=CARTESIAN_POINT ( 'NONE',  ( 1.204475114971339522, -82.82837777568340698, -0.3367243055637897942 ) ) ;
#41819=CARTESIAN_POINT ( 'NONE',  ( -0.2201363562291999698, -79.36327907013999550, -1.483758735329000045 ) ) ;
#41827=AXIS2_PLACEMENT_3D ( 'NONE', #12658, #7941, #26810 ) ;
#41840=CARTESIAN_POINT ( 'NONE',  ( 1.124534988792357471, -82.88598862276096213, 0.5462022235247268043 ) ) ;
#41842=CARTESIAN_POINT ( 'NONE',  ( -1.250652913346715689, -78.08346917523292063, 0.2616640092690510899 ) ) ;
#41898=CARTESIAN_POINT ( 'NONE',  ( 0.9708803083217455443, -78.16900954117737399, 1.156142391821560755 ) ) ;
#41916=CARTESIAN_POINT ( 'NONE',  ( -1.259088972310000054, -82.99040930645999481, 0.4905773767712000577 ) ) ;
#41919=CARTESIAN_POINT ( 'NONE',  ( 1.217465845835393967, -82.77083333333332860, 0.3271848554491025851 ) ) ;
#41944=CARTESIAN_POINT ( 'NONE',  ( 1.068867549261173000, -81.39395485511519723, 0.6488671464486228668 ) ) ;
#41966=EDGE_LOOP ( 'NONE', ( #37711, #30741, #45969 ) ) ;
#41971=CARTESIAN_POINT ( 'NONE',  ( 2.500000000000000000, -80.69999999999998863, 0.000000000000000000 ) ) ;
#41976=CARTESIAN_POINT ( 'NONE',  ( -0.6794254437148999903, -78.86112079180999501, -1.478865823597000029 ) ) ;
#41986=CARTESIAN_POINT ( 'NONE',  ( -1.425428639595999858, -80.85725624887999174, 0.6946581327067000711 ) ) ;
#42016=CARTESIAN_POINT ( 'NONE',  ( -0.7048934085577001074, -80.97905750928998714, -1.509431780672999990 ) ) ;
#42017=CARTESIAN_POINT ( 'NONE',  ( -1.314590664899999872, -77.98943747231999168, -0.5743650807226000632 ) ) ;
#42027=CARTESIAN_POINT ( 'NONE',  ( -0.4710266599135919940, -81.69439008557912985, -1.157763597771598540 ) ) ;
#42049=B_SPLINE_CURVE_WITH_KNOTS ( 'NONE', 3,
 ( #46549, #6075, #55970, #1668, #19658, #15225, #37948, #15521, #26102, #11967, #29658, #48281, #35234, #38820, #16107, #6950 ),
 .UNSPECIFIED., .F., .F.,
 ( 4, 2, 2, 2, 2, 2, 2, 4 ),
 ( 0.000000000000000000, 0.1785697310289149631, 0.2678545965433721809, 0.3571394620578294266, 0.4464243275722866722, 0.5357091930867439178, 0.6249940586012011634, 0.7142789241156584090 ),
 .UNSPECIFIED. ) ;
#42054=CARTESIAN_POINT ( 'NONE',  ( -0.7285569484545000307, -79.65971054856998990, -1.138057995564000002 ) ) ;
#42058=CARTESIAN_POINT ( 'NONE',  ( 0.7142021645403204833, -79.58595579008107279, 1.332894191355008529 ) ) ;
#42074=DIRECTION ( 'NONE',  ( 0.000000000000000000, -1.000000000000000000, 0.000000000000000000 ) ) ;
#42076=CARTESIAN_POINT ( 'NONE',  ( 1.167836049095117623, -78.37932260450160982, 0.4458657978228700025 ) ) ;
#42118=CARTESIAN_POINT ( 'NONE',  ( -1.505451346423154257, -79.24564413794375639, 0.08303611744945066375 ) ) ;
#42119=AXIS2_PLACEMENT_3D ( 'NONE', #21752, #35912, #53344 ) ;
#42136=CARTESIAN_POINT ( 'NONE',  ( 0.2018703831548298022, -82.96236683731123662, 1.233436793893810890 ) ) ;
#42138=CARTESIAN_POINT ( 'NONE',  ( 1.092232985442820992, -80.29166666666665719, 0.6295237254636267821 ) ) ;
#42162=CARTESIAN_POINT ( 'NONE',  ( -0.4492251327744000156, -81.78555210223998984, 1.604198796042999753 ) ) ;
#42173=CARTESIAN_POINT ( 'NONE',  ( 0.007231935760147001867, -80.72610880796425192, -1.249626014905791171 ) ) ;
#42178=ORIENTED_EDGE ( 'NONE', *, *, #44622, .T. ) ;
#42180=CARTESIAN_POINT ( 'NONE',  ( -0.9228900258640634346, -80.54165424860717337, 0.8427052285091912731 ) ) ;
#42191=CARTESIAN_POINT ( 'NONE',  ( -0.5056747962987626632, -80.19197092624497714, -1.143462194401485998 ) ) ;
#42195=CARTESIAN_POINT ( 'NONE',  ( -1.463614972483658683, -78.37424901929817622, -0.4741960517313459356 ) ) ;
#42212=CARTESIAN_POINT ( 'NONE',  ( 1.242145130744999992, -82.73777244601899383, -0.5320213307544999770 ) ) ;
#42224=CARTESIAN_POINT ( 'NONE',  ( 1.213634779058999857, -82.86625531570498993, 0.5941895605367999433 ) ) ;
#42242=CARTESIAN_POINT ( 'NONE',  ( 0.4771002761174171769, -81.44403856892047600, 1.155230721378893044 ) ) ;
#42245=DIRECTION ( 'NONE',  ( 0.000000000000000000, 1.000000000000000000, 0.000000000000000000 ) ) ;
#42249=CARTESIAN_POINT ( 'NONE',  ( -1.405934784949000038, -79.13159159781999108, 0.2091203166687999881 ) ) ;
#42276=CARTESIAN_POINT ( 'NONE',  ( -0.7004323366084000968, -78.41920298766999053, -1.469032877812000093 ) ) ;
#42277=CARTESIAN_POINT ( 'NONE',  ( -1.049212147998610511, -79.14604918627101426, -0.6836784682508713074 ) ) ;
#42289=EDGE_CURVE ( 'NONE', #7824, #14640, #4851, .T. ) ;
#42308=CARTESIAN_POINT ( 'NONE',  ( -0.9465222407332000154, -81.15663953506998496, -0.8164530897714000757 ) ) ;
#42310=CARTESIAN_POINT ( 'NONE',  ( -0.4987175214384371169, -80.00792896450899150, 1.146052696381754110 ) ) ;
#42314=EDGE_CURVE ( 'NONE', #31856, #19957, #46568, .T. ) ;
#42315=CARTESIAN_POINT ( 'NONE',  ( -1.387963714323000142, -79.72375898957000118, 0.9213108730841000904 ) ) ;
#42316=CARTESIAN_POINT ( 'NONE',  ( 1.158746710145999836, -78.15648218165999594, -0.8458044512135999282 ) ) ;
#42318=CARTESIAN_POINT ( 'NONE',  ( 1.105771037839567761, -81.55968126227546122, 1.028509483357399112 ) ) ;
#42319=CARTESIAN_POINT ( 'NONE',  ( -1.464697089188547574, -83.32914288647991441, 0.3814761973796438888 ) ) ;
#42322=CARTESIAN_POINT ( 'NONE',  ( 0.3279140402491176332, -80.95484126934748303, 1.218292940065619057 ) ) ;
#42324=CARTESIAN_POINT ( 'NONE',  ( -0.03659624652677806456, -81.72330189448304338, -1.249620685942105958 ) ) ;
#42327=CARTESIAN_POINT ( 'NONE',  ( -1.217465845835394411, -80.02083333333330017, -0.3271848554491003647 ) ) ;
#42336=LINE ( 'NONE', #1903, #18855 ) ;
#42351=CARTESIAN_POINT ( 'NONE',  ( -1.250000000000001332, -79.98958333333332860, 0.1636246173744632659 ) ) ;
#42353=CARTESIAN_POINT ( 'NONE',  ( 1.554657762476000071, -80.98652648686000077, -0.6948770361563999520 ) ) ;
#42356=CARTESIAN_POINT ( 'NONE',  ( 1.437150570762024460, -79.52522577555218675, 0.4693744638702325722 ) ) ;
#42372=CARTESIAN_POINT ( 'NONE',  ( 0.4847454816353202744, -78.44349313809972557, 1.152238203202561762 ) ) ;
#42399=EDGE_CURVE ( 'NONE', #32925, #50534, #39341, .T. ) ;
#42408=CARTESIAN_POINT ( 'NONE',  ( 0.7483892436387024061, -82.77648090350101029, -1.000966064142216450 ) ) ;
#42413=CARTESIAN_POINT ( 'NONE',  ( -1.339962141614804425, -78.21213723365808335, 0.6906518060847610663 ) ) ;
#42423=CARTESIAN_POINT ( 'NONE',  ( 1.092232985442823212, -81.20833333333332860, -0.6295237254636224522 ) ) ;
#42433=CARTESIAN_POINT ( 'NONE',  ( 0.8790514971010287004, -82.91354635334799639, 0.8881463262467683695 ) ) ;
#42456=CARTESIAN_POINT ( 'NONE',  ( 1.484562552624000054, -82.10134817779000116, -0.7558657512595999828 ) ) ;
#42460=DIRECTION ( 'NONE',  ( 0.000000000000000000, 0.000000000000000000, -1.000000000000000000 ) ) ;
#42473=CARTESIAN_POINT ( 'NONE',  ( -0.3529553161740807132, -80.49780249966943302, 1.199325851874515125 ) ) ;
#42488=CARTESIAN_POINT ( 'NONE',  ( 1.440361722493033625, -79.12381928720844826, 0.4511061928964619772 ) ) ;
#42491=AXIS2_PLACEMENT_3D ( 'NONE', #5348, #663, #18650 ) ;
#42501=CARTESIAN_POINT ( 'NONE',  ( -1.266615395500999997, -82.54829480068799796, -0.4708042714212999913 ) ) ;
#42514=DIRECTION ( 'NONE',  ( 0.000000000000000000, 1.000000000000000000, 0.000000000000000000 ) ) ;
#42530=CARTESIAN_POINT ( 'NONE',  ( -0.007979420377872919676, -81.47602220864618516, 1.249669167965647532 ) ) ;
#42536=CARTESIAN_POINT ( 'NONE',  ( -1.293726968080000095, -79.06827490904998967, 0.1924304001467000147 ) ) ;
#42538=CARTESIAN_POINT ( 'NONE',  ( -0.1636246173744726473, -78.38541666666664298, 1.249999999999999112 ) ) ;
#42564=CARTESIAN_POINT ( 'NONE',  ( 1.621809933883000099, -78.58624769700999479, 0.1356303529659999840 ) ) ;
#42575=VECTOR ( 'NONE', #56421, 1000.000000000000114 ) ;
#42576=CARTESIAN_POINT ( 'NONE',  ( -0.9103895169571000201, -79.40443682768999167, -1.233764334031000054 ) ) ;
#42586=CYLINDRICAL_SURFACE ( 'NONE', #22417, 1.250000000000000000 ) ;
#42603=CARTESIAN_POINT ( 'NONE',  ( -1.157298774452520496, -80.06939412680100077, 0.4720562922803016592 ) ) ;
#42609=DIRECTION ( 'NONE',  ( 0.000000000000000000, -1.000000000000000000, 0.000000000000000000 ) ) ;
#42610=CARTESIAN_POINT ( 'NONE',  ( -1.539734144441496699, -82.35743973534117401, -0.1659400480913056364 ) ) ;
#42611=CARTESIAN_POINT ( 'NONE',  ( -1.151101085867609397, -79.63220894243453074, -0.4868159640311818803 ) ) ;
#42614=CARTESIAN_POINT ( 'NONE',  ( 0.01697733933020722369, -81.72664603025980057, -1.249565628801712291 ) ) ;
#42637=CARTESIAN_POINT ( 'NONE',  ( 1.092232985442820992, -79.79166666666665719, 0.6295237254636267821 ) ) ;
#42639=CARTESIAN_POINT ( 'NONE',  ( -0.7205381521189000438, -80.86020805664000477, -1.542932836074000003 ) ) ;
#42642=ADVANCED_FACE ( 'NONE', ( #34482, #51669 ), #38924, .F. ) ;
#42644=CARTESIAN_POINT ( 'NONE',  ( -0.02850738685234475642, -79.62644246643365875, 1.511250209800697908 ) ) ;
#42657=CARTESIAN_POINT ( 'NONE',  ( -0.001748811790489142098, -78.47533359273272424, 1.249867168124328298 ) ) ;
#42674=CARTESIAN_POINT ( 'NONE',  ( -0.9995835529977249445, -82.55208333333330017, -0.7681833999686439318 ) ) ;
#42676=DIRECTION ( 'NONE',  ( 1.000000000000000000, 0.000000000000000000, 0.000000000000000000 ) ) ;
#42683=CARTESIAN_POINT ( 'NONE',  ( -10.14999999998000035, -87.10000000002298748, 2.878919856867000406E-10 ) ) ;
#42695=CARTESIAN_POINT ( 'NONE',  ( 0.7046260488188935689, -82.77294570575585908, -1.032333493006673653 ) ) ;
#42700=CARTESIAN_POINT ( 'NONE',  ( 0.9175530224387180578, -78.92634932198247100, -1.226298970086918905 ) ) ;
#42707=CARTESIAN_POINT ( 'NONE',  ( 0.7445603198294054037, -81.18334426506562806, 1.317420973437698484 ) ) ;
#42708=VECTOR ( 'NONE', #33595, 1000.000000000000000 ) ;
#42720=CARTESIAN_POINT ( 'NONE',  ( 0.8801428981091761194, -82.91344897987683282, 0.8870736079473547919 ) ) ;
#42733=SURFACE_STYLE_USAGE ( .BOTH. , #47179 ) ;
#42755=CARTESIAN_POINT ( 'NONE',  ( 0.4031446930405725992, -80.75178943763351924, -1.187466692091743159 ) ) ;
#42761=ORIENTED_EDGE ( 'NONE', *, *, #33179, .F. ) ;
#42764=CARTESIAN_POINT ( 'NONE',  ( -0.7013479997696390189, -80.52279179898042116, 1.035593156588225039 ) ) ;
#42791=CARTESIAN_POINT ( 'NONE',  ( 1.465719397218613329, -79.98070088451875392, -0.3642262430507383630 ) ) ;
#42793=CARTESIAN_POINT ( 'NONE',  ( 1.217465845835393967, -79.27083333333330017, 0.3271848554491025851 ) ) ;
#42809=DIRECTION ( 'NONE',  ( -8.423171624505000574E-11, 1.000000000000000000, 1.870145497457000051E-10 ) ) ;
#42813=ORIENTED_EDGE ( 'NONE', *, *, #43305, .F. ) ;
#42818=CARTESIAN_POINT ( 'NONE',  ( 0.4720932691372294321, -81.44439364009578242, 1.157282337904234737 ) ) ;
#42855=CARTESIAN_POINT ( 'NONE',  ( -0.8961266428360998848, -77.81024047417999157, 1.358359200922999888 ) ) ;
#42864=CARTESIAN_POINT ( 'NONE',  ( 0.8470819118255000779, -81.66359336816999814, 1.477252506412999988 ) ) ;
#42865=CARTESIAN_POINT ( 'NONE',  ( -1.563706488702000019, -81.36237249610999811, -0.6734635195847999967 ) ) ;
#42893=CARTESIAN_POINT ( 'NONE',  ( -0.7863337385806483670, -80.02967789379255237, 0.9744850512003893073 ) ) ;
#42899=CARTESIAN_POINT ( 'NONE',  ( 0.5365775619572886734, -82.00317296149017920, -1.414790940926362151 ) ) ;
#42900=CARTESIAN_POINT ( 'NONE',  ( 0.6717993463937350640, -79.77075207433689741, -1.054362998114927619 ) ) ;
#42901=CARTESIAN_POINT ( 'NONE',  ( -1.093352572409234780, -81.05902749701662913, 0.6297817180695111094 ) ) ;
#42909=ORIENTED_EDGE ( 'NONE', *, *, #14581, .T. ) ;
#42916=PRODUCT_CONTEXT ( 'NONE', #11925, 'mechanical' ) ;
#42932=CARTESIAN_POINT ( 'NONE',  ( 0.1636246173744642929, -79.86458333333331439, 1.250000000000000888 ) ) ;
#42934=CARTESIAN_POINT ( 'NONE',  ( -0.5553526962645999321, -81.36548177752000299, -1.429183993495000138 ) ) ;
#42935=CARTESIAN_POINT ( 'NONE',  ( -0.3271848554490991434, -81.10416666666665719, -1.217465845835395299 ) ) ;
#42952=CARTESIAN_POINT ( 'NONE',  ( 0.4131922926977418253, -78.44830526474305543, 1.179719367296339527 ) ) ;
#42954=AXIS2_PLACEMENT_3D ( 'NONE', #52149, #57435, #52433 ) ;
#42965=CARTESIAN_POINT ( 'NONE',  ( -1.613878645371000120, -79.31052490905000241, 0.4035920743843999792 ) ) ;
#42974=CARTESIAN_POINT ( 'NONE',  ( -0.9995835529977281642, -81.94791666666664298, 0.7681833999686391579 ) ) ;
#42980=ORIENTED_EDGE ( 'NONE', *, *, #52535, .T. ) ;
#42987=CARTESIAN_POINT ( 'NONE',  ( 0.8412509418493856472, -82.78432527956375964, -0.9249430534936740056 ) ) ;
#42991=VERTEX_POINT ( 'NONE', #44109 ) ;
#42993=CARTESIAN_POINT ( 'NONE',  ( 1.440783608768007706, -78.47261458352124919, -0.5214944750746852709 ) ) ;
#43014=CARTESIAN_POINT ( 'NONE',  ( 1.249999999999999778, -80.26041666666665719, 0.1636246173744711763 ) ) ;
#43033=CARTESIAN_POINT ( 'NONE',  ( -1.596536837631000072, -81.91187053245998584, -0.4757406268331999533 ) ) ;
#43043=CARTESIAN_POINT ( 'NONE',  ( -1.249670801961172417, -80.60660109082429869, -0.09504704068232089353 ) ) ;
#43050=CARTESIAN_POINT ( 'NONE',  ( -0.2554408763343102851, -80.49153132872807248, 1.223531717389471307 ) ) ;
#43051=B_SPLINE_CURVE_WITH_KNOTS ( 'NONE', 3,
 ( #18577, #874, #36852, #47204, #25024, #24740, #6147, #42755, #37436, #46910, #56616, #11179, #20602, #15591, #19735, #42173, #1450, #29155, #14999, #7021, #38601, #16175, #28276, #43043, #51625 ),
 .UNSPECIFIED., .F., .F.,
 ( 4, 2, 2, 2, 2, 1, 1, 1, 2, 2, 2, 2, 2, 4 ),
 ( 0.000000000000000000, 0.1249999999999988620, 0.2499999999999977240, 0.3749999999999965583, 0.4374999999999960587, 0.4687499999999961142, 0.4843749999999958367, 0.4921874999999953371, 0.4960937499999951150, 0.4999999999999948375, 0.6249999999999961142, 0.7499999999999973355, 0.8749999999999986677, 1.000000000000000000 ),
 .UNSPECIFIED. ) ;
#43054=EDGE_LOOP ( 'NONE', ( #53444, #4090, #26148, #44467 ) ) ;
#43083=ORIENTED_EDGE ( 'NONE', *, *, #32931, .F. ) ;
#43084=CARTESIAN_POINT ( 'NONE',  ( -1.091831352987487014, -80.68921772068907217, 1.043502948795002494 ) ) ;
#43094=CARTESIAN_POINT ( 'NONE',  ( -0.3959877895327999497, -81.54006927205000466, 1.414086365320999850 ) ) ;
#43110=CARTESIAN_POINT ( 'NONE',  ( 0.5742445440065669926, -81.43721952292473532, 1.113553851155867358 ) ) ;
#43125=CARTESIAN_POINT ( 'NONE',  ( 1.419425106214999843, -78.39754962090999868, 0.07512760555724000422 ) ) ;
#43129=B_SPLINE_CURVE_WITH_KNOTS ( 'NONE', 3,
 ( #51484, #29024, #50609, #47063 ),
 .UNSPECIFIED., .F., .F.,
 ( 4, 4 ),
 ( 0.000000000000000000, 1.000000000000000000 ),
 .UNSPECIFIED. ) ;
#43138=ORIENTED_EDGE ( 'NONE', *, *, #49890, .T. ) ;
#43148=CARTESIAN_POINT ( 'NONE',  ( -1.573065832928000063, -78.86819029998999042, 0.4172852021023999991 ) ) ;
#43156=CARTESIAN_POINT ( 'NONE',  ( 1.575652246471999973, -82.61098159482399694, 0.6458614041720999177 ) ) ;
#43157=CARTESIAN_POINT ( 'NONE',  ( 0.2307066564514000107, -79.59422942033999959, -1.449970716867000187 ) ) ;
#43166=CARTESIAN_POINT ( 'NONE',  ( 0.3647771924839282587, -81.24853632404513348, -1.197947852285521142 ) ) ;
#43184=CARTESIAN_POINT ( 'NONE',  ( -1.246072329358421271, -80.09278992987992751, 0.1233981338585028870 ) ) ;
#43192=CARTESIAN_POINT ( 'NONE',  ( -1.356806863440251254, -82.81292558743855636, 0.6692837476566168009 ) ) ;
#43217=CARTESIAN_POINT ( 'NONE',  ( 0.6295237254636211199, -79.83333333333334281, 1.092232985442824322 ) ) ;
#43219=CARTESIAN_POINT ( 'NONE',  ( -0.7646200840319000713, -80.29161764699000514, -1.389155443296000048 ) ) ;
#43222=CARTESIAN_POINT ( 'NONE',  ( -0.4053727578492293815, -79.64668580460995884, 1.457040148635480703 ) ) ;
#43239=CARTESIAN_POINT ( 'NONE',  ( 0.5021253177900999454, -81.91975631494000254, -1.588436081161999969 ) ) ;
#43245=CIRCLE ( 'NONE', #17778, 0.5000000000000004441 ) ;
#43246=DIRECTION ( 'NONE',  ( 0.000000000000000000, -1.000000000000000000, 0.000000000000000000 ) ) ;
#43253=CARTESIAN_POINT ( 'NONE',  ( -0.3694735273699065181, -81.99927641614389984, 1.197870979555107684 ) ) ;
#43254=CARTESIAN_POINT ( 'NONE',  ( 1.657805164101999962, -78.58666450191999786, 0.1386405982960000061 ) ) ;
#43276=CARTESIAN_POINT ( 'NONE',  ( -0.7673595064252045628, -82.67326891823354629, -0.9989183397387743080 ) ) ;
#43280=CARTESIAN_POINT ( 'NONE',  ( -1.455755625768786476, -79.22883914762999780, 0.3955483087397376751 ) ) ;
#43305=EDGE_CURVE ( 'NONE', #32917, #56978, #32650, .T. ) ;
#43334=CARTESIAN_POINT ( 'NONE',  ( -0.2640682808882320876, -80.49207712388174230, 1.221730848296998628 ) ) ;
#43348=CARTESIAN_POINT ( 'NONE',  ( -0.4635254915624000271, -77.75000000000000000, 1.426584774443000025 ) ) ;
#43358=CARTESIAN_POINT ( 'NONE',  ( 1.384776930952473339, -80.53739268436684995, 0.6934519277319081132 ) ) ;
#43369=CARTESIAN_POINT ( 'NONE',  ( 0.6721823118158000154, -81.41359336816999814, 1.172239651246999914 ) ) ;
#43388=CARTESIAN_POINT ( 'NONE',  ( 1.472546342128999930, -80.54088589475999527, -0.7790162248558000213 ) ) ;
#43389=VERTEX_POINT ( 'NONE', #11021 ) ;
#43392=CARTESIAN_POINT ( 'NONE',  ( 0.3277380945383860378, -82.24648727505658030, -1.218584741938794069 ) ) ;
#43395=CARTESIAN_POINT ( 'NONE',  ( -1.217465845835396188, -78.47916666666667140, 0.3271848554490955907 ) ) ;
#43402=ORIENTED_EDGE ( 'NONE', *, *, #22210, .F. ) ;
#43407=CONICAL_SURFACE ( 'NONE', #29237, 10.04999999996000071, 0.7853981633972997312 ) ;
#43437=CARTESIAN_POINT ( 'NONE',  ( -0.5918520097389999846, -82.92677767037399406, -1.596724312065999962 ) ) ;
#43439=CARTESIAN_POINT ( 'NONE',  ( 1.367321113498000118, -81.23636901320000447, 0.5356168500207999505 ) ) ;
#43447=CARTESIAN_POINT ( 'NONE',  ( 0.07980242249672332699, -81.22984433478460176, -1.250509936556952972 ) ) ;
#43456=EDGE_CURVE ( 'NONE', #14640, #22489, #52042, .T. ) ;
#43458=CARTESIAN_POINT ( 'NONE',  ( 1.484562552624000054, -82.04213185391999730, -0.7558657512595999828 ) ) ;
#43470=CARTESIAN_POINT ( 'NONE',  ( -1.155224866089091806, -80.06903521657417855, 0.4771177278498179852 ) ) ;
#43476=CARTESIAN_POINT ( 'NONE',  ( -1.373635873769706306, -82.88377894220877806, -0.6352465044905353242 ) ) ;
#43477=CARTESIAN_POINT ( 'NONE',  ( -1.146293260019806359, -79.63300943463677584, -0.4980201403389062365 ) ) ;
#43499=AXIS2_PLACEMENT_3D ( 'NONE', #31532, #32411, #37145 ) ;
#43506=CARTESIAN_POINT ( 'NONE',  ( 0.9651418585498000580, -79.59702375444000211, 1.402967275931999769 ) ) ;
#43526=AXIS2_PLACEMENT_3D ( 'NONE', #45889, #10156, #14564 ) ;
#43536=CARTESIAN_POINT ( 'NONE',  ( 1.251911631106801481, -81.85749929900767086, 0.1121443075355554597 ) ) ;
#43561=CARTESIAN_POINT ( 'NONE',  ( 0.4026330982763580701, -82.75123106872544554, -1.183384811856946550 ) ) ;
#43565=CARTESIAN_POINT ( 'NONE',  ( 0.4406872078701824513, -79.44681088524180268, 1.169590271965520678 ) ) ;
#43575=CARTESIAN_POINT ( 'NONE',  ( -1.135826688880000157, -81.40663953506998496, -0.9797437077257000748 ) ) ;
#43576=EDGE_CURVE ( 'NONE', #40202, #515, #22093, .T. ) ;
#43585=CARTESIAN_POINT ( 'NONE',  ( 1.153890966263953377, -82.88144626544078619, 0.4805918701253220071 ) ) ;
#43624=CARTESIAN_POINT ( 'NONE',  ( -0.4930276506569527539, -80.50736121252504063, 1.148608259268683041 ) ) ;
#43654=CARTESIAN_POINT ( 'NONE',  ( 0.01012999788566228306, -81.12444949148175510, 1.533525924451510258 ) ) ;
#43665=CARTESIAN_POINT ( 'NONE',  ( -1.329983713389000011, -82.10850220804000799, 0.6225684403671000178 ) ) ;
#43686=B_SPLINE_CURVE_WITH_KNOTS ( 'NONE', 3,
 ( #38810, #6648, #15800, #20236, #56828, #29361, #24944, #11672, #29648, #47699, #25233, #15209, #19645, #43253, #16383, #28486, #33201, #51249, #21378, #48835, #39393, #44695, #4250, #31086, #7523, #16958, #57108, #58271, #16674, #12238, #11955, #8673, #34655, #8377, #34940, #30802, #13089, #22247, #26375, #26662, #21949, #21666, #40258, #30229, #49123, #44394, #52972, #39961, #3946, #35521, #48272, #43837, #57400, #34367, #12803, #3666, #12522, #30519, #48549, #8096, #39672, #52401, #26092, #52683, #57974, #17530, #3385, #7809, #29933, #44117, #53550, #57678, #47986, #25520, #43536, #3100, #21095 ),
 .UNSPECIFIED., .F., .F.,
 ( 4, 2, 2, 1, 1, 2, 2, 2, 2, 2, 2, 2, 2, 2, 2, 2, 1, 1, 2, 2, 2, 2, 2, 2, 2, 2, 1, 2, 2, 2, 2, 2, 1, 1, 1, 2, 2, 2, 1, 1, 1, 2, 2, 4 ),
 ( 0.000000000000000000, 0.1249999999999903411, 0.1874999999999855671, 0.2187499999999831524, 0.2343749999999819034, 0.2421874999999813205, 0.2499999999999807376, 0.3749999999999688582, 0.4374999999999629186, 0.4687499999999600320, 0.4843749999999581446, 0.4999999999999562572, 0.5312499999999524825, 0.5468749999999509281, 0.5624999999999494849, 0.5937499999999463762, 0.6093749999999444888, 0.6171874999999434896, 0.6210937499999430456, 0.6249999999999424904, 0.6562499999999377165, 0.6718749999999353850, 0.6796874999999346079, 0.6874999999999338307, 0.7187499999999299449, 0.7343749999999280575, 0.7421874999999275024, 0.7460937499999268363, 0.7499999999999260591, 0.8124999999999485967, 0.8437499999999600320, 0.8593749999999655831, 0.8671874999999680256, 0.8710937499999695799, 0.8730468749999700240, 0.8740234374999701350, 0.8749999999999701350, 0.9062499999999734657, 0.9218749999999751310, 0.9296874999999763522, 0.9335937499999772404, 0.9355468749999780176, 0.9374999999999786837, 1.000000000000000000 ),
 .UNSPECIFIED. ) ;
#43689=CARTESIAN_POINT ( 'NONE',  ( 0.9441861370063999725, -79.65665688321999482, 1.372505234203999835 ) ) ;
#43695=CARTESIAN_POINT ( 'NONE',  ( -0.9995835529977281642, -78.44791666666662877, 0.7681833999686391579 ) ) ;
#43702=EDGE_CURVE ( 'NONE', #10013, #25387, #51270, .T. ) ;
#43721=CARTESIAN_POINT ( 'NONE',  ( 1.250000000000000222, -83.23958333333330017, -0.1636246173744659582 ) ) ;
#43728=CARTESIAN_POINT ( 'NONE',  ( -1.120375320789137374, -79.13669362328037948, -0.5555032894416228606 ) ) ;
#43735=CARTESIAN_POINT ( 'NONE',  ( 0.7233469165846999616, -82.98993688548499392, -1.541617362406000113 ) ) ;
#43736=CARTESIAN_POINT ( 'NONE',  ( -0.3011984493834000132, -79.78354959200999019, 1.556817658704999996 ) ) ;
#43740=CARTESIAN_POINT ( 'NONE',  ( 1.531359430757999851, -82.42897292706200574, -0.6558942768039000004 ) ) ;
#43762=CARTESIAN_POINT ( 'NONE',  ( 1.197732772806416435, -79.87413707337499602, 0.3747399189747252501 ) ) ;
#43769=CARTESIAN_POINT ( 'NONE',  ( 0.09712307587844953849, -82.47890262923529292, -1.544439509817217893 ) ) ;
#43770=CARTESIAN_POINT ( 'NONE',  ( -0.4052009782446514552, -79.69920052394734000, -1.182528148650172195 ) ) ;
#43804=AXIS2_PLACEMENT_3D ( 'NONE', #15290, #10882, #42460 ) ;
#43805=CARTESIAN_POINT ( 'NONE',  ( -1.250000000000000000, -80.99999999999998579, 0.000000000000000000 ) ) ;
#43837=CARTESIAN_POINT ( 'NONE',  ( 0.8828684872424523711, -81.91318357668050965, 0.8843653071331574189 ) ) ;
#43847=CARTESIAN_POINT ( 'NONE',  ( -1.217465845835396188, -81.97916666666667140, 0.3271848554490955907 ) ) ;
#43864=CARTESIAN_POINT ( 'NONE',  ( -1.376157783432642834, -77.78360998065747367, -0.6179252952255732678 ) ) ;
#43888=DIRECTION ( 'NONE',  ( 1.000000000000000000, 0.000000000000000000, 0.000000000000000000 ) ) ;
#43905=ORIENTED_EDGE ( 'NONE', *, *, #6014, .F. ) ;
#43941=CARTESIAN_POINT ( 'NONE',  ( -0.8698823052784736554, -80.17301259719361894, 1.277977011521524986 ) ) ;
#43951=CARTESIAN_POINT ( 'NONE',  ( -1.486328135279999962, -82.23497811192000029, -0.5524720742449998889 ) ) ;
#43976=DIRECTION ( 'NONE',  ( 0.000000000000000000, -1.000000000000000000, 0.000000000000000000 ) ) ;
#44015=CARTESIAN_POINT ( 'NONE',  ( -0.7976765672644999805, -81.91623022861000436, -1.504502914139000058 ) ) ;
#44016=CARTESIAN_POINT ( 'NONE',  ( -0.6213570041975999825, -81.04689136786998915, -1.330550119908999962 ) ) ;
#44017=CARTESIAN_POINT ( 'NONE',  ( -0.7494329999370912265, -77.79166666666556296, 1.289876867660085802 ) ) ;
#44020=CARTESIAN_POINT ( 'NONE',  ( -0.5790013745696001024, -82.80792821772298851, -1.562055304842999925 ) ) ;
#44034=CARTESIAN_POINT ( 'NONE',  ( 1.541440768196999933, -82.61056478991099539, 0.6318380856084999664 ) ) ;
#44042=CARTESIAN_POINT ( 'NONE',  ( 0.8345252027113252424, -79.91718069607952657, 0.9304729155346801450 ) ) ;
#44051=CARTESIAN_POINT ( 'NONE',  ( -1.011175526638764532, -81.41610230767864209, -1.124394554489388964 ) ) ;
#44077=CARTESIAN_POINT ( 'NONE',  ( 1.136899222205000060, -79.02463074706000157, 1.164526648744999893 ) ) ;
#44109=CARTESIAN_POINT ( 'NONE',  ( 1.250000000000000000, -79.75000000000000000, 0.000000000000000000 ) ) ;
#44117=CARTESIAN_POINT ( 'NONE',  ( 1.217406450052350930, -81.86832592185405133, 0.2837533658167560313 ) ) ;
#44119=CARTESIAN_POINT ( 'NONE',  ( -0.1834469635243000107, -79.61327907013999550, -1.236465612773999911 ) ) ;
#44193=ORIENTED_EDGE ( 'NONE', *, *, #58205, .F. ) ;
#44206=EDGE_LOOP ( 'NONE', ( #715, #11570, #8241, #35554 ) ) ;
#44214=DIRECTION ( 'NONE',  ( 0.000000000000000000, -1.000000000000000000, 0.000000000000000000 ) ) ;
#44220=CARTESIAN_POINT ( 'NONE',  ( 0.3271848554490964789, -83.35416666666665719, 1.217465845835395521 ) ) ;
#44226=CARTESIAN_POINT ( 'NONE',  ( -1.239625787815246127, -79.89786197137119927, -0.8640456112635624963 ) ) ;
#44234=CARTESIAN_POINT ( 'NONE',  ( -0.5103843434498001042, -82.74009435914298649, -1.376937268564000005 ) ) ;
#44242=CONICAL_SURFACE ( 'NONE', #23516, 2.399999999383999771, 0.7853981633972997312 ) ;
#44251=LINE ( 'NONE', #39236, #35598 ) ;
#44257=CARTESIAN_POINT ( 'NONE',  ( 1.250000000000000000, -80.84999999999999432, 0.000000000000000000 ) ) ;
#44270=CARTESIAN_POINT ( 'NONE',  ( 0.008809971122743728150, -80.22610841291549377, -1.249644143390686413 ) ) ;
#44297=CARTESIAN_POINT ( 'NONE',  ( -0.6878774159238000285, -82.04286360614999296, -1.297410027194999982 ) ) ;
#44298=CARTESIAN_POINT ( 'NONE',  ( 0.5308835263170998964, -81.36284491707999678, 1.242631599581000001 ) ) ;
#44323=CARTESIAN_POINT ( 'NONE',  ( 0.5265852960253567527, -79.94056130876022337, 1.134781841323134088 ) ) ;
#44334=ORIENTED_EDGE ( 'NONE', *, *, #14364, .F. ) ;
#44360=CARTESIAN_POINT ( 'NONE',  ( 0.3271848554491016414, -78.14583333333330017, -1.217465845835393967 ) ) ;
#44394=CARTESIAN_POINT ( 'NONE',  ( 0.8296278938361448807, -81.91774775679489551, 0.9347690852748764545 ) ) ;
#44395=CARTESIAN_POINT ( 'NONE',  ( -1.391773598262999956, -79.42952316759999576, -0.6803270823529999900 ) ) ;
#44405=CARTESIAN_POINT ( 'NONE',  ( 1.199037830717708752, -81.82746532552805263, -0.3535722597945603063 ) ) ;
#44409=ORIENTED_EDGE ( 'NONE', *, *, #10969, .F. ) ;
#44429=CARTESIAN_POINT ( 'NONE',  ( -0.1461529444412975054, -77.86763493222619559, -1.524614525945181320 ) ) ;
#44440=CIRCLE ( 'NONE', #39713, 2.299999999999999822 ) ;
#44467=ORIENTED_EDGE ( 'NONE', *, *, #51070, .F. ) ;
#44468=EDGE_CURVE ( 'NONE', #56551, #38752, #57597, .T. ) ;
#44478=VERTEX_POINT ( 'NONE', #9721 ) ;
#44512=CARTESIAN_POINT ( 'NONE',  ( 0.2546825748345945550, -80.21164111392475604, 1.525549965237892769 ) ) ;
#44522=CARTESIAN_POINT ( 'NONE',  ( -0.5667803598935999831, -82.17197637046999148, 1.605794812195000087 ) ) ;
#44524=CARTESIAN_POINT ( 'NONE',  ( -1.250000000000000000, -83.09999999999999432, 0.000000000000000000 ) ) ;
#44530=CIRCLE ( 'NONE', #28517, 2.899999999999999911 ) ;
#44538=DIRECTION ( 'NONE',  ( -1.000000000000000000, 0.000000000000000000, 0.000000000000000000 ) ) ;
#44556=ORIENTED_EDGE ( 'NONE', *, *, #25410, .T. ) ;
#44559=CARTESIAN_POINT ( 'NONE',  ( -0.7298471776477999384, -78.68147770778000449, 1.477907092941999956 ) ) ;
#44562=CARTESIAN_POINT ( 'NONE',  ( -1.505183525871029993, -79.25404663310062858, -0.07739674404991536694 ) ) ;
#44563=CARTESIAN_POINT ( 'NONE',  ( -0.2325945923070667498, -80.21064443203673022, -1.228314969166735215 ) ) ;
#44588=AXIS2_PLACEMENT_3D ( 'NONE', #5878, #55482, #15331 ) ;
#44590=ORIENTED_EDGE ( 'NONE', *, *, #8876, .F. ) ;
#44591=CARTESIAN_POINT ( 'NONE',  ( -1.519651782304000109, -81.91638770227000066, -0.4528301974880000191 ) ) ;
#44592=CARTESIAN_POINT ( 'NONE',  ( -1.273831304311999979, -81.04704884152999966, -0.4509157470602000450 ) ) ;
#44610=CARTESIAN_POINT ( 'NONE',  ( 0.8286895765316001361, -81.60396023938999122, 1.445177540541999983 ) ) ;
#44619=CARTESIAN_POINT ( 'NONE',  ( 0.8492318889338164034, -79.91594626102744314, 0.9170975991313886633 ) ) ;
#44622=EDGE_CURVE ( 'NONE', #32925, #12786, #5287, .T. ) ;
#44632=AXIS2_PLACEMENT_3D ( 'NONE', #40368, #49532, #19399 ) ;
#44644=CARTESIAN_POINT ( 'NONE',  ( -1.218569463821508547, -82.57982710409879701, 0.3278157668757434862 ) ) ;
#44647=CARTESIAN_POINT ( 'NONE',  ( 1.086236247072508654, -79.39183646607358469, 0.6189023910738301604 ) ) ;
#44658=FACE_OUTER_BOUND ( 'NONE', #12438, .T. ) ;
#44678=ORIENTED_EDGE ( 'NONE', *, *, #26975, .T. ) ;
#44690=DIRECTION ( 'NONE',  ( 0.000000000000000000, 1.000000000000000000, 0.000000000000000000 ) ) ;
#44695=CARTESIAN_POINT ( 'NONE',  ( 0.03753981069206074189, -81.97327235835214765, 1.249602265122939704 ) ) ;
#44696=CARTESIAN_POINT ( 'NONE',  ( 0.1360381241691999976, -78.76134433024999737, 1.543111746742000134 ) ) ;
#44703=ORIENTED_EDGE ( 'NONE', *, *, #53175, .T. ) ;
#44704=CARTESIAN_POINT ( 'NONE',  ( 0.8896540882221496416, -81.78862763931634561, -0.8776062606573753477 ) ) ;
#44716=LINE ( 'NONE', #32279, #45194 ) ;
#44736=CARTESIAN_POINT ( 'NONE',  ( -0.4406873220133000202, -81.17553171121998901, -1.134095991600000186 ) ) ;
#44762=ADVANCED_FACE ( 'NONE', ( #55745 ), #10813, .T. ) ;
#44774=ORIENTED_EDGE ( 'NONE', *, *, #13626, .T. ) ;
#44776=CARTESIAN_POINT ( 'NONE',  ( 0.000000000000000000, -76.75499999999999545, 0.000000000000000000 ) ) ;
#44813=CARTESIAN_POINT ( 'NONE',  ( -0.6609564419650209022, -79.93834960266842415, -1.360574577815365949 ) ) ;
#44823=CARTESIAN_POINT ( 'NONE',  ( -0.4591954515747000420, -81.66670264959000747, 1.639803156192000122 ) ) ;
#44829=ADVANCED_FACE ( 'NONE', ( #34147 ), #26171, .T. ) ;
#44859=CARTESIAN_POINT ( 'NONE',  ( -1.301250031112000105, -78.25114003055999490, -0.8139582694945000085 ) ) ;
#44863=CARTESIAN_POINT ( 'NONE',  ( 1.203234187881469852, -80.32853980534089544, -0.3383792636773915730 ) ) ;
#44887=DIRECTION ( 'NONE',  ( 0.000000000000000000, -1.000000000000000000, 0.000000000000000000 ) ) ;
#44890=CARTESIAN_POINT ( 'NONE',  ( 0.3767945000176999848, -81.53743241160998423, -1.540381938526000027 ) ) ;
#44891=CARTESIAN_POINT ( 'NONE',  ( 0.3870708775265000456, -80.66809355086999744, -1.294661097694999929 ) ) ;
#44932=VERTEX_POINT ( 'NONE', #36775 ) ;
#44975=CARTESIAN_POINT ( 'NONE',  ( -9.500000000000000000, -91.89999999999999147, 7.261899921535998111E-14 ) ) ;
#44990=CARTESIAN_POINT ( 'NONE',  ( 0.6544915521845998674, -81.05404539811999598, 1.531959166345999934 ) ) ;
#44991=CARTESIAN_POINT ( 'NONE',  ( -1.595231864207000028, -77.80712252499999693, 0.4722078832578999741 ) ) ;
#44993=CARTESIAN_POINT ( 'NONE',  ( 0.09701925739682260019, -82.37953645841547257, -1.543345753052644875 ) ) ;
#45000=CARTESIAN_POINT ( 'NONE',  ( 1.158141336542465760, -81.81941502368277952, -0.4701679534010050343 ) ) ;
#45003=DIRECTION ( 'NONE',  ( 0.000000000000000000, -1.000000000000000000, 0.000000000000000000 ) ) ;
#45012=DIRECTION ( 'NONE',  ( 0.000000000000000000, 1.000000000000000000, 1.567738888216000128E-14 ) ) ;
#45035=CARTESIAN_POINT ( 'NONE',  ( 0.6120151737828000149, -80.41762112988999434, 1.204744225600999918 ) ) ;
#45037=CARTESIAN_POINT ( 'NONE',  ( -0.7482985437745418578, -79.17427425103403493, -1.003727883348249472 ) ) ;
#45048=ADVANCED_FACE ( 'NONE', ( #57114 ), #12244, .F. ) ;
#45072=ORIENTED_EDGE ( 'NONE', *, *, #52097, .T. ) ;
#45098=EDGE_CURVE ( 'NONE', #16529, #19092, #7528, .T. ) ;
#45109=CARTESIAN_POINT ( 'NONE',  ( 0.9519702974794926886, -79.69303294589165887, -0.8296275306155781459 ) ) ;
#45120=CARTESIAN_POINT ( 'NONE',  ( 0.3139938800012240794, -80.99102801640374594, -1.479408638137562182 ) ) ;
#45163=CARTESIAN_POINT ( 'NONE',  ( 1.514178452211000225, -78.05229887042999337, 0.6512674748728999319 ) ) ;
#45166=CARTESIAN_POINT ( 'NONE',  ( 0.4581446724472641452, -80.25495920898164570, -1.163148308167606171 ) ) ;
#45175=EDGE_CURVE ( 'NONE', #57178, #31856, #36283, .T. ) ;
#45187=EDGE_CURVE ( 'NONE', #44478, #19275, #38235, .T. ) ;
#45189=CARTESIAN_POINT ( 'NONE',  ( 1.495758047513000122, -83.11641278936299670, -0.5264119980271999566 ) ) ;
#45194=VECTOR ( 'NONE', #45012, 1000.000000000000000 ) ;
#45219=CARTESIAN_POINT ( 'NONE',  ( -0.4802501944169854653, -81.75012526588245976, 1.435307468129154440 ) ) ;
#45237=CARTESIAN_POINT ( 'NONE',  ( -1.250000000000000000, -82.59999999999999432, 0.000000000000000000 ) ) ;
#45251=CARTESIAN_POINT ( 'NONE',  ( -1.566959183383000109, -78.18940720036999892, 0.4396611996733000294 ) ) ;
#45254=CARTESIAN_POINT ( 'NONE',  ( 1.217465845835394855, -78.22916666666665719, -0.3271848554490981997 ) ) ;
#45291=CARTESIAN_POINT ( 'NONE',  ( 0.4771943503223999850, -80.35929403190999665, -1.596102929133000004 ) ) ;
#45292=CARTESIAN_POINT ( 'NONE',  ( -0.6467060841615001054, -78.98407060936000335, -1.407647497788000024 ) ) ;
#45304=CARTESIAN_POINT ( 'NONE',  ( 1.250000000000000222, -80.23958333333330017, -0.1636246173744659582 ) ) ;
#45309=ORIENTED_EDGE ( 'NONE', *, *, #53583, .F. ) ;
#45330=CARTESIAN_POINT ( 'NONE',  ( 0.3004848064042999756, -79.72286976367999500, -1.317452118262000038 ) ) ;
#45372=VERTEX_POINT ( 'NONE', #48841 ) ;
#45389=CARTESIAN_POINT ( 'NONE',  ( 1.157512255224546038, -82.81922399004812974, -0.4718293121365144671 ) ) ;
#45414=CARTESIAN_POINT ( 'NONE',  ( -1.464549325067485253, -80.86956512251046547, -0.3794217626884464623 ) ) ;
#45416=CARTESIAN_POINT ( 'NONE',  ( -1.140226658635634216, -81.53775969004665569, -0.5918896188631093125 ) ) ;
#45418=CARTESIAN_POINT ( 'NONE',  ( 1.217465845835394855, -80.72916666666665719, -0.3271848554490981997 ) ) ;
#45423=CARTESIAN_POINT ( 'NONE',  ( 1.565347158977999920, -82.48777244601899383, -0.6704515100525999527 ) ) ;
#45457=CARTESIAN_POINT ( 'NONE',  ( 1.261551586316999707, -78.40843473990000234, -0.8742238293381999759 ) ) ;
#45461=CARTESIAN_POINT ( 'NONE',  ( 0.9060466714856187931, -80.29006661044611803, -0.8607755742940681465 ) ) ;
#45481=CARTESIAN_POINT ( 'NONE',  ( -1.331776743724000234, -83.47447248197899228, -0.3115240295706999674 ) ) ;
#45482=CARTESIAN_POINT ( 'NONE',  ( -0.9994823880747228939, -78.65231536704800419, -0.7681904385035477345 ) ) ;
#45483=CARTESIAN_POINT ( 'NONE',  ( -0.7681833999686477066, -79.42708333333332860, 0.9995835529977223910 ) ) ;
#45510=AXIS2_PLACEMENT_3D ( 'NONE', #29195, #34192, #7920 ) ;
#45547=CARTESIAN_POINT ( 'NONE',  ( 0.1198033158700999995, -79.19874496458000124, 1.623056241665000066 ) ) ;
#45584=B_SPLINE_SURFACE_WITH_KNOTS ( 'NONE', 3, 3, ( 
 ( #47274, #1813, #11245, #6215, #42536, #29224, #50525, #33656, #46106, #19223, #10668, #33069, #51114, #1234, #24230, #55525, #15072, #33368, #10079, #28646, #46696, #37215, #10958, #24521, #949, #10363, #28350, #28060, #37803, #23930, #2103, #55228, #5630, #56114, #6803 ),
 ( #23642, #51697, #41655, #14775, #42249, #19810, #55823, #46398, #20102, #38093, #24811, #18934, #23146, #8992, #16255, #34233, #21247, #30670, #43125, #47576, #39250, #38966, #30090, #29800, #16540, #34520, #57265, #12393, #52552, #12107, #30383, #7962, #21538, #39543, #17109 ),
 ( #12678, #8250, #26252, #23296, #50177, #9138, #27423, #12958, #27123, #35690, #31247, #30954, #27711, #31845, #32136, #5288, #4713, #9722, #41304, #45457, #45755, #41015, #44859, #40724, #889, #49289, #18873, #9433, #13554, #40122, #18294, #8840, #607, #18, #4999 ),
 ( #53409, #22113, #18587, #35988, #26830, #48993, #23004, #8539, #17997, #13255, #36577, #54600, #4411, #54013, #26532, #44559, #4112, #58135, #49887, #36288, #17701, #14137, #53717, #22414, #40427, #31546, #49592, #45163, #22711, #316, #54310, #13848, #37450, #10605, #10312 ) ),
 .UNSPECIFIED., .F., .F., .F.,
 ( 4, 4 ),
 ( 4, 1, 1, 1, 1, 1, 1, 1, 1, 1, 1, 1, 1, 1, 1, 1, 1, 1, 1, 1, 1, 1, 1, 1, 1, 1, 1, 1, 1, 1, 1, 1, 4 ),
 ( -0.1331668876848000060, 1.133166887685000068 ),
 ( -0.01660298332971000060, 0.01037686458107000068, 0.03735671249184999848, 0.06433656040262999976, 0.09131640831340999409, 0.1182962562242000082, 0.1452761041350000004, 0.1722559520456999893, 0.1992357999565000093, 0.2262156478673000015, 0.2531954957780999660, 0.2801753436889000137, 0.3071551915995999749, 0.3341350395104000226, 0.3611148874212000148, 0.3880947353320000071, 0.4150745832427999993, 0.4420544311535000159, 0.4690342790643000082, 0.4960141269751000004, 0.5229939748859000481, 0.5499738227967000403, 0.5769536707074000015, 0.6039335186181999937, 0.6309133665289999859, 0.6578932144397999782, 0.6848730623505999704, 0.7118529102612999315, 0.7388327581721000348, 0.7658126060829000270, 0.7927924539937000192, 0.8197723019045000115, 0.8467521498151999726 ),
 .UNSPECIFIED. ) ;
#45587=CARTESIAN_POINT ( 'NONE',  ( 1.551146335801999898, -81.05010250687999473, 0.6076261867840000441 ) ) ;
#45588=CARTESIAN_POINT ( 'NONE',  ( 0.3327358950964000028, -78.66525142865999953, -1.277483743371999880 ) ) ;
#45590=CARTESIAN_POINT ( 'NONE',  ( -0.4470518900855922073, -83.14878330911811588, 1.443941350861193129 ) ) ;
#45605=EDGE_CURVE ( 'NONE', #7477, #35380, #7520, .T. ) ;
#45626=CARTESIAN_POINT ( 'NONE',  ( 1.149971879181999945, -79.78602897879000011, -0.7096026395132000175 ) ) ;
#45639=CARTESIAN_POINT ( 'NONE',  ( -0.9995835529977249445, -79.05208333333331439, -0.7681833999686439318 ) ) ;
#45641=VERTEX_POINT ( 'NONE', #13022 ) ;
#45672=B_SPLINE_CURVE_WITH_KNOTS ( 'NONE', 3,
 ( #15008, #27415, #55166, #5566, #23575, #45747, #51049, #10596, #4992, #5282, #23289, #41009, #50759, #36860, #28581, #41299, #32130, #46625, #19744, #19158, #6155, #24163, #14709, #32707, #42180, #37738, #47502, #56051, #20608, #33875, #51914, #29732, #46917, #42764, #6444, #24461, #11475, #16469, #28872, #43624, #29445, #33594, #20321, #20887, #34161, #42473, #56913, #47783, #43334, #43050, #7029, #38609, #25031, #52198, #2612, #2041, #2325, #2891, #24748, #38892, #33300, #56622, #29163, #25318, #3188, #16183, #11753, #30020, #34451, #7314, #15307, #52483, #56337, #12040, #51633, #48075, #7603, #55761, #47210, #6739, #51337, #21176, #25603, #10896, #20042, #38030, #15600, #11186, #38317, #15890, #14282, #25890, #58291, #49744, #13702, #31697, #39475, #4862, #18147, #36145, #13993, #34739, #30310, #9285, #39179 ),
 .UNSPECIFIED., .F., .F.,
 ( 4, 2, 2, 2, 2, 1, 1, 2, 2, 2, 2, 2, 2, 2, 1, 2, 2, 2, 2, 2, 1, 1, 1, 2, 2, 2, 1, 1, 1, 2, 2, 2, 2, 2, 2, 2, 2, 2, 1, 1, 2, 2, 2, 1, 1, 1, 2, 2, 2, 2, 2, 2, 2, 2, 1, 1, 1, 2, 2, 2, 4 ),
 ( 0.000000000000000000, 0.03124999999997688654, 0.04687499999996567329, 0.06249999999995446698, 0.09374999999993136046, 0.1093749999999194672, 0.1171874999999131528, 0.1210937499999096278, 0.1249999999999061029, 0.1562499999998830935, 0.1718749999998716582, 0.1874999999998602229, 0.2187499999998378242, 0.2343749999998269717, 0.2421874999998215316, 0.2460937499998188116, 0.2499999999998160916, 0.3124999999997497557, 0.3437499999997168376, 0.3593749999997004063, 0.3671874999996924127, 0.3710937499996884159, 0.3730468749996864175, 0.3740234374996853628, 0.3749999999996843081, 0.4062499999996578848, 0.4218749999996443956, 0.4296874999996373456, 0.4335937499996337929, 0.4355468749996320166, 0.4374999999996302402, 0.4687499999996005973, 0.4843749999995854982, 0.4921874999995774491, 0.4999999999995694000, 0.5624999999995077271, 0.5937499999994767519, 0.6093749999994613198, 0.6171874999994536592, 0.6210937499994495514, 0.6230468749994475530, 0.6249999999994455546, 0.6562499999994138022, 0.6718749999993975930, 0.6796874999993898214, 0.6835937499993859356, 0.6855468749993842703, 0.6874999999993826050, 0.7187499999993595123, 0.7343749999993479660, 0.7499999999993364197, 0.8124999999992913446, 0.8437499999992684740, 0.8593749999992571498, 0.8671874999992511546, 0.8710937499992481570, 0.8730468749992466027, 0.8740234374992456035, 0.8749999999992447153, 0.9374999999996223021, 1.000000000000000000 ),
 .UNSPECIFIED. ) ;
#45681=CARTESIAN_POINT ( 'NONE',  ( 0.8852892051488824299, -82.78829553564608545, -0.8819059964711186694 ) ) ;
#45691=DIRECTION ( 'NONE',  ( 1.000000000000000000, 0.000000000000000000, 0.000000000000000000 ) ) ;
#45709=CARTESIAN_POINT ( 'NONE',  ( 1.249999999999999778, -80.76041666666665719, 0.1636246173744711763 ) ) ;
#45713=CARTESIAN_POINT ( 'NONE',  ( 1.508371072044173422, -79.59420473664194162, -0.09860998784024260777 ) ) ;
#45721=CARTESIAN_POINT ( 'NONE',  ( -1.544355253863999966, -83.28778917074799892, -0.3612495668209000366 ) ) ;
#45747=CARTESIAN_POINT ( 'NONE',  ( -1.233649858953178802, -80.58776855326779298, 0.2004323432050792997 ) ) ;
#45755=CARTESIAN_POINT ( 'NONE',  ( 0.4622620975400000276, -78.35600317011999039, -1.463589239453999991 ) ) ;
#45780=CARTESIAN_POINT ( 'NONE',  ( -1.259718275736121162, -81.29651786598202534, -0.8346564987574691674 ) ) ;
#45784=CARTESIAN_POINT ( 'NONE',  ( 0.6295237254636211199, -79.33333333333332860, 1.092232985442824322 ) ) ;
#45785=CARTESIAN_POINT ( 'NONE',  ( 0.9995835529977233902, -82.80208333333331439, 0.7681833999686461523 ) ) ;
#45792=EDGE_LOOP ( 'NONE', ( #33332, #30010 ) ) ;
#45808=CARTESIAN_POINT ( 'NONE',  ( -0.5949523839205194120, -81.51488924677137504, 1.099213967298130923 ) ) ;
#45841=CARTESIAN_POINT ( 'NONE',  ( 0.1660104325307999729, -78.13726038467999047, 1.618982269915999916 ) ) ;
#45849=ORIENTED_EDGE ( 'NONE', *, *, #42289, .F. ) ;
#45880=CARTESIAN_POINT ( 'NONE',  ( 1.587978134902999994, -80.48561246212999265, 0.5035716945827000135 ) ) ;
#45881=CARTESIAN_POINT ( 'NONE',  ( 1.016693945846000036, -78.76897944923000239, 1.012133007862000111 ) ) ;
#45883=CARTESIAN_POINT ( 'NONE',  ( -0.7630392650730208892, -81.83296632765541290, -1.305528064125151655 ) ) ;
#45888=CARTESIAN_POINT ( 'NONE',  ( -1.227645687060430424, -81.61625190046059686, -0.2506207581016212105 ) ) ;
#45889=CARTESIAN_POINT ( 'NONE',  ( 0.000000000000000000, 0.000000000000000000, 0.000000000000000000 ) ) ;
#45893=ORIENTED_EDGE ( 'NONE', *, *, #11738, .F. ) ;
#45909=CARTESIAN_POINT ( 'NONE',  ( -0.3271848554491046945, -81.39583333333327175, 1.217465845835393301 ) ) ;
#45917=CARTESIAN_POINT ( 'NONE',  ( 0.4206423954835999401, -80.29146017332999463, -1.406949933701999944 ) ) ;
#45932=CARTESIAN_POINT ( 'NONE',  ( 0.1636246173744697330, -79.13541666666665719, -1.249999999999999778 ) ) ;
#45952=CARTESIAN_POINT ( 'NONE',  ( -0.7681833999686432657, -82.57291666666667140, -0.9995835529977258327 ) ) ;
#45969=ORIENTED_EDGE ( 'NONE', *, *, #9490, .T. ) ;
#45972=EDGE_LOOP ( 'NONE', ( #53709, #37731 ) ) ;
#45973=ADVANCED_FACE ( 'NONE', ( #4563 ), #1421, .F. ) ;
#45997=CARTESIAN_POINT ( 'NONE',  ( -1.181971670502384386, -83.07366182756899775, 0.4080206837518099428 ) ) ;
#46004=CARTESIAN_POINT ( 'NONE',  ( 1.438147912481374968, -79.62457046011485318, 0.4697345871869623712 ) ) ;
#46051=CARTESIAN_POINT ( 'NONE',  ( -1.153438870374268843, -80.13165335068218553, -0.4814466031038698302 ) ) ;
#46056=CARTESIAN_POINT ( 'NONE',  ( 1.461966789315192861, -78.07977498547253958, -0.3730248769685299282 ) ) ;
#46058=ORIENTED_EDGE ( 'NONE', *, *, #26674, .F. ) ;
#46073=CARTESIAN_POINT ( 'NONE',  ( -1.135826688880000157, -81.30663953507000485, -0.9797437077257000748 ) ) ;
#46075=CARTESIAN_POINT ( 'NONE',  ( -2.299999999999999822, -77.50000000000000000, 0.000000000000000000 ) ) ;
#46086=CARTESIAN_POINT ( 'NONE',  ( -0.2201363562291999698, -79.36327907013999550, -1.483758735329000045 ) ) ;
#46103=CARTESIAN_POINT ( 'NONE',  ( -1.249625625013177643, -81.59763177894343755, 0.04702936436425671218 ) ) ;
#46106=CARTESIAN_POINT ( 'NONE',  ( 1.224841740086000108, -78.85854862992999870, 0.4588522236800000043 ) ) ;
#46120=EDGE_CURVE ( 'NONE', #54581, #34281, #23464, .T. ) ;
#46126=EDGE_CURVE ( 'NONE', #8817, #1475, #50060, .T. ) ;
#46137=CARTESIAN_POINT ( 'NONE',  ( -0.9156221410628999635, -78.13372563058999276, 1.345473579290000110 ) ) ;
#46173=CARTESIAN_POINT ( 'NONE',  ( -1.603789611582999930, -80.23297560169000064, -0.4506860216877000558 ) ) ;
#46174=CARTESIAN_POINT ( 'NONE',  ( 1.066267001953999927, -78.21979887042999735, -0.7783007006953001072 ) ) ;
#46176=CARTESIAN_POINT ( 'NONE',  ( 0.04619448413486952620, -81.37749121868887414, -1.509966902698022251 ) ) ;
#46178=CARTESIAN_POINT ( 'NONE',  ( -1.500128069024530220, -83.33926479430419931, 0.1908857210655489633 ) ) ;
#46184=CARTESIAN_POINT ( 'NONE',  ( -0.4655645666672672545, -81.69477528390797261, -1.159972523025642799 ) ) ;
#46186=( NAMED_UNIT ( * ) PLANE_ANGLE_UNIT ( ) SI_UNIT ( $, .RADIAN. ) );
#46188=FACE_OUTER_BOUND ( 'NONE', #56050, .T. ) ;
#46191=EDGE_CURVE ( 'NONE', #3682, #56978, #33181, .T. ) ;
#46203=VERTEX_POINT ( 'NONE', #38496 ) ;
#46205=DIRECTION ( 'NONE',  ( 0.7071067811865975328, -0.7071067811864976127, -2.062935344748993860E-09 ) ) ;
#46212=CARTESIAN_POINT ( 'NONE',  ( 1.340661125304000167, -80.85989310931999796, -0.5992281077721001159 ) ) ;
#46245=CARTESIAN_POINT ( 'NONE',  ( 0.7681833999686451531, -82.67708333333334281, -0.9995835529977240563 ) ) ;
#46261=ORIENTED_EDGE ( 'NONE', *, *, #20636, .F. ) ;
#46265=ORIENTED_EDGE ( 'NONE', *, *, #46120, .T. ) ;
#46269=CARTESIAN_POINT ( 'NONE',  ( 1.250000000000000000, -82.84999999999999432, 0.000000000000000000 ) ) ;
#46275=CARTESIAN_POINT ( 'NONE',  ( 0.000000000000000000, -77.70312499986998489, -1.546875000130000011 ) ) ;
#46279=CARTESIAN_POINT ( 'NONE',  ( 1.217465845835394855, -81.22916666666665719, -0.3271848554490981997 ) ) ;
#46289=CARTESIAN_POINT ( 'NONE',  ( 0.8221611544660735182, -82.91846127699133717, 0.9412421169495641671 ) ) ;
#46291=CARTESIAN_POINT ( 'NONE',  ( 0.000000000000000000, -76.75499999999999545, 0.000000000000000000 ) ) ;
#46295=CARTESIAN_POINT ( 'NONE',  ( 0.000000000000000000, -76.75499999999999545, 0.000000000000000000 ) ) ;
#46301=CARTESIAN_POINT ( 'NONE',  ( -0.9995835529977249445, -80.55208333333331439, -0.7681833999686439318 ) ) ;
#46314=FACE_OUTER_BOUND ( 'NONE', #6745, .T. ) ;
#46316=CARTESIAN_POINT ( 'NONE',  ( 1.496210884224999926, -83.17505483466200644, 0.7325374182646999799 ) ) ;
#46345=CARTESIAN_POINT ( 'NONE',  ( -1.110657947776001686, -80.13830072341400523, -0.5734848811478387987 ) ) ;
#46349=CARTESIAN_POINT ( 'NONE',  ( -1.440089456762498221, -78.32070828587532674, 0.5413449664772868042 ) ) ;
#46353=FACE_OUTER_BOUND ( 'NONE', #39629, .T. ) ;
#46355=CARTESIAN_POINT ( 'NONE',  ( 0.000000000000000000, -80.79999999999999716, 0.000000000000000000 ) ) ;
#46375=EDGE_LOOP ( 'NONE', ( #20481, #2754, #4329, #34026 ) ) ;
#46382=CARTESIAN_POINT ( 'NONE',  ( -0.1834469635243000107, -79.21327907014000402, -1.236465612773999911 ) ) ;
#46387=ORIENTED_EDGE ( 'NONE', *, *, #20043, .T. ) ;
#46394=CARTESIAN_POINT ( 'NONE',  ( -1.059991318881813527, -81.55564210288132188, 0.6642688495852149266 ) ) ;
#46398=CARTESIAN_POINT ( 'NONE',  ( 0.7471696327285000105, -78.97429688847999785, 1.209193494017000159 ) ) ;
#46408=CARTESIAN_POINT ( 'NONE',  ( 0.000000000000000000, -80.79999999999999716, 0.000000000000000000 ) ) ;
#46425=CARTESIAN_POINT ( 'NONE',  ( 1.328072050606999843, -78.41213347948999512, -0.9406846882429998891 ) ) ;
#46435=CARTESIAN_POINT ( 'NONE',  ( 1.623222485893000000, -80.60446191477998923, 0.5147482071316000773 ) ) ;
#46464=CARTESIAN_POINT ( 'NONE',  ( -1.542698325316999908, -81.35801279995000357, 0.6290719308543000210 ) ) ;
#46465=CARTESIAN_POINT ( 'NONE',  ( -0.6174246106352999641, -78.54625317011999641, -1.294938861597000113 ) ) ;
#46470=ORIENTED_EDGE ( 'NONE', *, *, #11831, .F. ) ;
#46474=ORIENTED_EDGE ( 'NONE', *, *, #32990, .F. ) ;
#46475=CARTESIAN_POINT ( 'NONE',  ( 0.2646997931788037661, -81.74224111115465519, -1.223373072239541726 ) ) ;
#46505=CARTESIAN_POINT ( 'NONE',  ( 1.330733645151999989, -79.34391447301999278, 0.2346736355698000043 ) ) ;
#46509=CARTESIAN_POINT ( 'NONE',  ( -1.510398065887423646, -79.74790249549140242, 0.03865242478268100107 ) ) ;
#46518=DIRECTION ( 'NONE',  ( 1.000000000000000000, 0.000000000000000000, 0.000000000000000000 ) ) ;
#46519=CARTESIAN_POINT ( 'NONE',  ( 0.9995835529977264988, -79.19791666666664298, -0.7681833999686417114 ) ) ;
#46520=ORIENTED_EDGE ( 'NONE', *, *, #54755, .T. ) ;
#46533=DIRECTION ( 'NONE',  ( 0.000000000000000000, -1.000000000000000000, 0.000000000000000000 ) ) ;
#46538=CARTESIAN_POINT ( 'NONE',  ( -1.250000000000000000, -81.09999999999999432, 0.000000000000000000 ) ) ;
#46549=CARTESIAN_POINT ( 'NONE',  ( 1.250000000000000000, -78.35000000000000853, 0.000000000000000000 ) ) ;
#46562=CARTESIAN_POINT ( 'NONE',  ( 1.170361114333020813, -82.82144115138102336, -0.4391466590958141292 ) ) ;
#46566=CARTESIAN_POINT ( 'NONE',  ( -0.6802376739418862783, -78.33817466101120885, -1.374165118460863866 ) ) ;
#46568=CIRCLE ( 'NONE', #48440, 2.500000000000000000 ) ;
#46582=CARTESIAN_POINT ( 'NONE',  ( 0.000000000000000000, -76.75499999999999545, 0.000000000000000000 ) ) ;
#46584=CARTESIAN_POINT ( 'NONE',  ( 0.4742823758087600372, -82.94408184949666918, 1.156490669114161207 ) ) ;
#46625=CARTESIAN_POINT ( 'NONE',  ( -1.102620915002880730, -80.56095890462103171, 0.5891712059213058961 ) ) ;
#46637=CARTESIAN_POINT ( 'NONE',  ( -0.7681743634654464303, -80.17267673354702140, -0.9864499039395765445 ) ) ;
#46642=CARTESIAN_POINT ( 'NONE',  ( 1.252773319961611787, -79.05243164265034750, -0.8433518312087610047 ) ) ;
#46656=CARTESIAN_POINT ( 'NONE',  ( -0.7107282322889000303, -81.60090657403999614, -1.148979047684000054 ) ) ;
#46659=CARTESIAN_POINT ( 'NONE',  ( -1.217465845835396188, -79.47916666666668561, 0.3271848554490955907 ) ) ;
#46666=CARTESIAN_POINT ( 'NONE',  ( -1.259088972310000054, -82.55045924015399805, 0.4905773767712000577 ) ) ;
#46674=B_SPLINE_CURVE_WITH_KNOTS ( 'NONE', 3,
 ( #50916, #19323, #10465, #9883, #33167, #51211, #54468, #45909, #5443, #50044, #10764, #37024, #46793, #23449, #9591, #6317, #20690, #24333 ),
 .UNSPECIFIED., .F., .F.,
 ( 4, 2, 2, 2, 2, 2, 2, 2, 4 ),
 ( 0.000000000000000000, 0.1249999999999999722, 0.2500000000000000000, 0.3750000000000000000, 0.5000000000000001110, 0.6250000000000001110, 0.7500000000000000000, 0.8750000000000000000, 1.000000000000000000 ),
 .UNSPECIFIED. ) ;
#46677=AXIS2_PLACEMENT_3D ( 'NONE', #51853, #11408, #11124 ) ;
#46679=CARTESIAN_POINT ( 'NONE',  ( -0.5979264001123455463, -79.18538552819090626, -1.097664844063911183 ) ) ;
#46691=CARTESIAN_POINT ( 'NONE',  ( 0.3573905483915326697, -81.45234743160045809, 1.197690458606871733 ) ) ;
#46696=CARTESIAN_POINT ( 'NONE',  ( 0.3939293589371000159, -78.22936979258000179, -1.247237820087999882 ) ) ;
#46711=DIRECTION ( 'NONE',  ( -1.000000000000000000, 0.000000000000000000, 0.000000000000000000 ) ) ;
#46720=AXIS2_PLACEMENT_3D ( 'NONE', #33084, #5362, #46711 ) ;
#46727=CARTESIAN_POINT ( 'NONE',  ( 1.314530797355000225, -78.08864832307999393, -0.9595159925157999981 ) ) ;
#46764=CARTESIAN_POINT ( 'NONE',  ( 0.7545134501129999727, -80.66720432497999127, 1.485250302772000097 ) ) ;
#46765=CARTESIAN_POINT ( 'NONE',  ( -1.306286088552999880, -78.49057160033999025, -0.5930400157040000009 ) ) ;
#46767=CARTESIAN_POINT ( 'NONE',  ( -1.416309796911555674, -81.72162796768579085, 0.5272991973399487886 ) ) ;
#46774=CARTESIAN_POINT ( 'NONE',  ( -1.125627005581746554, -81.63605386171199996, -0.5432748768604414025 ) ) ;
#46791=CARTESIAN_POINT ( 'NONE',  ( -3.000000000000000000, -80.79999999999999716, 0.000000000000000000 ) ) ;
#46793=CARTESIAN_POINT ( 'NONE',  ( 0.7681833999686413783, -81.32291666666667140, 0.9995835529977274980 ) ) ;
#46797=CARTESIAN_POINT ( 'NONE',  ( 1.249999999999999778, -79.76041666666665719, 0.1636246173744711763 ) ) ;
#46799=CARTESIAN_POINT ( 'NONE',  ( 1.539929345890999945, -79.97582157143999382, 0.3781723503825999422 ) ) ;
#46832=CARTESIAN_POINT ( 'NONE',  ( 1.217465845835394855, -82.72916666666667140, -0.3271848554490981997 ) ) ;
#46840=DIRECTION ( 'NONE',  ( 0.000000000000000000, -1.000000000000000000, 0.000000000000000000 ) ) ;
#46845=ORIENTED_EDGE ( 'NONE', *, *, #54106, .T. ) ;
#46851=CARTESIAN_POINT ( 'NONE',  ( 0.3708152058599178957, -82.74916602882588279, -1.193631158523653424 ) ) ;
#46856=CARTESIAN_POINT ( 'NONE',  ( -1.374356897932604848, -78.71628694306663476, 0.6198793800460191683 ) ) ;
#46870=DIRECTION ( 'NONE',  ( -1.000000000000000000, 0.000000000000000000, 0.000000000000000000 ) ) ;
#46875=CARTESIAN_POINT ( 'NONE',  ( 0.6069111558698970788, -82.93513506220737952, 1.101446694455507913 ) ) ;
#46910=CARTESIAN_POINT ( 'NONE',  ( 0.2040051533403345885, -80.73872320341082798, -1.234301858716469580 ) ) ;
#46917=CARTESIAN_POINT ( 'NONE',  ( -0.7411337730108847888, -80.52597511522522211, 1.006651954983204700 ) ) ;
#46931=CARTESIAN_POINT ( 'NONE',  ( -9.500000000000000000, -87.20000000000000284, 0.000000000000000000 ) ) ;
#46936=CARTESIAN_POINT ( 'NONE',  ( -1.265047507048352449, -79.30228839861766232, 0.8556988754165529842 ) ) ;
#46942=AXIS2_PLACEMENT_3D ( 'NONE', #11166, #6423, #24727 ) ;
#46950=CARTESIAN_POINT ( 'NONE',  ( 1.274651354540000003, -83.24304616690000103, -0.4485964608026000167 ) ) ;
#46953=CARTESIAN_POINT ( 'NONE',  ( 1.250000000000000000, -78.75000000000000000, 0.000000000000000000 ) ) ;
#46959=CARTESIAN_POINT ( 'NONE',  ( 0.5113695407423999306, -82.42414080993400205, 1.250788716666000111 ) ) ;
#46979=CARTESIAN_POINT ( 'NONE',  ( -0.07738748721609896297, -81.48033942009458030, 1.247494957338889821 ) ) ;
#46981=CARTESIAN_POINT ( 'NONE',  ( 0.9995416268372391277, -82.29857430458693557, -0.7677867857872645585 ) ) ;
#46983=AXIS2_PLACEMENT_3D ( 'NONE', #9051, #232, #18211 ) ;
#47001=ORIENTED_EDGE ( 'NONE', *, *, #40352, .T. ) ;
#47011=CARTESIAN_POINT ( 'NONE',  ( -0.6794254437148999903, -78.92033711567999887, -1.478865823597000029 ) ) ;
#47020=CARTESIAN_POINT ( 'NONE',  ( -0.6472661464068000248, -81.23605406588998790, 1.575051776950999960 ) ) ;
#47029=CARTESIAN_POINT ( 'NONE',  ( 1.249469270068990001, -81.33640427608399648, -0.2274969907241829736 ) ) ;
#47044=CARTESIAN_POINT ( 'NONE',  ( -1.043587583837393806, -81.14777710806242794, -0.7040735577254533251 ) ) ;
#47047=CARTESIAN_POINT ( 'NONE',  ( -0.5187597050509943353, -80.00936726310753500, 1.137174289053646703 ) ) ;
#47054=CARTESIAN_POINT ( 'NONE',  ( -0.2340378853370451706, -82.13661640029980049, 1.530701560988515064 ) ) ;
#47056=CARTESIAN_POINT ( 'NONE',  ( -0.8258380295080043343, -79.66783667981496819, -0.9386737271208877020 ) ) ;
#47060=CARTESIAN_POINT ( 'NONE',  ( -0.4746745519540126468, -81.69413255355395620, -1.156278043614258566 ) ) ;
#47061=SURFACE_STYLE_USAGE ( .BOTH. , #50607 ) ;
#47063=CARTESIAN_POINT ( 'NONE',  ( -0.9465222407332000154, -81.55663953507000485, -0.8164530897714000757 ) ) ;
#47068=ORIENTED_EDGE ( 'NONE', *, *, #23705, .T. ) ;
#47086=CARTESIAN_POINT ( 'NONE',  ( -1.092232985442824100, -79.95833333333330017, 0.6295237254636200097 ) ) ;
#47088=CARTESIAN_POINT ( 'NONE',  ( -1.551612880221999946, -79.72318471100000181, -0.3269472641410000047 ) ) ;
#47090=CARTESIAN_POINT ( 'NONE',  ( 1.024262641765716131, -79.56571245190475850, 1.112022483175320708 ) ) ;
#47094=DIRECTION ( 'NONE',  ( 0.000000000000000000, -1.000000000000000000, 0.000000000000000000 ) ) ;
#47108=CARTESIAN_POINT ( 'NONE',  ( -0.0005049683876466860800, -78.47525317868688433, 1.249867733114310431 ) ) ;
#47115=AXIS2_PLACEMENT_3D ( 'NONE', #23440, #55028, #19597 ) ;
#47121=LINE ( 'NONE', #34077, #6936 ) ;
#47137=ORIENTED_EDGE ( 'NONE', *, *, #51070, .T. ) ;
#47148=CARTESIAN_POINT ( 'NONE',  ( 0.3445775672978685367, -79.45339798296083700, 1.202313393638915873 ) ) ;
#47149=CARTESIAN_POINT ( 'NONE',  ( 1.051388242708131360, -77.93485489348125839, -1.116012858508012018 ) ) ;
#47168=CARTESIAN_POINT ( 'NONE',  ( 0.7966631500014442757, -82.92057275665307259, 0.9633609681394961211 ) ) ;
#47170=CARTESIAN_POINT ( 'NONE',  ( -0.6295237254636286695, -80.41666666666665719, 1.092232985442819881 ) ) ;
#47171=CARTESIAN_POINT ( 'NONE',  ( 1.250000000000000000, -78.25000000000000000, 0.000000000000000000 ) ) ;
#47175=CIRCLE ( 'NONE', #31100, 2.500000000000000000 ) ;
#47179=SURFACE_SIDE_STYLE ('',( #6416 ) ) ;
#47191=CARTESIAN_POINT ( 'NONE',  ( -1.508789225394999933, -82.35398503822999317, 0.7062677124845000431 ) ) ;
#47204=CARTESIAN_POINT ( 'NONE',  ( 1.093630560900841653, -80.80912397737533581, -0.6301138695088878139 ) ) ;
#47210=CARTESIAN_POINT ( 'NONE',  ( 0.6852450043578414141, -80.42895784771916112, 1.045337512399482582 ) ) ;
#47225=CARTESIAN_POINT ( 'NONE',  ( -1.119858561985657586, -78.40994284158009009, -1.052207020318775443 ) ) ;
#47238=ORIENTED_EDGE ( 'NONE', *, *, #58046, .T. ) ;
#47239=CARTESIAN_POINT ( 'NONE',  ( 1.458792785548086002, -80.02118756087138252, 0.3985484442472759792 ) ) ;
#47247=CARTESIAN_POINT ( 'NONE',  ( 0.4072933538588000002, -81.72938944371999526, -1.288442219433000080 ) ) ;
#47249=ORIENTED_EDGE ( 'NONE', *, *, #38361, .T. ) ;
#47274=CARTESIAN_POINT ( 'NONE',  ( 0.3106417784598000109, -79.22556961838999712, -1.176384596728999865 ) ) ;
#47292=CARTESIAN_POINT ( 'NONE',  ( -2.899999999413999774, -80.69999999940999658, -1.301622169156000167E-09 ) ) ;
#47303=CARTESIAN_POINT ( 'NONE',  ( 0.1742577344548000007, -77.69534258052999576, 1.489843697164999980 ) ) ;
#47310=CARTESIAN_POINT ( 'NONE',  ( 0.8701072296501000114, -80.16234740900999611, 1.463806805601000072 ) ) ;
#47314=AXIS2_PLACEMENT_3D ( 'NONE', #39322, #42609, #39035 ) ;
#47321=DIRECTION ( 'NONE',  ( -1.000000000000000000, 0.000000000000000000, 0.000000000000000000 ) ) ;
#47338=CARTESIAN_POINT ( 'NONE',  ( -1.113964114829858021, -80.06227650713580601, 0.5734498748148272318 ) ) ;
#47346=CARTESIAN_POINT ( 'NONE',  ( -1.064943818649878970, -81.91207579107143033, -1.072564683137462893 ) ) ;
#47377=CARTESIAN_POINT ( 'NONE',  ( 0.6690176526880000640, -81.11284491707999678, 1.565960205386000004 ) ) ;
#47395=CARTESIAN_POINT ( 'NONE',  ( 1.250000000000000000, -78.35000000000000853, 0.000000000000000000 ) ) ;
#47398=CIRCLE ( 'NONE', #37965, 3.000000000000000000 ) ;
#47424=ORIENTED_EDGE ( 'NONE', *, *, #28852, .T. ) ;
#47426=CARTESIAN_POINT ( 'NONE',  ( 3.000000000000000000, -86.20000000000000284, 0.000000000000000000 ) ) ;
#47433=CARTESIAN_POINT ( 'NONE',  ( 0.7382888704586531015, -82.77565560264896760, -1.008472483837859368 ) ) ;
#47438=CARTESIAN_POINT ( 'NONE',  ( 1.470702262612896716, -78.52302955446236865, 0.4327831235184762537 ) ) ;
#47448=EDGE_CURVE ( 'NONE', #16901, #19957, #32220, .T. ) ;
#47462=CARTESIAN_POINT ( 'NONE',  ( 0.4094730476285221021, -82.94845345813016024, 1.181202292546965182 ) ) ;
#47485=CARTESIAN_POINT ( 'NONE',  ( -1.561527218546999940, -82.41714425333900351, -0.5804237711334999661 ) ) ;
#47502=CARTESIAN_POINT ( 'NONE',  ( -0.8989222131784045944, -80.53948156304845440, 0.8681004554801105000 ) ) ;
#47519=CARTESIAN_POINT ( 'NONE',  ( 0.4630162960789051541, -77.99946388533825825, -1.437486996108025217 ) ) ;
#47529=CARTESIAN_POINT ( 'NONE',  ( -0.3271848554490991434, -78.60416666666665719, -1.217465845835395299 ) ) ;
#47532=B_SPLINE_SURFACE_WITH_KNOTS ( 'NONE', 3, 3, ( 
 ( #44736, #31424, #4287, #57717, #22287, #13423, #17874, #35864, #53893, #49467, #9014, #27000, #35265, #45035, #4586, #25844, #3421, #195, #34977, #18170, #39429, #33173, #50051, #45626, #45330, #42054, #9597, #1335, #50339, #5739, #46505, #55629, #19330, #1625, #55338 ),
 ( #18457, #37322, #4880, #9890, #19616, #28457, #9304, #46212, #5167, #36448, #18745, #15181, #27871, #23167, #54477, #14883, #45917, #41175, #37614, #32878, #6030, #14299, #27583, #50922, #10471, #36738, #768, #27293, #5452, #24039, #41467, #22877, #40887, #478, #14012 ),
 ( #55044, #23455, #54756, #32010, #50635, #1053, #10183, #19038, #37030, #14593, #32586, #28161, #23746, #34045, #51797, #24915, #29049, #43219, #2776, #51218, #24628, #2206, #46799, #29616, #15766, #20775, #47088, #6325, #47957, #37905, #7488, #3065, #16354, #38197, #25486 ),
 ( #42934, #2488, #51509, #16060, #29330, #47377, #25199, #42353, #56217, #42639, #20492, #55929, #21061, #24342, #39062, #6907, #6617, #11352, #11067, #16638, #57076, #38489, #56505, #52083, #15480, #33760, #56794, #10770, #28749, #43506, #1920, #11641, #33471, #19914, #20205 ) ),
 .UNSPECIFIED., .F., .F., .F.,
 ( 4, 4 ),
 ( 4, 1, 1, 1, 1, 1, 1, 1, 1, 1, 1, 1, 1, 1, 1, 1, 1, 1, 1, 1, 1, 1, 1, 1, 1, 1, 1, 1, 1, 1, 1, 1, 4 ),
 ( -0.1331668876848000060, 1.133166887685000068 ),
 ( -0.02000000000000000042, 0.01250000000000000069, 0.04499999999999999833, 0.07749999999999999944, 0.1100000000000000006, 0.1424999999999999878, 0.1749999999999999889, 0.2074999999999999900, 0.2399999999999999911, 0.2725000000000000200, 0.3049999999999999933, 0.3375000000000000222, 0.3699999999999999956, 0.4025000000000000244, 0.4349999999999999978, 0.4675000000000000266, 0.5000000000000000000, 0.5324999999999999734, 0.5649999999999999467, 0.5975000000000000311, 0.6300000000000000044, 0.6624999999999999778, 0.6949999999999999512, 0.7275000000000000355, 0.7600000000000000089, 0.7924999999999999822, 0.8249999999999999556, 0.8575000000000000400, 0.8900000000000000133, 0.9224999999999999867, 0.9549999999999999600, 0.9875000000000000444, 1.020000000000000018 ),
 .UNSPECIFIED. ) ;
#47535=CARTESIAN_POINT ( 'NONE',  ( 0.3137356748008011120, -80.89165110245198775, -1.478359838030668172 ) ) ;
#47545=CARTESIAN_POINT ( 'NONE',  ( -1.512180334517000180, -83.18236633857299012, 0.4761993468540999808 ) ) ;
#47556=ORIENTED_EDGE ( 'NONE', *, *, #8876, .T. ) ;
#47561=CARTESIAN_POINT ( 'NONE',  ( -0.1487011411093689672, -81.48479960741362049, 1.241381877223513897 ) ) ;
#47564=CARTESIAN_POINT ( 'NONE',  ( -1.249826857837516236, -82.11106099827752303, -0.1638645779436204153 ) ) ;
#47576=CARTESIAN_POINT ( 'NONE',  ( 1.168308732057000032, -78.34511805113000094, -0.8096088536258000401 ) ) ;
#47592=CARTESIAN_POINT ( 'NONE',  ( 1.250000000000000000, -83.24999999999998579, 0.000000000000000000 ) ) ;
#47597=CARTESIAN_POINT ( 'NONE',  ( -0.8961266428360998848, -77.75102415030998770, 1.358359200922999888 ) ) ;
#47607=CARTESIAN_POINT ( 'NONE',  ( 0.5538255850406000880, -81.04673389420999285, -1.485824439479999981 ) ) ;
#47615=CARTESIAN_POINT ( 'NONE',  ( 0.5926408534130915839, -81.26475886697264173, -1.100658270916459847 ) ) ;
#47622=VECTOR ( 'NONE', #21101, 1000.000000000000000 ) ;
#47627=CARTESIAN_POINT ( 'NONE',  ( -1.211372597667456974, -79.40044640989285085, -0.9001875127581699942 ) ) ;
#47633=ORIENTED_EDGE ( 'NONE', *, *, #48957, .T. ) ;
#47634=CARTESIAN_POINT ( 'NONE',  ( -0.02557347534276610546, -79.97707957153141933, 1.249510814140374126 ) ) ;
#47640=CARTESIAN_POINT ( 'NONE',  ( -1.509086691184912343, -82.85341321873580966, -0.07812501990390177675 ) ) ;
#47641=CARTESIAN_POINT ( 'NONE',  ( -1.109799271607774029, -79.63855864794726358, -0.5747890205896009075 ) ) ;
#47669=CARTESIAN_POINT ( 'NONE',  ( 1.250000000000000000, -79.75000000000000000, 0.000000000000000000 ) ) ;
#47672=CARTESIAN_POINT ( 'NONE',  ( -0.9995835529977249445, -81.05208333333334281, -0.7681833999686439318 ) ) ;
#47688=CARTESIAN_POINT ( 'NONE',  ( 0.9450313017535940663, -78.40681886214652252, 0.8189801504775520158 ) ) ;
#47692=DIRECTION ( 'NONE',  ( 0.000000000000000000, -1.000000000000000000, 0.000000000000000000 ) ) ;
#47699=CARTESIAN_POINT ( 'NONE',  ( -0.8980135761429828278, -82.03944583936498702, 0.8691029177942691808 ) ) ;
#47709=CARTESIAN_POINT ( 'NONE',  ( 1.092232985442820992, -81.79166666666667140, 0.6295237254636267821 ) ) ;
#47725=CARTESIAN_POINT ( 'NONE',  ( 0.4576869496836571405, -79.44562341424763474, 1.163108042213991444 ) ) ;
#47726=CARTESIAN_POINT ( 'NONE',  ( -1.058013582825246601, -78.18692974818745256, 1.074266245500460570 ) ) ;
#47742=CARTESIAN_POINT ( 'NONE',  ( 1.250000000000000000, -82.34999999999999432, 0.000000000000000000 ) ) ;
#47773=CIRCLE ( 'NONE', #25106, 1.250000000000000000 ) ;
#47783=CARTESIAN_POINT ( 'NONE',  ( -0.2838824429006977512, -80.49333599480686985, 1.217375917920300532 ) ) ;
#47789=ADVANCED_FACE ( 'NONE', ( #46353 ), #37461, .F. ) ;
#47811=CARTESIAN_POINT ( 'NONE',  ( -1.092232985442822102, -78.54166666666664298, -0.6295237254636245616 ) ) ;
#47812=AXIS2_PLACEMENT_3D ( 'NONE', #21191, #44214, #20623 ) ;
#47813=CARTESIAN_POINT ( 'NONE',  ( -0.4436761913305327099, -80.64873104433648621, 1.445706986503831892 ) ) ;
#47815=CARTESIAN_POINT ( 'NONE',  ( -1.250000000000000000, -79.00000000000000000, 0.000000000000000000 ) ) ;
#47824=CARTESIAN_POINT ( 'NONE',  ( 1.308628125960000110, -81.85586534759998756, -0.6662886516973000051 ) ) ;
#47842=CARTESIAN_POINT ( 'NONE',  ( -1.497546582071999977, -80.79352275519998727, 0.7298035716741000378 ) ) ;
#47879=CARTESIAN_POINT ( 'NONE',  ( 1.623578234368999951, -78.08511356898999622, 0.1125035222880000074 ) ) ;
#47880=CARTESIAN_POINT ( 'NONE',  ( 0.000000000000000000, -80.69999999999998863, 0.000000000000000000 ) ) ;
#47888=CARTESIAN_POINT ( 'NONE',  ( 0.5386432692752000095, -83.17941453081499503, 1.615427185862999826 ) ) ;
#47889=CARTESIAN_POINT ( 'NONE',  ( -0.3737996561424999920, -80.35214000165998982, 1.420113360969999849 ) ) ;
#47897=CARTESIAN_POINT ( 'NONE',  ( 1.250000000000000000, -81.34999999999999432, 0.000000000000000000 ) ) ;
#47898=ADVANCED_FACE ( 'NONE', ( #24769 ), #56931, .T. ) ;
#47900=CARTESIAN_POINT ( 'NONE',  ( -1.250000000000000000, -78.00000000000000000, 2.658254822585999717E-14 ) ) ;
#47901=DIRECTION ( 'NONE',  ( 0.000000000000000000, 1.000000000000000000, 0.000000000000000000 ) ) ;
#47907=VECTOR ( 'NONE', #17544, 1000.000000000000000 ) ;
#47909=CARTESIAN_POINT ( 'NONE',  ( -1.561527218546999940, -82.35792792946999441, -0.5804237711334999661 ) ) ;
#47911=CARTESIAN_POINT ( 'NONE',  ( -1.493873713138741843, -79.33798222089950514, 0.2208649169497922671 ) ) ;
#47925=CARTESIAN_POINT ( 'NONE',  ( 0.04925494599860675421, -82.72182841701953748, 1.510347986472535320 ) ) ;
#47939=CARTESIAN_POINT ( 'NONE',  ( -0.1861229965304324052, -77.82161458351710337, -1.428385417274072422 ) ) ;
#47957=CARTESIAN_POINT ( 'NONE',  ( -0.3011984493834000132, -79.59686628078000581, 1.556817658704999996 ) ) ;
#47971=CARTESIAN_POINT ( 'NONE',  ( 1.189217420461008423, -78.37516310198307679, 0.3845707844590672830 ) ) ;
#47986=CARTESIAN_POINT ( 'NONE',  ( 1.224722617583677176, -81.86616265547245064, 0.2496387431639754406 ) ) ;
#47997=EDGE_CURVE ( 'NONE', #36547, #7212, #51338, .T. ) ;
#47999=CARTESIAN_POINT ( 'NONE',  ( -1.072483829238511044, -81.25721727793691684, -0.9250620443464491194 ) ) ;
#48009=CARTESIAN_POINT ( 'NONE',  ( 0.2479148173105888420, -82.74134425127877535, -1.224891232295899801 ) ) ;
#48013=CARTESIAN_POINT ( 'NONE',  ( 0.8760958855005448465, -79.41347816698738882, 0.8914155223916401249 ) ) ;
#48026=B_SPLINE_CURVE_WITH_KNOTS ( 'NONE', 3,
 ( #8346, #40223, #45254, #57647, #40522, #27216, #53513, #44360, #18093, #54105, #57941, #40815, #30766, #13349, #48799, #8060, #115, #31347 ),
 .UNSPECIFIED., .F., .F.,
 ( 4, 2, 2, 2, 2, 2, 2, 2, 4 ),
 ( 0.000000000000000000, 0.1250000000000000833, 0.2500000000000001110, 0.3750000000000000000, 0.4999999999999999445, 0.6249999999999998890, 0.7499999999999997780, 0.8749999999999998890, 1.000000000000000000 ),
 .UNSPECIFIED. ) ;
#48047=ORIENTED_EDGE ( 'NONE', *, *, #7090, .T. ) ;
#48075=CARTESIAN_POINT ( 'NONE',  ( 0.6303254723250644176, -80.43299358135132593, 1.079794037324565581 ) ) ;
#48098=CARTESIAN_POINT ( 'NONE',  ( 1.504090402702771501, -80.99286779333345976, -0.1339503099265954567 ) ) ;
#48099=CARTESIAN_POINT ( 'NONE',  ( -3.000000000000000000, -86.20000000000000284, 0.000000000000000000 ) ) ;
#48108=CARTESIAN_POINT ( 'NONE',  ( -0.7208041749482999583, -83.11920712346199025, 1.412512638229999951 ) ) ;
#48111=CARTESIAN_POINT ( 'NONE',  ( 0.1636246173744697330, -82.13541666666665719, -1.249999999999999778 ) ) ;
#48126=CARTESIAN_POINT ( 'NONE',  ( -1.630114970985000022, -79.78691820467999207, -0.3434887894992000312 ) ) ;
#48131=CARTESIAN_POINT ( 'NONE',  ( -0.9994139296504542802, -82.15273062190185271, -0.7675533749920089299 ) ) ;
#48136=CARTESIAN_POINT ( 'NONE',  ( 0.000000000000000000, -77.59999999938000315, -2.399999999383999771 ) ) ;
#48164=CYLINDRICAL_SURFACE ( 'NONE', #30402, 1.250000000000000000 ) ;
#48175=CARTESIAN_POINT ( 'NONE',  ( -1.596184505169000012, -82.35834473437999748, -0.5933059756569000198 ) ) ;
#48176=CARTESIAN_POINT ( 'NONE',  ( 0.8987165921316000450, -79.72039037689999930, 1.306408957324000086 ) ) ;
#48180=CARTESIAN_POINT ( 'NONE',  ( -1.374853770045000090, -81.25000091166998573, -0.7192078502473999713 ) ) ;
#48193=CARTESIAN_POINT ( 'NONE',  ( 0.8286895765316001361, -81.66317656325999508, 1.445177540541999983 ) ) ;
#48210=CARTESIAN_POINT ( 'NONE',  ( 1.098001230595262445, -82.66109697007367174, 1.088914393985984885 ) ) ;
#48211=CARTESIAN_POINT ( 'NONE',  ( -0.3740291581177058733, -79.70132840708080835, -1.192537797324159099 ) ) ;
#48227=EDGE_CURVE ( 'NONE', #53705, #12208, #20672, .T. ) ;
#48229=VERTEX_POINT ( 'NONE', #17924 ) ;
#48259=B_SPLINE_CURVE_WITH_KNOTS ( 'NONE', 3,
 ( #7486, #42351, #20489, #47086, #52366, #11350, #6322, #52081, #51795, #42932, #29046, #43217, #20773, #51216, #42637, #2204, #46797, #47669 ),
 .UNSPECIFIED., .F., .F.,
 ( 4, 2, 2, 2, 2, 2, 2, 2, 4 ),
 ( 0.000000000000000000, 0.1249999999999999722, 0.2500000000000000000, 0.3750000000000000000, 0.5000000000000001110, 0.6250000000000001110, 0.7500000000000000000, 0.8750000000000000000, 1.000000000000000000 ),
 .UNSPECIFIED. ) ;
#48261=STYLED_ITEM ( 'NONE', ( #24010 ), #34903 ) ;
#48272=CARTESIAN_POINT ( 'NONE',  ( 0.8795903431313560894, -81.91347361793080495, 0.8876339888831865643 ) ) ;
#48278=CARTESIAN_POINT ( 'NONE',  ( 0.000000000000000000, -76.75499999999999545, 0.000000000000000000 ) ) ;
#48281=CARTESIAN_POINT ( 'NONE',  ( -0.9995866622284782510, -78.15219033508832069, -0.7680681559914127599 ) ) ;
#48338=VERTEX_POINT ( 'NONE', #51510 ) ;
#48366=CARTESIAN_POINT ( 'NONE',  ( -1.297604665245808642, -77.89238241849264455, -0.7720361663834586219 ) ) ;
#48372=CARTESIAN_POINT ( 'NONE',  ( -1.333333333333332815, -83.45000000000000284, 0.000000000000000000 ) ) ;
#48379=CARTESIAN_POINT ( 'NONE',  ( -0.7266214904040529943, -81.16493616783630216, 1.326165027772164828 ) ) ;
#48389=CARTESIAN_POINT ( 'NONE',  ( 1.457613149566999944, -82.42445575724998719, -0.6243081169531999874 ) ) ;
#48409=CARTESIAN_POINT ( 'NONE',  ( 1.617840321509000034, -80.03955506511998408, 0.3973055507782000118 ) ) ;
#48437=CARTESIAN_POINT ( 'NONE',  ( -0.3271848554490991434, -83.10416666666665719, -1.217465845835395299 ) ) ;
#48440=AXIS2_PLACEMENT_3D ( 'NONE', #6187, #6479, #10336 ) ;
#48446=FACE_OUTER_BOUND ( 'NONE', #29960, .T. ) ;
#48447=CARTESIAN_POINT ( 'NONE',  ( -0.8868929876605555762, -83.03844894029447232, 0.8802993065933630845 ) ) ;
#48451=CARTESIAN_POINT ( 'NONE',  ( 1.614964347157999747, -82.10570787394000547, 0.5400991692461000193 ) ) ;
#48452=CARTESIAN_POINT ( 'NONE',  ( 0.4206423954835999401, -80.60477686209999604, -1.406949933701999944 ) ) ;
#48453=CARTESIAN_POINT ( 'NONE',  ( -1.291666666665713281, -77.95833333333236226, 0.2617993877989879259 ) ) ;
#48457=CARTESIAN_POINT ( 'NONE',  ( -1.462746796095000024, -81.22894783996999024, -0.3322225316158000097 ) ) ;
#48468=CARTESIAN_POINT ( 'NONE',  ( 0.6304340365998000184, -82.67372400502100049, 1.542015542100000136 ) ) ;
#48510=CARTESIAN_POINT ( 'NONE',  ( -1.462188802161999979, -79.24735702617999777, -0.7147474581103999691 ) ) ;
#48549=CARTESIAN_POINT ( 'NONE',  ( 1.118667866065873318, -81.88699651758111031, 0.5575489754530202902 ) ) ;
#48581=CARTESIAN_POINT ( 'NONE',  ( -0.7509728292934746419, -77.83402495159873524, -1.337060448512992439 ) ) ;
#48621=EDGE_LOOP ( 'NONE', ( #56328, #4454, #10234, #50065 ) ) ;
#48627=EDGE_CURVE ( 'NONE', #14640, #44478, #26310, .T. ) ;
#48641=ORIENTED_EDGE ( 'NONE', *, *, #53545, .F. ) ;
#48656=CARTESIAN_POINT ( 'NONE',  ( -1.250000000000001332, -83.48958333333335702, 0.1636246173744632659 ) ) ;
#48662=CARTESIAN_POINT ( 'NONE',  ( 0.2751614629225042630, -79.98895914179001920, -1.487999588816689700 ) ) ;
#48672=CARTESIAN_POINT ( 'NONE',  ( -0.5511181765943999888, -82.80341104791099838, -1.486830790314999984 ) ) ;
#48675=ORIENTED_EDGE ( 'NONE', *, *, #37768, .F. ) ;
#48690=LINE ( 'NONE', #35670, #13855 ) ;
#48692=ORIENTED_EDGE ( 'NONE', *, *, #19862, .F. ) ;
#48711=CARTESIAN_POINT ( 'NONE',  ( 0.4901547383881838527, -80.25723238900481249, -1.149788170831134382 ) ) ;
#48717=CARTESIAN_POINT ( 'NONE',  ( 1.250000000000000000, -82.84999999999999432, 0.000000000000000000 ) ) ;
#48733=CARTESIAN_POINT ( 'NONE',  ( -1.155223306477086931, -83.06892497275070752, 0.4772783199500317819 ) ) ;
#48737=CARTESIAN_POINT ( 'NONE',  ( 0.6735630312197999903, -83.05325357425300581, -1.435516540950999786 ) ) ;
#48738=CARTESIAN_POINT ( 'NONE',  ( -0.5136231202413000796, -81.42600413218998767, 1.249846006485000105 ) ) ;
#48743=CARTESIAN_POINT ( 'NONE',  ( 0.5269479332349999989, -83.11978140203299859, 1.580352090963000000 ) ) ;
#48750=CARTESIAN_POINT ( 'NONE',  ( -0.4767998270009902728, -79.59439922511664633, -1.192942613436671406 ) ) ;
#48762=CARTESIAN_POINT ( 'NONE',  ( 0.8738424494231588069, -79.91383025740681489, 0.8934342867657290022 ) ) ;
#48765=CIRCLE ( 'NONE', #22331, 1.750000000000000000 ) ;
#48799=CARTESIAN_POINT ( 'NONE',  ( -1.092232985442822102, -78.04166666666664298, -0.6295237254636245616 ) ) ;
#48819=ORIENTED_EDGE ( 'NONE', *, *, #19355, .F. ) ;
#48835=CARTESIAN_POINT ( 'NONE',  ( -0.03524841727520977575, -81.97784558154000933, 1.249284716020608421 ) ) ;
#48836=CARTESIAN_POINT ( 'NONE',  ( -0.8529715180118000450, -77.81475764398999218, 1.292944160158000066 ) ) ;
#48838=CARTESIAN_POINT ( 'NONE',  ( -0.9512744292220589593, -83.17914831638273654, 1.173546308381462122 ) ) ;
#48841=CARTESIAN_POINT ( 'NONE',  ( -2.500000000000000000, -80.69999999999998863, 0.000000000000000000 ) ) ;
#48843=CARTESIAN_POINT ( 'NONE',  ( 0.5039928918671183755, -81.75818078180917325, -1.143829648980971836 ) ) ;
#48851=EDGE_CURVE ( 'NONE', #3682, #15743, #34768, .T. ) ;
#48879=CARTESIAN_POINT ( 'NONE',  ( 10.14999999998000035, -87.10000000002298748, -2.878934427392999978E-10 ) ) ;
#48883=CIRCLE ( 'NONE', #23427, 2.899999999999999911 ) ;
#48909=VERTEX_POINT ( 'NONE', #29536 ) ;
#48913=ORIENTED_EDGE ( 'NONE', *, *, #50687, .T. ) ;
#48919=VERTEX_POINT ( 'NONE', #20980 ) ;
#48941=CARTESIAN_POINT ( 'NONE',  ( -1.416666666666666519, -83.39999999999999147, 0.000000000000000000 ) ) ;
#48947=CARTESIAN_POINT ( 'NONE',  ( 0.1636246173744642929, -80.86458333333331439, 1.250000000000000888 ) ) ;
#48949=CARTESIAN_POINT ( 'NONE',  ( 1.466761443839349921, -80.08005631220875387, -0.3644506899237003328 ) ) ;
#48950=CARTESIAN_POINT ( 'NONE',  ( -1.193943581762582529, -78.57580789766646490, 0.3796058497236899920 ) ) ;
#48957=EDGE_CURVE ( 'NONE', #17800, #32925, #41688, .T. ) ;
#48960=CARTESIAN_POINT ( 'NONE',  ( -1.586699731716999962, -82.74040930645999481, 0.6182239771991999699 ) ) ;
#48976=FACE_OUTER_BOUND ( 'NONE', #19962, .T. ) ;
#48980=ORIENTED_EDGE ( 'NONE', *, *, #21040, .F. ) ;
#48983=DIRECTION ( 'NONE',  ( 1.000000000000000000, 0.000000000000000000, 0.000000000000000000 ) ) ;
#48993=CARTESIAN_POINT ( 'NONE',  ( -1.140637725705999861, -79.20579340557999615, 1.189889555309999958 ) ) ;
#48996=CARTESIAN_POINT ( 'NONE',  ( -1.262801891034090351, -79.29605910888498954, -0.8245544024085487145 ) ) ;
#48997=CARTESIAN_POINT ( 'NONE',  ( 0.4103876590417050441, -80.25167417027007843, -1.183805647784901494 ) ) ;
#49012=AXIS2_PLACEMENT_3D ( 'NONE', #44776, #41217, #22630 ) ;
#49014=CARTESIAN_POINT ( 'NONE',  ( 10.14999999999999858, -86.39999999999999147, 0.000000000000000000 ) ) ;
#49025=CARTESIAN_POINT ( 'NONE',  ( -0.5793938177159999592, -82.86393340258099727, 1.349352049262000142 ) ) ;
#49026=CARTESIAN_POINT ( 'NONE',  ( 1.288070761429999989, -80.79441198108999345, 0.4084665662698999666 ) ) ;
#49029=CARTESIAN_POINT ( 'NONE',  ( 1.750000000000000000, -77.50000000000000000, 0.000000000000000000 ) ) ;
#49051=CARTESIAN_POINT ( 'NONE',  ( 0.6919073629492709099, -79.92850570978326630, 1.042099490686354990 ) ) ;
#49052=DIRECTION ( 'NONE',  ( -1.000000000000000000, 0.000000000000000000, 0.000000000000000000 ) ) ;
#49075=CARTESIAN_POINT ( 'NONE',  ( -0.9956369009631184097, -79.54819107059427097, 0.7605103355424140954 ) ) ;
#49084=CARTESIAN_POINT ( 'NONE',  ( 1.619712389308999967, -78.96894917727999541, 0.1587296492880999887 ) ) ;
#49087=EDGE_CURVE ( 'NONE', #10981, #19814, #27635, .T. ) ;
#49123=CARTESIAN_POINT ( 'NONE',  ( 0.7831030525921437446, -81.92154750067230395, 0.9747994925984700965 ) ) ;
#49124=CARTESIAN_POINT ( 'NONE',  ( -1.601737029647000154, -78.30825665301999550, 0.4494192519392999907 ) ) ;
#49126=CARTESIAN_POINT ( 'NONE',  ( -1.505894968352336827, -82.74391654559087783, 0.1164684639126788851 ) ) ;
#49194=CARTESIAN_POINT ( 'NONE',  ( -0.3271848554491046945, -82.39583333333330017, 1.217465845835393301 ) ) ;
#49204=CARTESIAN_POINT ( 'NONE',  ( 0.000000000000000000, -76.75499999999999545, 0.000000000000000000 ) ) ;
#49241=CARTESIAN_POINT ( 'NONE',  ( 0.8080229617562444400, -80.01932486526288812, -1.277038703091432748 ) ) ;
#49242=CARTESIAN_POINT ( 'NONE',  ( -1.054090230153319485, -78.55495177038956456, 0.6754526289925347760 ) ) ;
#49251=CARTESIAN_POINT ( 'NONE',  ( 1.529418508686999800, -83.05620538201100089, 0.7487957062819000642 ) ) ;
#49267=FACE_OUTER_BOUND ( 'NONE', #3466, .T. ) ;
#49274=CARTESIAN_POINT ( 'NONE',  ( 0.3704480504712000521, -80.03166928263999580, -1.624200486671999899 ) ) ;
#49289=CARTESIAN_POINT ( 'NONE',  ( -0.2341392558410000102, -78.09384532121998745, 1.516891056133000015 ) ) ;
#49293=CARTESIAN_POINT ( 'NONE',  ( 1.181968933961157653, -80.32389716667498192, -0.4063731449358948256 ) ) ;
#49320=CARTESIAN_POINT ( 'NONE',  ( -1.308644393797000038, -81.43216705308998371, -0.6845726736234999388 ) ) ;
#49321=CARTESIAN_POINT ( 'NONE',  ( 1.218119833583123146, -78.82945698446253857, -0.3274011781227666451 ) ) ;
#49325=B_SPLINE_CURVE_WITH_KNOTS ( 'NONE', 3,
 ( #35334, #48656, #8785, #3207, #12627, #25625, #57499, #52502, #8200, #25912, #44220, #26481, #12060, #3769, #58083, #22059, #30623, #21772 ),
 .UNSPECIFIED., .F., .F.,
 ( 4, 2, 2, 2, 2, 2, 2, 2, 4 ),
 ( 0.000000000000000000, 0.1249999999999999722, 0.2500000000000000000, 0.3750000000000000000, 0.5000000000000001110, 0.6250000000000001110, 0.7500000000000000000, 0.8750000000000000000, 1.000000000000000000 ),
 .UNSPECIFIED. ) ;
#49326=CIRCLE ( 'NONE', #16295, 3.000000000000000000 ) ;
#49343=CARTESIAN_POINT ( 'NONE',  ( 0.5189408976694140918, -79.25928653513095412, -1.150586733911741932 ) ) ;
#49366=ORIENTED_EDGE ( 'NONE', *, *, #51188, .T. ) ;
#49372=CARTESIAN_POINT ( 'NONE',  ( -1.250000000000000000, -82.99999999999998579, 0.000000000000000000 ) ) ;
#49408=ORIENTED_EDGE ( 'NONE', *, *, #52709, .T. ) ;
#49424=CARTESIAN_POINT ( 'NONE',  ( 0.9441861370063999725, -79.53822423548000131, 1.372505234203999835 ) ) ;
#49425=CARTESIAN_POINT ( 'NONE',  ( 0.3963282436660999775, -77.97416723434000119, -1.615693196437999912 ) ) ;
#49427=CARTESIAN_POINT ( 'NONE',  ( 1.545316077588782866, -82.50099648747466574, 0.02805363615183451356 ) ) ;
#49433=CARTESIAN_POINT ( 'NONE',  ( 1.094998213286220823, -81.80994750764530465, -0.6032700728990865180 ) ) ;
#49439=ORIENTED_EDGE ( 'NONE', *, *, #43576, .T. ) ;
#49467=CARTESIAN_POINT ( 'NONE',  ( -0.5717664302369001028, -80.67025799034000499, -1.224358761826999986 ) ) ;
#49502=CYLINDRICAL_SURFACE ( 'NONE', #46983, 1.250000000000000000 ) ;
#49511=ORIENTED_EDGE ( 'NONE', *, *, #31790, .T. ) ;
#49532=DIRECTION ( 'NONE',  ( 0.000000000000000000, 1.000000000000000000, 0.000000000000000000 ) ) ;
#49538=CARTESIAN_POINT ( 'NONE',  ( 1.210984793496805656, -79.72721317835664934, -0.3578339234309608208 ) ) ;
#49546=CARTESIAN_POINT ( 'NONE',  ( 1.292974957763964872, -81.14285663376836055, 0.7849688150825027133 ) ) ;
#49547=CARTESIAN_POINT ( 'NONE',  ( -1.085375040598030250, -78.55880290454010151, 0.6235288048130009919 ) ) ;
#49577=CARTESIAN_POINT ( 'NONE',  ( 1.417725061834000044, -80.09482849775000091, -0.8748226493128999914 ) ) ;
#49581=ADVANCED_FACE ( 'NONE', ( #14969 ), #9388, .F. ) ;
#49592=CARTESIAN_POINT ( 'NONE',  ( 0.7985095004294999743, -78.10473044020999112, 1.441967081790000105 ) ) ;
#49620=CARTESIAN_POINT ( 'NONE',  ( 0.6000739755967000599, -82.73745749870199973, 1.467756090344000119 ) ) ;
#49621=CARTESIAN_POINT ( 'NONE',  ( -0.3439666625990999704, -80.41545669043000544, 1.306773950318999900 ) ) ;
#49639=CARTESIAN_POINT ( 'NONE',  ( -0.3862712429687000237, -78.00000000000000000, 1.188820645369000006 ) ) ;
#49646=CARTESIAN_POINT ( 'NONE',  ( -0.9860104425937412653, -81.54762977175269612, 0.7687338358433186691 ) ) ;
#49662=ORIENTED_EDGE ( 'NONE', *, *, #19862, .T. ) ;
#49667=DIRECTION ( 'NONE',  ( 0.000000000000000000, -1.000000000000000000, -1.853433557485999982E-14 ) ) ;
#49682=CARTESIAN_POINT ( 'NONE',  ( -0.7213013439201000354, -77.85885253578000231, -1.458901041394999876 ) ) ;
#49688=ORIENTED_EDGE ( 'NONE', *, *, #33087, .F. ) ;
#49699=CARTESIAN_POINT ( 'NONE',  ( 0.000000000000000000, -87.09999999999999432, -10.15000000000498659 ) ) ;
#49712=AXIS2_PLACEMENT_3D ( 'NONE', #11080, #34057, #46518 ) ;
#49718=DIRECTION ( 'NONE',  ( 0.000000000000000000, -1.000000000000000000, 0.000000000000000000 ) ) ;
#49723=CARTESIAN_POINT ( 'NONE',  ( -1.497546582071999977, -80.73430643132999762, 0.7298035716741000378 ) ) ;
#49724=CARTESIAN_POINT ( 'NONE',  ( 0.4117780953839000335, -79.03975217913999529, -1.493365003632999954 ) ) ;
#49744=CARTESIAN_POINT ( 'NONE',  ( 1.122609662881488113, -80.38645885631675014, 0.5495315797171209660 ) ) ;
#49802=ORIENTED_EDGE ( 'NONE', *, *, #30681, .F. ) ;
#49815=CARTESIAN_POINT ( 'NONE',  ( 0.8873640354812792896, -82.78847969525013184, -0.8798066330654785716 ) ) ;
#49824=CARTESIAN_POINT ( 'NONE',  ( 10.05000000000000071, -87.20000000000000284, 0.000000000000000000 ) ) ;
#49839=ADVANCED_FACE ( 'NONE', ( #16007 ), #29565, .F. ) ;
#49842=CARTESIAN_POINT ( 'NONE',  ( 1.491372860315189230, -81.11249091029543479, 0.2478840690545696945 ) ) ;
#49844=CARTESIAN_POINT ( 'NONE',  ( -0.3473130761334148331, -78.49761955947900560, 1.203549973938182527 ) ) ;
#49847=PRODUCT ( 'Push Button', 'Push Button', '', ( #42916 ) ) ;
#49853=CARTESIAN_POINT ( 'NONE',  ( 0.4046438523804999909, -81.41406578915000125, -1.654233492563000008 ) ) ;
#49887=CARTESIAN_POINT ( 'NONE',  ( 1.645994068133999955, -78.52418299843999705, 0.08711949123553000551 ) ) ;
#49890=EDGE_CURVE ( 'NONE', #21051, #28446, #14237, .T. ) ;
#49891=CARTESIAN_POINT ( 'NONE',  ( 1.131496422793114576, -80.31479908467704831, -0.5381041634472353286 ) ) ;
#49912=CARTESIAN_POINT ( 'NONE',  ( -1.329983713389000011, -82.42181889680900042, 0.6225684403671000178 ) ) ;
#49919=CIRCLE ( 'NONE', #47115, 9.500000000000000000 ) ;
#49934=CARTESIAN_POINT ( 'NONE',  ( 1.250000000000000000, -79.34999999999999432, 0.000000000000000000 ) ) ;
#49941=CARTESIAN_POINT ( 'NONE',  ( -0.4845542736245379567, -81.50687699870314873, 1.152130999872969852 ) ) ;
#49951=ORIENTED_EDGE ( 'NONE', *, *, #45098, .F. ) ;
#49960=AXIS2_PLACEMENT_3D ( 'NONE', #56201, #1605, #55912 ) ;
#49963=CARTESIAN_POINT ( 'NONE',  ( 1.250000000000000000, -82.34999999999999432, 0.000000000000000000 ) ) ;
#49976=CARTESIAN_POINT ( 'NONE',  ( 0.08338359222296000406, -79.45859229021999681, -1.538001148114999994 ) ) ;
#50014=CARTESIAN_POINT ( 'NONE',  ( 1.097836406584000057, -78.70566276047000542, 1.092911459613999936 ) ) ;
#50016=CARTESIAN_POINT ( 'NONE',  ( 1.423276841203632515, -83.02732328005990325, 0.5108568199358340944 ) ) ;
#50022=CARTESIAN_POINT ( 'NONE',  ( 0.8955375890287041729, -81.78914646445058168, -0.8716670893819381538 ) ) ;
#50023=EDGE_CURVE ( 'NONE', #2755, #12936, #16393, .T. ) ;
#50044=CARTESIAN_POINT ( 'NONE',  ( 0.1636246173744642929, -81.36458333333332860, 1.250000000000000888 ) ) ;
#50051=CARTESIAN_POINT ( 'NONE',  ( 1.312293141192999890, -79.84918819389999101, 0.3222699683723999620 ) ) ;
#50060=LINE ( 'NONE', #9606, #5192 ) ;
#50065=ORIENTED_EDGE ( 'NONE', *, *, #14581, .F. ) ;
#50087=CARTESIAN_POINT ( 'NONE',  ( -0.1636246173744726473, -82.38541666666665719, 1.249999999999999112 ) ) ;
#50107=CARTESIAN_POINT ( 'NONE',  ( 0.8928342013463602678, -82.78896698447270808, -0.8742295960309274250 ) ) ;
#50124=DIRECTION ( 'NONE',  ( -1.000000000000000000, 0.000000000000000000, 0.000000000000000000 ) ) ;
#50132=DIRECTION ( 'NONE',  ( 1.000000000000000000, 0.000000000000000000, 0.000000000000000000 ) ) ;
#50134=CARTESIAN_POINT ( 'NONE',  ( 1.217465845835393967, -80.77083333333331439, 0.3271848554491025851 ) ) ;
#50136=CARTESIAN_POINT ( 'NONE',  ( -0.2201363562291999698, -79.46327907014000402, -1.483758735329000045 ) ) ;
#50140=CARTESIAN_POINT ( 'NONE',  ( 1.250000000000000222, -80.73958333333331439, -0.1636246173744659582 ) ) ;
#50145=CARTESIAN_POINT ( 'NONE',  ( 0.4779442704572000045, -81.85602282125999807, -1.511941137165000004 ) ) ;
#50158=VERTEX_POINT ( 'NONE', #248 ) ;
#50173=ORIENTED_EDGE ( 'NONE', *, *, #28325, .F. ) ;
#50177=CARTESIAN_POINT ( 'NONE',  ( -1.518142601816999893, -79.19490828658999249, 0.2258102331908000138 ) ) ;
#50180=CARTESIAN_POINT ( 'NONE',  ( -0.8807074628163545915, -80.16329956998615103, -0.8865880600332928241 ) ) ;
#50199=CARTESIAN_POINT ( 'NONE',  ( 0.4917238316050000502, -82.67461323090898873, -1.258641686703000140 ) ) ;
#50201=CARTESIAN_POINT ( 'NONE',  ( -1.250000000000001332, -79.48958333333334281, 0.1636246173744632659 ) ) ;
#50229=CARTESIAN_POINT ( 'NONE',  ( -1.154931660856736153, -81.56894284788815241, 0.4778881009946403524 ) ) ;
#50261=VECTOR ( 'NONE', #39785, 1000.000000000000000 ) ;
#50264=CARTESIAN_POINT ( 'NONE',  ( 0.08338359222296000406, -79.39937596634999295, -1.538001148114999994 ) ) ;
#50285=VERTEX_POINT ( 'NONE', #18232 ) ;
#50303=CARTESIAN_POINT ( 'NONE',  ( -1.445929428138999828, -80.22903271044999940, 0.8273736140038000508 ) ) ;
#50304=CARTESIAN_POINT ( 'NONE',  ( 1.316947385243999902, -78.27548044020998930, 0.09125597792054998547 ) ) ;
#50306=CARTESIAN_POINT ( 'NONE',  ( 1.364940739897916533, -81.96454802580129240, -0.6510407284856819521 ) ) ;
#50307=CARTESIAN_POINT ( 'NONE',  ( 1.424284261262790618, -83.12670472999310789, 0.5112557424970984865 ) ) ;
#50313=CARTESIAN_POINT ( 'NONE',  ( -1.184527705118542107, -81.62653070104380504, -0.4082925468394342783 ) ) ;
#50316=CARTESIAN_POINT ( 'NONE',  ( -1.250000000000000000, -80.00000000000000000, 0.000000000000000000 ) ) ;
#50339=CARTESIAN_POINT ( 'NONE',  ( -0.2566745418018999692, -79.47023290324000300, 1.326684981396999863 ) ) ;
#50358=CARTESIAN_POINT ( 'NONE',  ( 0.000000000000000000, -86.29999999996098836, 0.000000000000000000 ) ) ;
#50366=EDGE_CURVE ( 'NONE', #17800, #55505, #32646, .T. ) ;
#50407=VECTOR ( 'NONE', #34771, 1000.000000000000000 ) ;
#50435=ORIENTED_EDGE ( 'NONE', *, *, #50023, .F. ) ;
#50468=DIRECTION ( 'NONE',  ( 0.000000000000000000, -1.000000000000000000, -1.327216516273000122E-14 ) ) ;
#50472=CARTESIAN_POINT ( 'NONE',  ( -1.249805685293928548, -80.10851784185619806, -0.1286959038651522835 ) ) ;
#50476=CARTESIAN_POINT ( 'NONE',  ( -0.2142199289669327877, -78.96319708694683470, -1.521292673437905529 ) ) ;
#50492=CARTESIAN_POINT ( 'NONE',  ( 1.281517705925000028, -82.29565794024999548, 0.4285832374949000156 ) ) ;
#50521=CARTESIAN_POINT ( 'NONE',  ( -1.200102204978513942, -81.57785406893258084, 0.3492695309771673418 ) ) ;
#50525=CARTESIAN_POINT ( 'NONE',  ( -0.1375932915944000079, -78.96341176948999419, 1.300711684584999972 ) ) ;
#50528=AXIS2_PLACEMENT_3D ( 'NONE', #20945, #8517, #3801 ) ;
#50534=VERTEX_POINT ( 'NONE', #33237 ) ;
#50554=CARTESIAN_POINT ( 'NONE',  ( -1.578837173282999995, -79.31010810413999934, 0.3948290484592000271 ) ) ;
#50597=CARTESIAN_POINT ( 'NONE',  ( -0.3164372427141999844, -79.60138345058999221, 1.635583079321000000 ) ) ;
#50598=CARTESIAN_POINT ( 'NONE',  ( 0.3615948191998999972, -78.60193473990000257, -1.388282749240000058 ) ) ;
#50600=CARTESIAN_POINT ( 'NONE',  ( 0.1760362647577854434, -82.11637306212345777, 1.535881408346201127 ) ) ;
#50607=SURFACE_SIDE_STYLE ('',( #14272 ) ) ;
#50609=CARTESIAN_POINT ( 'NONE',  ( -1.009333286406026264, -81.50605136130415929, -0.8706792349393618347 ) ) ;
#50630=CARTESIAN_POINT ( 'NONE',  ( 0.000000000000000000, -78.00000000000000000, 0.000000000000000000 ) ) ;
#50635=CARTESIAN_POINT ( 'NONE',  ( -0.6027184710183000060, -81.11268744342000048, 1.466649853462000053 ) ) ;
#50675=DIRECTION ( 'NONE',  ( 1.000000000000000000, 0.000000000000000000, 0.000000000000000000 ) ) ;
#50687=EDGE_CURVE ( 'NONE', #54581, #36547, #8522, .T. ) ;
#50692=CARTESIAN_POINT ( 'NONE',  ( 1.242748055744218760, -82.84189893657375592, -0.1341030727711693959 ) ) ;
#50694=CARTESIAN_POINT ( 'NONE',  ( -1.242284077307689305, -79.59059820921201833, 0.1573562424055395537 ) ) ;
#50715=CARTESIAN_POINT ( 'NONE',  ( 0.03615408296859652648, -82.97326937661254931, 1.249771234374210449 ) ) ;
#50717=DIRECTION ( 'NONE',  ( 1.000000000000000000, 0.000000000000000000, 0.000000000000000000 ) ) ;
#50726=CARTESIAN_POINT ( 'NONE',  ( 0.7681833999686451531, -80.67708333333332860, -0.9995835529977240563 ) ) ;
#50757=ADVANCED_FACE ( 'NONE', ( #19073 ), #5777, .T. ) ;
#50759=CARTESIAN_POINT ( 'NONE',  ( -1.162396057392936166, -80.57013522272643513, 0.4596509125629028580 ) ) ;
#50769=CARTESIAN_POINT ( 'NONE',  ( 1.343749999883000035, -77.90625000011999646, 3.156563468101999814E-09 ) ) ;
#50773=CARTESIAN_POINT ( 'NONE',  ( 1.297392051789066025, -78.14223917446591372, 0.7709785167501194136 ) ) ;
#50788=CARTESIAN_POINT ( 'NONE',  ( -0.4696505103051999974, -83.11672773667999081, -1.267043746813000249 ) ) ;
#50816=CARTESIAN_POINT ( 'NONE',  ( -0.8894962667724020111, -81.53855449988152770, 0.8777776201967760761 ) ) ;
#50847=CARTESIAN_POINT ( 'NONE',  ( 1.623578234368999951, -77.96668092124998850, 0.1125035222880000074 ) ) ;
#50849=CARTESIAN_POINT ( 'NONE',  ( -0.6002759491738461906, -79.18521723992915895, -1.096379978449760095 ) ) ;
#50886=CARTESIAN_POINT ( 'NONE',  ( 0.5818457612699999837, -81.04221672439999224, -1.560998038830999857 ) ) ;
#50887=CARTESIAN_POINT ( 'NONE',  ( 0.9355514851091999429, -78.83229613799998958, 0.9313545561094999092 ) ) ;
#50889=CARTESIAN_POINT ( 'NONE',  ( -1.010492441417754073, -81.31676120415845332, -1.123586503558430039 ) ) ;
#50894=CARTESIAN_POINT ( 'NONE',  ( 0.6298731215011567075, -80.93400402381369929, 1.093396141891215922 ) ) ;
#50896=CARTESIAN_POINT ( 'NONE',  ( 0.4784268551903346767, -81.75636360286721072, -1.154745182890940081 ) ) ;
#50898=DIRECTION ( 'NONE',  ( -1.000000000000000000, 0.000000000000000000, 0.000000000000000000 ) ) ;
#50912=EDGE_CURVE ( 'NONE', #53705, #23434, #40954, .T. ) ;
#50916=CARTESIAN_POINT ( 'NONE',  ( -1.250000000000000000, -81.49999999999998579, 0.000000000000000000 ) ) ;
#50922=CARTESIAN_POINT ( 'NONE',  ( 1.249711497515000103, -79.84934566756000152, -0.7711480544179000196 ) ) ;
#50936=CARTESIAN_POINT ( 'NONE',  ( -1.250000000000000000, -80.59999999999999432, 0.000000000000000000 ) ) ;
#50978=CARTESIAN_POINT ( 'NONE',  ( 0.9194760088113610452, -82.79137680920143794, -0.8462349433019908940 ) ) ;
#51004=CARTESIAN_POINT ( 'NONE',  ( 0.3908001115028792993, -82.94971160634423768, 1.187542448887068725 ) ) ;
#51011=CARTESIAN_POINT ( 'NONE',  ( -0.9184750406504611497, -79.77639907747951042, 1.199933283862223421 ) ) ;
#51029=CARTESIAN_POINT ( 'NONE',  ( -0.5544740949720999845, -82.29082582312000227, 1.570928860995999932 ) ) ;
#51049=CARTESIAN_POINT ( 'NONE',  ( -1.229694712338595508, -80.58624861086376256, 0.2234822223714939271 ) ) ;
#51065=CARTESIAN_POINT ( 'NONE',  ( 1.523426795032935654, -78.58841195298964521, -0.2098259862101924111 ) ) ;
#51066=ADVANCED_FACE ( 'NONE', ( #2172 ), #8025, .T. ) ;
#51070=EDGE_CURVE ( 'NONE', #41164, #22489, #3615, .T. ) ;
#51076=CARTESIAN_POINT ( 'NONE',  ( -10.14999999999999858, -87.09999999999999432, 0.000000000000000000 ) ) ;
#51080=CARTESIAN_POINT ( 'NONE',  ( -1.281643947269487605, -81.20542284418931445, 0.8013805647649642205 ) ) ;
#51090=CARTESIAN_POINT ( 'NONE',  ( -0.4696505103051999974, -82.67677767037399406, -1.267043746813000249 ) ) ;
#51099=CARTESIAN_POINT ( 'NONE',  ( -0.5328894382976427924, -79.19002943946934181, -1.131072528211912953 ) ) ;
#51105=CONICAL_SURFACE ( 'NONE', #25612, 10.09999999997999964, 0.7853981633972997312 ) ;
#51114=CARTESIAN_POINT ( 'NONE',  ( -0.8488654463164000408, -78.64882235081999795, -0.9950929470245999386 ) ) ;
#51142=CARTESIAN_POINT ( 'NONE',  ( 1.328072050606999843, -78.58978245110000671, -0.9406846882429998891 ) ) ;
#51179=CARTESIAN_POINT ( 'NONE',  ( -1.387963714323000142, -79.78297531344000504, 0.9213108730841000904 ) ) ;
#51182=CARTESIAN_POINT ( 'NONE',  ( 1.411403051189575431, -81.52931625501098267, 0.5428011461610074972 ) ) ;
#51184=CARTESIAN_POINT ( 'NONE',  ( 0.000000000000000000, -77.59999999938000315, 0.000000000000000000 ) ) ;
#51186=CARTESIAN_POINT ( 'NONE',  ( 0.9661093279367058972, -79.79552230973584415, -0.7934550806089618602 ) ) ;
#51188=EDGE_CURVE ( 'NONE', #54320, #31102, #51980, .T. ) ;
#51190=CARTESIAN_POINT ( 'NONE',  ( -1.032281996597182339, -81.64822189729572699, -0.7051746695584234503 ) ) ;
#51211=CARTESIAN_POINT ( 'NONE',  ( -0.7681833999686477066, -81.42708333333332860, 0.9995835529977223910 ) ) ;
#51216=CARTESIAN_POINT ( 'NONE',  ( 0.9995835529977233902, -79.80208333333334281, 0.7681833999686461523 ) ) ;
#51218=CARTESIAN_POINT ( 'NONE',  ( -1.376297233339999870, -80.16529921676999493, 0.7875294559552000750 ) ) ;
#51237=CARTESIAN_POINT ( 'NONE',  ( 1.182180303898404006, -78.37658685848882101, 0.4056014702486911983 ) ) ;
#51249=CARTESIAN_POINT ( 'NONE',  ( -0.08911090410158063746, -81.98124066240951890, 1.246717735211338107 ) ) ;
#51253=DIRECTION ( 'NONE',  ( 0.000000000000000000, 0.000000000000000000, -1.000000000000000000 ) ) ;
#51270=CIRCLE ( 'NONE', #35208, 9.000000000000000000 ) ;
#51274=CARTESIAN_POINT ( 'NONE',  ( 0.2515381494466178980, -82.74157260121474167, -1.224160487734374358 ) ) ;
#51279=CARTESIAN_POINT ( 'NONE',  ( -0.8773474274045136578, -78.82551938010156789, -1.226174542836929726 ) ) ;
#51281=DIRECTION ( 'NONE',  ( 0.000000000000000000, -1.000000000000000000, 0.000000000000000000 ) ) ;
#51297=CARTESIAN_POINT ( 'NONE',  ( 0.4743252877779617904, -82.94407894522871061, 1.156479017802467757 ) ) ;
#51302=LINE ( 'NONE', #37701, #5444 ) ;
#51320=CARTESIAN_POINT ( 'NONE',  ( -1.519662023741000123, -82.92241797422099125, -0.6825586799200999977 ) ) ;
#51325=CARTESIAN_POINT ( 'NONE',  ( -0.2201363562291999698, -79.36327907013999550, -1.483758735329000045 ) ) ;
#51337=CARTESIAN_POINT ( 'NONE',  ( 0.6909066256383181726, -80.42853791983925760, 1.041600136228693518 ) ) ;
#51338=LINE ( 'NONE', #56052, #42708 ) ;
#51352=CARTESIAN_POINT ( 'NONE',  ( 0.8454482194665522421, -79.17736002063097089, 1.250557891722181347 ) ) ;
#51380=CARTESIAN_POINT ( 'NONE',  ( 0.6295237254636258939, -82.16666666666665719, -1.092232985442821658 ) ) ;
#51399=CARTESIAN_POINT ( 'NONE',  ( -0.1211015312307294062, -81.48306870518814549, 1.244369522078131451 ) ) ;
#51400=EDGE_CURVE ( 'NONE', #20349, #36091, #43051, .T. ) ;
#51405=FACE_OUTER_BOUND ( 'NONE', #32182, .T. ) ;
#51407=CARTESIAN_POINT ( 'NONE',  ( -1.250000000000000000, -80.49999999999998579, 0.000000000000000000 ) ) ;
#51433=CARTESIAN_POINT ( 'NONE',  ( -0.9465222407332000154, -81.55663953507000485, -0.8164530897714000757 ) ) ;
#51434=CARTESIAN_POINT ( 'NONE',  ( -0.1732310466989999687, -77.71390310378998834, 1.530487294790999986 ) ) ;
#51435=ADVANCED_FACE ( 'NONE', ( #2319 ), #33586, .F. ) ;
#51443=CARTESIAN_POINT ( 'NONE',  ( -0.3234604031741999952, -79.72023290324000300, 1.671883997359000062 ) ) ;
#51468=CARTESIAN_POINT ( 'NONE',  ( -0.07152028281723200875, -79.97993409046794966, 1.247844452081509292 ) ) ;
#51473=CARTESIAN_POINT ( 'NONE',  ( 1.431169160529000006, -78.21216375143998789, 0.09917081181617999619 ) ) ;
#51475=CARTESIAN_POINT ( 'NONE',  ( -1.454013506048745130, -81.77223631312656948, -0.4159240082623796297 ) ) ;
#51476=CARTESIAN_POINT ( 'NONE',  ( -0.2580402550692753594, -83.23804571606062552, 1.489083542988291153 ) ) ;
#51477=CARTESIAN_POINT ( 'NONE',  ( 0.4990820023277747763, -79.75804326553362955, -1.145820899119790681 ) ) ;
#51478=CIRCLE ( 'NONE', #32595, 10.14999999999999858 ) ;
#51481=CARTESIAN_POINT ( 'NONE',  ( -1.144794046686379296, -81.63306042909437110, -0.5017307455195174626 ) ) ;
#51482=FILL_AREA_STYLE_COLOUR ( '', #12406 ) ;
#51484=CARTESIAN_POINT ( 'NONE',  ( -1.135826688880000157, -81.40663953506998496, -0.9797437077257000748 ) ) ;
#51509=CARTESIAN_POINT ( 'NONE',  ( -1.563706488702000019, -81.30232256240998368, -0.6734635195847999967 ) ) ;
#51510=CARTESIAN_POINT ( 'NONE',  ( 1.250000000000000000, -80.25000000000000000, 0.000000000000000000 ) ) ;
#51511=CARTESIAN_POINT ( 'NONE',  ( -1.387074871800343834, -79.71753748822699492, 0.5993129225438764696 ) ) ;
#51529=CARTESIAN_POINT ( 'NONE',  ( 1.185568982899148693, -78.37591526493211802, 0.3956926376703175929 ) ) ;
#51564=CARTESIAN_POINT ( 'NONE',  ( 0.2560571373808674389, -82.74185738613888930, -1.223228159499044398 ) ) ;
#51569=CARTESIAN_POINT ( 'NONE',  ( 0.2655774789948861514, -78.38858963195251306, -1.510445311185437456 ) ) ;
#51589=CARTESIAN_POINT ( 'NONE',  ( 1.022162451771789549, -82.89907212072580478, 0.7192351975817576903 ) ) ;
#51596=CARTESIAN_POINT ( 'NONE',  ( -0.1834469635243000107, -79.21327907014000402, -1.236465612773999911 ) ) ;
#51614=CARTESIAN_POINT ( 'NONE',  ( 1.431241028886999889, -81.59607445691000294, -0.8524881072380000591 ) ) ;
#51621=ORIENTED_EDGE ( 'NONE', *, *, #10642, .T. ) ;
#51625=CARTESIAN_POINT ( 'NONE',  ( -1.250000000000000000, -80.59999999999999432, 0.000000000000000000 ) ) ;
#51633=CARTESIAN_POINT ( 'NONE',  ( 0.6030484120316327301, -80.43496411464462881, 1.095119744681182228 ) ) ;
#51651=CARTESIAN_POINT ( 'NONE',  ( -0.1181554223150161204, -79.23090075405382038, 1.505089927673818773 ) ) ;
#51666=CARTESIAN_POINT ( 'NONE',  ( -0.7953408400917133525, -80.83092108792313013, -1.285395336168587033 ) ) ;
#51669=FACE_OUTER_BOUND ( 'NONE', #17485, .T. ) ;
#51697=CARTESIAN_POINT ( 'NONE',  ( 0.05681272259054000184, -79.27140911722999306, -1.352556977364000046 ) ) ;
#51699=CARTESIAN_POINT ( 'NONE',  ( 1.250000000000000000, -78.25000000000000000, 0.000000000000000000 ) ) ;
#51724=CARTESIAN_POINT ( 'NONE',  ( 1.623578234368999951, -78.14432989285998588, 0.1125035222880000074 ) ) ;
#51733=CARTESIAN_POINT ( 'NONE',  ( 0.6229729438976999711, -81.23621153953999396, 1.458184003450999855 ) ) ;
#51752=CARTESIAN_POINT ( 'NONE',  ( -0.8459884596345884633, -79.42721677660425428, -1.250127555251149047 ) ) ;
#51758=CARTESIAN_POINT ( 'NONE',  ( -0.9200625262326408427, -80.04125824231630304, 0.8460283513402829803 ) ) ;
#51765=CARTESIAN_POINT ( 'NONE',  ( 0.3895721858179450048, -82.99511992827669360, -1.461044772055308361 ) ) ;
#51766=CARTESIAN_POINT ( 'NONE',  ( -1.124179317452199900, -79.63649961456538051, -0.5465545694080121697 ) ) ;
#51795=CARTESIAN_POINT ( 'NONE',  ( -0.1636246173744726473, -79.88541666666664298, 1.249999999999999112 ) ) ;
#51797=CARTESIAN_POINT ( 'NONE',  ( 1.511505244404999893, -80.48109529231999204, 0.4793209935110999687 ) ) ;
#51817=CARTESIAN_POINT ( 'NONE',  ( 1.250000728980784181, -78.35225028680585524, 0.03536658250550711591 ) ) ;
#51840=DIRECTION ( 'NONE',  ( -1.000000000000000000, 0.000000000000000000, 0.000000000000000000 ) ) ;
#51853=CARTESIAN_POINT ( 'NONE',  ( 0.000000000000000000, -92.39999999999999147, 0.000000000000000000 ) ) ;
#51856=CARTESIAN_POINT ( 'NONE',  ( 0.9293276542485822134, -78.57344452540336022, 1.219933349864354977 ) ) ;
#51874=CARTESIAN_POINT ( 'NONE',  ( -0.08551465511880061710, -82.98103542870875060, 1.246841896993040155 ) ) ;
#51895=B_SPLINE_CURVE_WITH_KNOTS ( 'NONE', 3,
 ( #11150, #33553, #6701, #24120, #29124, #20571, #47170, #29412, #37698, #6988, #34416, #6405, #52164, #24712, #42138, #24993, #43014, #38856 ),
 .UNSPECIFIED., .F., .F.,
 ( 4, 2, 2, 2, 2, 2, 2, 2, 4 ),
 ( 0.000000000000000000, 0.1249999999999999722, 0.2500000000000000000, 0.3750000000000000000, 0.5000000000000001110, 0.6250000000000001110, 0.7500000000000000000, 0.8750000000000000000, 1.000000000000000000 ),
 .UNSPECIFIED. ) ;
#51914=CARTESIAN_POINT ( 'NONE',  ( -0.8719868943402252492, -80.53708738304344195, 0.8952310760180179905 ) ) ;
#51946=CARTESIAN_POINT ( 'NONE',  ( -0.06677702975030901100, -80.87140776427570188, -1.508501679119423677 ) ) ;
#51957=ORIENTED_EDGE ( 'NONE', *, *, #25410, .F. ) ;
#51973=CARTESIAN_POINT ( 'NONE',  ( 0.8462078165385277240, -81.41624116930810828, 0.9198965729622936571 ) ) ;
#51976=FACE_OUTER_BOUND ( 'NONE', #5844, .T. ) ;
#51980=CIRCLE ( 'NONE', #43499, 1.750000000000000000 ) ;
#51985=ADVANCED_FACE ( 'NONE', ( #37070 ), #51105, .T. ) ;
#51995=CARTESIAN_POINT ( 'NONE',  ( -1.499999999971000086, -77.75000000002998490, -1.761798912373000190E-09 ) ) ;
#51999=DIRECTION ( 'NONE',  ( 0.7071067811865474617, -0.7071067811865474617, -1.236215424745081016E-09 ) ) ;
#52000=( GEOMETRIC_REPRESENTATION_CONTEXT ( 3 ) GLOBAL_UNCERTAINTY_ASSIGNED_CONTEXT ( ( #11845 ) ) GLOBAL_UNIT_ASSIGNED_CONTEXT ( ( #2180, #46186, #1027 ) ) REPRESENTATION_CONTEXT ( 'NONE', 'WORKASPACE' ) );
#52010=CARTESIAN_POINT ( 'NONE',  ( 1.621809933883000099, -78.64546402086999421, 0.1356303529659999840 ) ) ;
#52016=CARTESIAN_POINT ( 'NONE',  ( -0.8956573524961000121, -81.41095650773000614, -1.447939571232000011 ) ) ;
#52018=CARTESIAN_POINT ( 'NONE',  ( 0.3786699527928999442, -79.97286976367999500, -1.660248773968999947 ) ) ;
#52040=LINE ( 'NONE', #29858, #57179 ) ;
#52042=LINE ( 'NONE', #34581, #12599 ) ;
#52044=CARTESIAN_POINT ( 'NONE',  ( -0.3763322838831557604, -79.99938371673916038, 1.195031458938746738 ) ) ;
#52050=LINE ( 'NONE', #39034, #55635 ) ;
#52052=CARTESIAN_POINT ( 'NONE',  ( 1.491775814946131984, -83.08621709869576932, -0.2501303660045399169 ) ) ;
#52053=CARTESIAN_POINT ( 'NONE',  ( 0.4182184111412154404, -79.75227781930720994, -1.179636507925768907 ) ) ;
#52063=VECTOR ( 'NONE', #5436, 1000.000000000000000 ) ;
#52081=CARTESIAN_POINT ( 'NONE',  ( -0.3271848554491046945, -79.89583333333330017, 1.217465845835393301 ) ) ;
#52083=CARTESIAN_POINT ( 'NONE',  ( 1.449190734180999973, -79.97597904509999012, -0.8942388842271000726 ) ) ;
#52097=EDGE_CURVE ( 'NONE', #12955, #46203, #24384, .T. ) ;
#52101=CARTESIAN_POINT ( 'NONE',  ( 1.133628739905723437, -78.38499154607053754, 0.5281210143588952466 ) ) ;
#52114=CARTESIAN_POINT ( 'NONE',  ( 0.4422131289978999957, -78.97643549037999833, -1.603741477255999914 ) ) ;
#52119=DIRECTION ( 'NONE',  ( 0.000000000000000000, -1.000000000000000000, -1.378526922243000102E-14 ) ) ;
#52120=CARTESIAN_POINT ( 'NONE',  ( -1.135826688880000157, -81.30663953507000485, -0.9797437077257000748 ) ) ;
#52137=CARTESIAN_POINT ( 'NONE',  ( 0.2456986548642498824, -82.74120455909647376, -1.225335228240030050 ) ) ;
#52140=CARTESIAN_POINT ( 'NONE',  ( -0.8256138858706347783, -79.53279254742548687, 0.9417001439504392168 ) ) ;
#52141=CARTESIAN_POINT ( 'NONE',  ( 0.6432483788054168539, -78.59024951571676354, 1.390064027832063731 ) ) ;
#52149=CARTESIAN_POINT ( 'NONE',  ( 0.000000000000000000, -76.75499999999999545, 0.000000000000000000 ) ) ;
#52164=CARTESIAN_POINT ( 'NONE',  ( 0.7681833999686413783, -80.32291666666668561, 0.9995835529977274980 ) ) ;
#52198=CARTESIAN_POINT ( 'NONE',  ( -0.1244589946783580814, -80.48333614422827509, 1.244172789713544613 ) ) ;
#52208=ADVANCED_FACE ( 'NONE', ( #23616 ), #17920, .F. ) ;
#52218=DIRECTION ( 'NONE',  ( 0.000000000000000000, 0.000000000000000000, 1.000000000000000000 ) ) ;
#52226=CARTESIAN_POINT ( 'NONE',  ( 0.4626184419780025592, -79.89972753181358200, -1.439301428628166679 ) ) ;
#52233=EDGE_CURVE ( 'NONE', #13108, #35472, #41679, .T. ) ;
#52236=CARTESIAN_POINT ( 'NONE',  ( 0.4644997175289000135, -82.99273121958398747, 1.393065715888999856 ) ) ;
#52253=CARTESIAN_POINT ( 'NONE',  ( 0.4565975880176471602, -81.44548833070547289, 1.163485847307625942 ) ) ;
#52254=CARTESIAN_POINT ( 'NONE',  ( 1.356773869401999955, -79.53033845299998461, -0.9668579442890000708 ) ) ;
#52262=CARTESIAN_POINT ( 'NONE',  ( -1.250000000000000000, -78.50000000000000000, 0.000000000000000000 ) ) ;
#52285=CARTESIAN_POINT ( 'NONE',  ( 1.217465845835394855, -83.22916666666665719, -0.3271848554490981997 ) ) ;
#52289=DIRECTION ( 'NONE',  ( 0.000000000000000000, 1.000000000000000000, 0.000000000000000000 ) ) ;
#52290=CARTESIAN_POINT ( 'NONE',  ( -1.560595261880000084, -77.80670572008999386, 0.4619550309703999713 ) ) ;
#52302=CARTESIAN_POINT ( 'NONE',  ( -1.623947472758999977, -83.30573296103600001, 0.5113958356693000251 ) ) ;
#52304=CARTESIAN_POINT ( 'NONE',  ( 1.349451115848000038, -80.09934566756000152, -0.8326934693224998796 ) ) ;
#52307=DIRECTION ( 'NONE',  ( 0.000000000000000000, -1.000000000000000000, 0.000000000000000000 ) ) ;
#52308=CARTESIAN_POINT ( 'NONE',  ( 0.5269479332349999989, -83.06056507816398948, 1.580352090963000000 ) ) ;
#52317=CARTESIAN_POINT ( 'NONE',  ( 0.000000000000000000, -87.20000000000000284, 0.000000000000000000 ) ) ;
#52331=CARTESIAN_POINT ( 'NONE',  ( -1.178384143479807022, -80.07328496558248787, 0.4165272804027306819 ) ) ;
#52337=CARTESIAN_POINT ( 'NONE',  ( -1.144681710389366502, -82.79268177178988708, 0.9866455203037115540 ) ) ;
#52339=CARTESIAN_POINT ( 'NONE',  ( -0.9895445474833923782, -79.65312179139979776, -0.7673432424604474944 ) ) ;
#52349=B_SPLINE_CURVE_WITH_KNOTS ( 'NONE', 3,
 ( #33733, #20465, #5706, #42901, #14852, #28424, #19883, #24308, #42322, #50894, #33442, #6295, #55897, #24598, #41728, #55601 ),
 .UNSPECIFIED., .F., .F.,
 ( 4, 2, 1, 2, 1, 2, 2, 2, 4 ),
 ( 0.000000000000000000, 0.1249999999999998890, 0.2499999999999998335, 0.3749999999999998335, 0.4999999999999998890, 0.6249999999999998890, 0.7499999999999998890, 0.8749999999999998890, 1.000000000000000000 ),
 .UNSPECIFIED. ) ;
#52356=VECTOR ( 'NONE', #18467, 1000.000000000000000 ) ;
#52366=CARTESIAN_POINT ( 'NONE',  ( -0.9995835529977281642, -79.94791666666664298, 0.7681833999686391579 ) ) ;
#52389=CARTESIAN_POINT ( 'NONE',  ( 1.062401685567854859, -78.39434672560830109, 0.6596734765841812953 ) ) ;
#52401=CARTESIAN_POINT ( 'NONE',  ( 1.148655909719971113, -81.88235501812725659, 0.4929135997214548759 ) ) ;
#52408=CARTESIAN_POINT ( 'NONE',  ( -1.134730520616228144, -81.33997286840332208, -0.9788030900385257249 ) ) ;
#52423=CARTESIAN_POINT ( 'NONE',  ( 0.2465309757704703397, -82.74125708629129861, -1.225171777312197952 ) ) ;
#52426=CARTESIAN_POINT ( 'NONE',  ( 0.5606705885283177482, -79.43831444490541571, 1.120598156864235584 ) ) ;
#52427=CARTESIAN_POINT ( 'NONE',  ( 0.5698392209909881601, -79.09439922511995746, 1.421990052734795729 ) ) ;
#52433=DIRECTION ( 'NONE',  ( -1.000000000000000000, 0.000000000000000000, 0.000000000000000000 ) ) ;
#52482=ADVANCED_FACE ( 'NONE', ( #30442 ), #34580, .T. ) ;
#52483=CARTESIAN_POINT ( 'NONE',  ( 0.4761608617425592271, -80.44399108949784249, 1.155693504187701448 ) ) ;
#52488=EDGE_LOOP ( 'NONE', ( #47068, #46474, #55982, #13269 ) ) ;
#52502=CARTESIAN_POINT ( 'NONE',  ( -0.3271848554491046945, -83.39583333333332860, 1.217465845835393301 ) ) ;
#52510=CARTESIAN_POINT ( 'NONE',  ( 1.081520234856472307, -80.43617599348539215, -1.105279526349218111 ) ) ;
#52519=CARTESIAN_POINT ( 'NONE',  ( 0.5015714934020000237, -83.05604790835199935, 1.504246450876000063 ) ) ;
#52535=EDGE_CURVE ( 'NONE', #48909, #2755, #31050, .T. ) ;
#52538=CARTESIAN_POINT ( 'NONE',  ( 1.640574411872000038, -79.53428134424000007, 0.2893137654249999802 ) ) ;
#52552=CARTESIAN_POINT ( 'NONE',  ( 1.376276113774000054, -77.87323392310999282, -0.3553535975348000031 ) ) ;
#52588=CARTESIAN_POINT ( 'NONE',  ( -1.553390134080000040, -82.86361845526398895, -0.6977077157647000316 ) ) ;
#52589=CARTESIAN_POINT ( 'NONE',  ( -0.8477325451633000997, -79.46775351646000729, -1.148851298854000058 ) ) ;
#52593=CARTESIAN_POINT ( 'NONE',  ( 1.431241028886999889, -81.41842548529999135, -0.8524881072380000591 ) ) ;
#52607=CARTESIAN_POINT ( 'NONE',  ( -0.5544740949720999845, -82.23160949924999841, 1.570928860995999932 ) ) ;
#52616=CARTESIAN_POINT ( 'NONE',  ( -0.8849959507268040371, -80.03812507728116543, 0.8823318837302972506 ) ) ;
#52622=CARTESIAN_POINT ( 'NONE',  ( -0.6952495977537009875, -82.76231604831681921, 1.343821088991839607 ) ) ;
#52623=CARTESIAN_POINT ( 'NONE',  ( 0.8926277122277624931, -79.78871733315683912, -0.8747132943431308316 ) ) ;
#52652=CARTESIAN_POINT ( 'NONE',  ( -0.7681833999686432657, -81.07291666666668561, -0.9995835529977258327 ) ) ;
#52683=CARTESIAN_POINT ( 'NONE',  ( 1.153057336080759665, -81.88161975503362555, 0.4825267112434911687 ) ) ;
#52684=CARTESIAN_POINT ( 'NONE',  ( 1.162132110709999999, -79.14348019970999815, 1.190372713651999925 ) ) ;
#52694=CARTESIAN_POINT ( 'NONE',  ( 0.3271848554490964789, -81.85416666666667140, 1.217465845835395521 ) ) ;
#52696=CARTESIAN_POINT ( 'NONE',  ( -1.135826688880000157, -81.30663953507000485, -0.9797437077257000748 ) ) ;
#52700=ORIENTED_EDGE ( 'NONE', *, *, #27992, .F. ) ;
#52704=ORIENTED_EDGE ( 'NONE', *, *, #42399, .T. ) ;
#52709=EDGE_CURVE ( 'NONE', #1475, #56551, #22611, .T. ) ;
#52713=ORIENTED_EDGE ( 'NONE', *, *, #9775, .T. ) ;
#52755=CARTESIAN_POINT ( 'NONE',  ( 0.000000000000000000, -76.75499999999999545, 0.000000000000000000 ) ) ;
#52794=CARTESIAN_POINT ( 'NONE',  ( 0.01767233353438701221, -80.37544597895652032, -1.546831932022704414 ) ) ;
#52805=CARTESIAN_POINT ( 'NONE',  ( -1.167634245779999969, -83.18220886491398858, -0.6204341648412000643 ) ) ;
#52823=CARTESIAN_POINT ( 'NONE',  ( -1.570423240223999928, -80.85668197030999238, -0.5559045111934000083 ) ) ;
#52831=CARTESIAN_POINT ( 'NONE',  ( 0.9995835529977233902, -78.30208333333332860, 0.7681833999686461523 ) ) ;
#52857=CARTESIAN_POINT ( 'NONE',  ( 0.3271848554491016414, -83.14583333333332860, -1.217465845835393967 ) ) ;
#52868=CARTESIAN_POINT ( 'NONE',  ( -1.225907436145275087, -83.08370455176279279, 0.2589396600793889558 ) ) ;
#52874=CARTESIAN_POINT ( 'NONE',  ( -1.526555281555000088, -80.41514174310999863, -0.4289821568622999570 ) ) ;
#52878=CARTESIAN_POINT ( 'NONE',  ( -1.458706046781999888, -81.67106234573999757, 0.8046341008317999810 ) ) ;
#52896=DIRECTION ( 'NONE',  ( 0.000000000000000000, -1.000000000000000000, 0.000000000000000000 ) ) ;
#52906=CARTESIAN_POINT ( 'NONE',  ( -1.008405205759953738, -82.78255986396547428, 1.125655370664245591 ) ) ;
#52924=B_SPLINE_CURVE_WITH_KNOTS ( 'NONE', 3,
 ( #18538, #41842, #9971, #14966, #41257, #9674 ),
 .UNSPECIFIED., .F., .F.,
 ( 4, 2, 4 ),
 ( 0.7142789241156584090, 0.8571394620578292045, 1.000000000000000000 ),
 .UNSPECIFIED. ) ;
#52939=CARTESIAN_POINT ( 'NONE',  ( 0.1636246173744697330, -81.13541666666665719, -1.249999999999999778 ) ) ;
#52941=ORIENTED_EDGE ( 'NONE', *, *, #21040, .T. ) ;
#52963=CARTESIAN_POINT ( 'NONE',  ( 10.14999999998000035, -87.10000000002298748, -2.878934427392999978E-10 ) ) ;
#52972=CARTESIAN_POINT ( 'NONE',  ( 0.8430560329671303865, -81.91662283780821951, 0.9225686058375374143 ) ) ;
#52989=CARTESIAN_POINT ( 'NONE',  ( 1.250000000000000000, -83.49999999999998579, 0.000000000000000000 ) ) ;
#53071=CARTESIAN_POINT ( 'NONE',  ( -1.413836290689950648, -77.82099477392877418, 0.5308369793427527572 ) ) ;
#53082=CARTESIAN_POINT ( 'NONE',  ( 1.501221344685673476, -80.09017822003303877, -0.1728645978363567981 ) ) ;
#53093=CARTESIAN_POINT ( 'NONE',  ( 1.318896022268000179, -82.92957200447399657, 0.6457249424517998992 ) ) ;
#53097=CARTESIAN_POINT ( 'NONE',  ( -0.9995835529977249445, -82.05208333333328596, -0.7681833999686439318 ) ) ;
#53133=CARTESIAN_POINT ( 'NONE',  ( 0.4817127218574778769, -80.25663193929872818, -1.153353357640556798 ) ) ;
#53147=AXIS2_PLACEMENT_3D ( 'NONE', #9378, #22952, #50124 ) ;
#53151=CARTESIAN_POINT ( 'NONE',  ( 9.000000000000000000, -91.89999999999999147, 2.447153590879000268E-12 ) ) ;
#53155=DIRECTION ( 'NONE',  ( -1.000000000000000000, 0.000000000000000000, 0.000000000000000000 ) ) ;
#53158=CARTESIAN_POINT ( 'NONE',  ( 1.517511648408000013, -82.04254865883000036, -0.7726417995267998995 ) ) ;
#53160=CARTESIAN_POINT ( 'NONE',  ( 0.6650966107743999656, -80.79425450742999715, 1.309234371339000225 ) ) ;
#53164=CARTESIAN_POINT ( 'NONE',  ( -1.596536837631000072, -81.73422156085000267, -0.4757406268331999533 ) ) ;
#53175=EDGE_CURVE ( 'NONE', #12675, #24608, #19906, .T. ) ;
#53185=CARTESIAN_POINT ( 'NONE',  ( 1.152392759189329263, -79.88190785368323077, 0.4838130652222127903 ) ) ;
#53188=B_SPLINE_SURFACE_WITH_KNOTS ( 'NONE', 3, 3, ( 
 ( #33980, #2997, #52302, #16289, #47888, #6838, #25423, #43735, #43437, #52588, #2422, #30126, #35127, #43156, #12426, #20995, #24849, #48175, #7706, #3567, #30418, #48451, #53158, #39000, #44015, #57008, #21571, #29261, #42864, #20425, #25708, #2713, #52016, #20709, #16571 ),
 ( #34556, #3287, #12138, #4738, #31572, #22442, #45189, #48737, #4440, #13285, #18321, #9460, #49620, #9167, #27445, #27148, #53445, #26283, #36603, #40456, #632, #13580, #23028, #18024, #22145, #44591, #3852, #22737, #57873, #30985, #48, #44890, #30701, #49320, #53748 ),
 ( #40747, #45481, #8281, #8573, #26861, #41042, #35415, #58166, #8868, #21850, #13876, #49025, #35719, #36312, #342, #39859, #31871, #54337, #49912, #36016, #54043, #5026, #18614, #12707, #44297, #17428, #17732, #12989, #26559, #4146, #40153, #31277, #37184, #18899, #20069 ),
 ( #55492, #28905, #24196, #1779, #1199, #14741, #46950, #6476, #50788, #24486, #41916, #5317, #41621, #23325, #42212, #50199, #55198, #42501, #15340, #54626, #33034, #50492, #41332, #5594, #2071, #32740, #32448, #916, #19773, #10332, #10047, #14162, #46656, #33333, #19192 ) ),
 .UNSPECIFIED., .F., .F., .F.,
 ( 4, 4 ),
 ( 4, 1, 1, 1, 1, 1, 1, 1, 1, 1, 1, 1, 1, 1, 1, 1, 1, 1, 1, 1, 1, 1, 1, 1, 1, 1, 1, 1, 1, 1, 1, 1, 4 ),
 ( -0.1331668876848000060, 1.133166887685000068 ),
 ( -0.02000000000000000042, 0.01250000000000000069, 0.04499999999999999833, 0.07749999999999999944, 0.1100000000000000006, 0.1424999999999999878, 0.1749999999999999889, 0.2074999999999999900, 0.2399999999999999911, 0.2725000000000000200, 0.3049999999999999933, 0.3375000000000000222, 0.3699999999999999956, 0.4025000000000000244, 0.4349999999999999978, 0.4675000000000000266, 0.5000000000000000000, 0.5324999999999999734, 0.5649999999999999467, 0.5975000000000000311, 0.6300000000000000044, 0.6624999999999999778, 0.6949999999999999512, 0.7275000000000000355, 0.7600000000000000089, 0.7924999999999999822, 0.8249999999999999556, 0.8575000000000000400, 0.8900000000000000133, 0.9224999999999999867, 0.9549999999999999600, 0.9875000000000000444, 1.020000000000000018 ),
 .UNSPECIFIED. ) ;
#53203=EDGE_LOOP ( 'NONE', ( #8803, #23308, #13699, #5220 ) ) ;
#53245=DIRECTION ( 'NONE',  ( -1.040691342546000016E-11, 1.000000000000000000, 2.038009761064000191E-09 ) ) ;
#53254=CARTESIAN_POINT ( 'NONE',  ( 0.07936805562503999878, -79.52232578389998707, -1.463935019116999747 ) ) ;
#53257=CARTESIAN_POINT ( 'NONE',  ( -1.143843590492619189, -82.69330820015007077, 0.9859688983279260022 ) ) ;
#53287=CARTESIAN_POINT ( 'NONE',  ( -1.302408693230432402, -77.79201247581434586, -0.7600488025388738578 ) ) ;
#53344=DIRECTION ( 'NONE',  ( 1.000000000000000000, 0.000000000000000000, 0.000000000000000000 ) ) ;
#53365=CARTESIAN_POINT ( 'NONE',  ( 1.498260933585416455, -80.11042203568169384, 0.2089178497027620873 ) ) ;
#53375=CARTESIAN_POINT ( 'NONE',  ( -1.295013057735999951, -81.60307101349998504, -0.3858917059242000236 ) ) ;
#53409=CARTESIAN_POINT ( 'NONE',  ( 0.3914697351672000170, -79.41551968470000133, -1.482475952910999872 ) ) ;
#53415=CARTESIAN_POINT ( 'NONE',  ( 0.004398891372963634194, -80.22583377693190698, -1.249663113230017997 ) ) ;
#53427=ORIENTED_EDGE ( 'NONE', *, *, #48627, .F. ) ;
#53441=CARTESIAN_POINT ( 'NONE',  ( -1.155567653434479647, -83.06898091192337574, 0.4764477841603429464 ) ) ;
#53444=ORIENTED_EDGE ( 'NONE', *, *, #5485, .F. ) ;
#53445=CARTESIAN_POINT ( 'NONE',  ( -0.6483708932059000229, -82.48482063826099875, -1.447070110047999902 ) ) ;
#53446=CARTESIAN_POINT ( 'NONE',  ( -0.4789091134304000463, -81.55216508874998738, -1.232458658897999992 ) ) ;
#53458=CARTESIAN_POINT ( 'NONE',  ( -1.140226658635644874, -79.53775969004662727, -0.5918896188630813349 ) ) ;
#53462=CARTESIAN_POINT ( 'NONE',  ( 1.571434226476000173, -83.05267929568199747, -0.5530452149683998675 ) ) ;
#53473=CARTESIAN_POINT ( 'NONE',  ( 0.1339442445619486721, -79.96711704085768702, 1.244995031654752893 ) ) ;
#53478=FACE_OUTER_BOUND ( 'NONE', #32603, .T. ) ;
#53480=CARTESIAN_POINT ( 'NONE',  ( -0.3340625910779762009, -81.45658993897731648, -1.473584088927320623 ) ) ;
#53492=ORIENTED_EDGE ( 'NONE', *, *, #44468, .F. ) ;
#53498=CARTESIAN_POINT ( 'NONE',  ( -0.7617914920845411109, -79.52766219886571264, 0.9938330950829512567 ) ) ;
#53513=CARTESIAN_POINT ( 'NONE',  ( 0.6295237254636258939, -78.16666666666665719, -1.092232985442821658 ) ) ;
#53545=EDGE_CURVE ( 'NONE', #37205, #46203, #32645, .T. ) ;
#53550=CARTESIAN_POINT ( 'NONE',  ( 1.221746786348032687, -81.86707072010140962, 0.2639991584434943084 ) ) ;
#53551=CARTESIAN_POINT ( 'NONE',  ( -0.1770758199222000062, -77.71431990869999140, 1.564455666405000001 ) ) ;
#53553=CARTESIAN_POINT ( 'NONE',  ( -0.6947239650216572304, -82.66294319288569170, 1.342880243175269550 ) ) ;
#53559=CARTESIAN_POINT ( 'NONE',  ( 0.6808670543330055391, -81.77126629245766765, -1.049018940644094400 ) ) ;
#53562=CARTESIAN_POINT ( 'NONE',  ( -0.1636246173744673738, -80.11458333333332860, -1.249999999999999778 ) ) ;
#53583=EDGE_CURVE ( 'NONE', #26401, #15817, #19390, .T. ) ;
#53621=CARTESIAN_POINT ( 'NONE',  ( -0.9995835529977281642, -82.44791666666662877, 0.7681833999686391579 ) ) ;
#53629=CYLINDRICAL_SURFACE ( 'NONE', #49012, 10.14999999999999858 ) ;
#53631=CYLINDRICAL_SURFACE ( 'NONE', #17046, 3.000000000000000000 ) ;
#53641=ORIENTED_EDGE ( 'NONE', *, *, #26429, .T. ) ;
#53667=CARTESIAN_POINT ( 'NONE',  ( 1.249290605349439254, -81.05175946334958326, -0.8518751653260581147 ) ) ;
#53678=CARTESIAN_POINT ( 'NONE',  ( 1.533821497824999991, -81.47706753059999585, 0.4022281561003999695 ) ) ;
#53680=EDGE_CURVE ( 'NONE', #50158, #48229, #12339, .T. ) ;
#53702=CARTESIAN_POINT ( 'NONE',  ( -1.387963714323000142, -79.84219163730999469, 0.9213108730841000904 ) ) ;
#53705=VERTEX_POINT ( 'NONE', #17267 ) ;
#53709=ORIENTED_EDGE ( 'NONE', *, *, #3856, .T. ) ;
#53717=CARTESIAN_POINT ( 'NONE',  ( -1.397427047035999959, -78.31445671932998209, -0.8741189423671000824 ) ) ;
#53722=CARTESIAN_POINT ( 'NONE',  ( 1.231267358449230853, -80.33667723787161208, -0.2162300623809715050 ) ) ;
#53744=CYLINDRICAL_SURFACE ( 'NONE', #27927, 1.250000000000000000 ) ;
#53748=CARTESIAN_POINT ( 'NONE',  ( -1.392304720662999928, -81.41111398138998823, -0.3162235598901000366 ) ) ;
#53798=CARTESIAN_POINT ( 'NONE',  ( -0.7677219301324074152, -82.52774397455820576, 0.9995942476885919525 ) ) ;
#53801=CARTESIAN_POINT ( 'NONE',  ( 1.224974234943492446, -79.36964605286109986, 0.3088754873210631802 ) ) ;
#53810=CARTESIAN_POINT ( 'NONE',  ( 1.341343219651000229, -78.91326760749998925, -0.9216622887798999741 ) ) ;
#53851=CARTESIAN_POINT ( 'NONE',  ( -0.6332123272625999055, -81.17642093709999074, 1.540853336418999797 ) ) ;
#53852=CARTESIAN_POINT ( 'NONE',  ( 0.1056055121785000050, -79.32579514703000712, 1.430709028799999949 ) ) ;
#53854=CARTESIAN_POINT ( 'NONE',  ( 0.4262039658379053186, -82.60221317835673460, 1.450363779020775290 ) ) ;
#53864=EDGE_LOOP ( 'NONE', ( #44193, #4627, #34492, #9645 ) ) ;
#53893=CARTESIAN_POINT ( 'NONE',  ( 0.4719577028681999908, -80.73341720544999589, -1.266186157272999768 ) ) ;
#53935=DIRECTION ( 'NONE',  ( 0.000000000000000000, -1.000000000000000000, 0.000000000000000000 ) ) ;
#53937=ORIENTED_EDGE ( 'NONE', *, *, #45605, .F. ) ;
#53944=CARTESIAN_POINT ( 'NONE',  ( -1.500000000000000000, -83.28333333333331723, 0.000000000000000000 ) ) ;
#53969=CARTESIAN_POINT ( 'NONE',  ( -0.8705260234225306037, -80.27237256087059336, 1.278861286191462332 ) ) ;
#53978=CARTESIAN_POINT ( 'NONE',  ( 1.463006681111000074, -81.47722500425999215, -0.8714086385761999898 ) ) ;
#54013=CARTESIAN_POINT ( 'NONE',  ( -1.613562824561000086, -78.78634084733999998, -0.3366025691675999520 ) ) ;
#54016=CARTESIAN_POINT ( 'NONE',  ( 1.195573974400984119, -80.32674014211457347, -0.3649524205962666468 ) ) ;
#54043=CARTESIAN_POINT ( 'NONE',  ( 0.6445170026176001432, -82.29550046658999918, 1.319487011787000119 ) ) ;
#54044=CARTESIAN_POINT ( 'NONE',  ( 0.7658660592953000501, -79.84702375444000211, 1.113292320107999833 ) ) ;
#54069=CARTESIAN_POINT ( 'NONE',  ( 0.000000000000000000, -76.75499999999999545, 0.000000000000000000 ) ) ;
#54074=CARTESIAN_POINT ( 'NONE',  ( -1.119262997622045175, -81.79061289717962779, 1.016493713523941578 ) ) ;
#54096=ORIENTED_EDGE ( 'NONE', *, *, #56593, .F. ) ;
#54102=CARTESIAN_POINT ( 'NONE',  ( 0.3877229342594999961, -77.91453410555999426, -1.580612325761999948 ) ) ;
#54105=CARTESIAN_POINT ( 'NONE',  ( -0.1636246173744673738, -78.11458333333330017, -1.249999999999999778 ) ) ;
#54106=EDGE_CURVE ( 'NONE', #48229, #12675, #11265, .T. ) ;
#54132=EDGE_CURVE ( 'NONE', #27512, #9574, #15970, .T. ) ;
#54139=CARTESIAN_POINT ( 'NONE',  ( -0.6332123272625999055, -81.11720461324000553, 1.540853336418999797 ) ) ;
#54140=CARTESIAN_POINT ( 'NONE',  ( -1.485441059218000293, -77.87043921376999833, 0.4397084800123000070 ) ) ;
#54142=CARTESIAN_POINT ( 'NONE',  ( 1.009312198048121445, -83.06780995641257448, 1.154596580929102556 ) ) ;
#54149=CARTESIAN_POINT ( 'NONE',  ( 1.123730751682942453, -81.81383862517986927, -0.5490724999909163406 ) ) ;
#54170=APPLICATION_CONTEXT ( 'automotive_design' ) ;
#54194=CARTESIAN_POINT ( 'NONE',  ( -0.6295237254636235624, -79.08333333333332860, -1.092232985442822990 ) ) ;
#54215=CARTESIAN_POINT ( 'NONE',  ( -1.217465845835396188, -82.47916666666667140, 0.3271848554490955907 ) ) ;
#54223=CARTESIAN_POINT ( 'NONE',  ( -1.028867309006398445, -77.75000000000001421, 1.135838062686344241 ) ) ;
#54263=CARTESIAN_POINT ( 'NONE',  ( -1.217465845835396188, -80.97916666666667140, 0.3271848554490955907 ) ) ;
#54265=CARTESIAN_POINT ( 'NONE',  ( -0.3900435134041961294, -80.45456690170814795, -1.498726833963420102 ) ) ;
#54266=CARTESIAN_POINT ( 'NONE',  ( -0.8975083509913929225, -78.53903619159790139, 0.8699955927291534996 ) ) ;
#54275=DIRECTION ( 'NONE',  ( 1.000000000000000000, 0.000000000000000000, 0.000000000000000000 ) ) ;
#54310=CARTESIAN_POINT ( 'NONE',  ( 0.0006082099392775999975, -77.89500416108998593, -1.648286516476999974 ) ) ;
#54313=CARTESIAN_POINT ( 'NONE',  ( 0.2921935631638524211, -80.24396599101683591, -1.216359575293097350 ) ) ;
#54320=VERTEX_POINT ( 'NONE', #27431 ) ;
#54324=TOROIDAL_SURFACE ( 'NONE', #28854, 9.000000000000000000, 0.5000000000000000000 ) ;
#54337=CARTESIAN_POINT ( 'NONE',  ( -1.376471765390000046, -82.48497811192000029, -0.5116381728330999801 ) ) ;
#54349=ORIENTED_EDGE ( 'NONE', *, *, #15590, .F. ) ;
#54357=CARTESIAN_POINT ( 'NONE',  ( 0.9316830647087891437, -77.94531250006815526, 0.9357750704700737998 ) ) ;
#54368=CARTESIAN_POINT ( 'NONE',  ( 0.7772663842050028249, -81.51732138592326748, -1.296046382237271200 ) ) ;
#54386=CARTESIAN_POINT ( 'NONE',  ( -1.093189831540567036, -82.55899385228254062, 0.6295831063865356958 ) ) ;
#54399=CARTESIAN_POINT ( 'NONE',  ( 0.4192948356380000186, -79.47715281348000360, -1.440205485619000081 ) ) ;
#54428=VECTOR ( 'NONE', #41437, 1000.000000000000000 ) ;
#54439=CARTESIAN_POINT ( 'NONE',  ( -1.445929428138999828, -80.16981638657999554, 0.8273736140038000508 ) ) ;
#54440=CARTESIAN_POINT ( 'NONE',  ( -0.9076773815622000141, -79.31816002803999766, 1.255319232249999972 ) ) ;
#54442=CARTESIAN_POINT ( 'NONE',  ( -1.372670850766613659, -82.78440322194356327, -0.6347619962463861842 ) ) ;
#54444=DIRECTION ( 'NONE',  ( 0.000000000000000000, 0.000000000000000000, -1.000000000000000000 ) ) ;
#54447=CARTESIAN_POINT ( 'NONE',  ( 1.226805910823643986, -81.83485757964179186, -0.2432299854603273970 ) ) ;
#54468=CARTESIAN_POINT ( 'NONE',  ( -0.6295237254636286695, -81.41666666666667140, 1.092232985442819881 ) ) ;
#54477=CARTESIAN_POINT ( 'NONE',  ( 1.399788002916999785, -80.41777860354999063, 0.4438937798904999954 ) ) ;
#54532=CARTESIAN_POINT ( 'NONE',  ( 1.165652817183006063, -82.82060152807378017, -0.4515180940258363695 ) ) ;
#54559=CARTESIAN_POINT ( 'NONE',  ( -0.01370464116672059050, -78.47610054924975032, 1.249783674205719786 ) ) ;
#54568=CARTESIAN_POINT ( 'NONE',  ( -1.308644393797000038, -81.24548374185999933, -0.6845726736234999388 ) ) ;
#54581=VERTEX_POINT ( 'NONE', #39431 ) ;
#54600=CARTESIAN_POINT ( 'NONE',  ( -0.07808091635396000041, -78.89120398689999547, -1.646447584893999894 ) ) ;
#54604=CARTESIAN_POINT ( 'NONE',  ( -1.039294407854003843, -80.14744977795547243, -0.6948369225764182699 ) ) ;
#54606=CARTESIAN_POINT ( 'NONE',  ( 0.000000000000000000, -86.29999999996098836, -10.04999999996000071 ) ) ;
#54626=CARTESIAN_POINT ( 'NONE',  ( -0.4497554808884999811, -82.42197637046800196, 1.274241432965000032 ) ) ;
#54627=CARTESIAN_POINT ( 'NONE',  ( 1.100531998921000065, -79.72070532422000610, -0.7842560430284000184 ) ) ;
#54631=CARTESIAN_POINT ( 'NONE',  ( 0.7076411874954000591, -82.93030375670298326, -1.508144869335000138 ) ) ;
#54651=CARTESIAN_POINT ( 'NONE',  ( -1.179862061259663086, -81.57352980150935196, 0.4123850943632001442 ) ) ;
#54682=CARTESIAN_POINT ( 'NONE',  ( 0.4192948356380000186, -79.41793648960999974, -1.440205485619000081 ) ) ;
#54718=CARTESIAN_POINT ( 'NONE',  ( 0.4771943503223999850, -80.41851035578000051, -1.596102929133000004 ) ) ;
#54719=CARTESIAN_POINT ( 'NONE',  ( -0.5511083744702001130, -79.11070398689999195, -1.199565526491999989 ) ) ;
#54721=CARTESIAN_POINT ( 'NONE',  ( -1.064217634024700043, -81.81272298947914123, -1.071786072975686066 ) ) ;
#54722=CARTESIAN_POINT ( 'NONE',  ( 0.6756574613765372606, -83.18743617693904469, 1.353690879101595801 ) ) ;
#54726=CARTESIAN_POINT ( 'NONE',  ( -1.163712929666468110, -81.62986445498971477, -0.4567824189295925930 ) ) ;
#54731=ORIENTED_EDGE ( 'NONE', *, *, #34403, .T. ) ;
#54754=B_SPLINE_SURFACE_WITH_KNOTS ( 'NONE', 3, 3, ( 
 ( #26960, #27251, #5699, #18420, #54139, #44990, #5412, #442, #13679, #28123, #9853, #55007, #22837, #36123, #45880, #23420, #45291, #152, #46173, #54439, #41432, #9559, #14555, #32548, #4841, #1018, #23710, #41720, #50597, #49424, #36411, #40559, #17834, #18128, #31677 ),
 ( #10146, #35822, #40850, #31970, #53851, #8974, #45587, #4546, #5132, #22548, #23129, #49723, #9266, #729, #18709, #36703, #54718, #14261, #32257, #50303, #27834, #10736, #48409, #1883, #37575, #28417, #48126, #42315, #55592, #12378, #52538, #39238, #6286, #19576, #30076 ),
 ( #30366, #19877, #16817, #5992, #10432, #19291, #25658, #1586, #57250, #7945, #52823, #47842, #24301, #46764, #7659, #43388, #15141, #2947, #28712, #38663, #33136, #3243, #56683, #14845, #20947, #16240, #34219, #51179, #12095, #43689, #1298, #52254, #21235, #23998, #16528 ),
 ( #11812, #55299, #34801, #46464, #25948, #37283, #32839, #29787, #50886, #42016, #7373, #25373, #38952, #56965, #34507, #4, #31232, #13540, #21523, #3806, #26516, #9124, #30656, #49577, #49274, #40107, #17682, #53702, #8826, #58120, #35671, #35077, #17982, #26813, #22397 ) ),
 .UNSPECIFIED., .F., .F., .F.,
 ( 4, 4 ),
 ( 4, 1, 1, 1, 1, 1, 1, 1, 1, 1, 1, 1, 1, 1, 1, 1, 1, 1, 1, 1, 1, 1, 1, 1, 1, 1, 1, 1, 1, 1, 1, 1, 4 ),
 ( -0.3882448580381000491, 1.388244858038000018 ),
 ( -0.02000000000000000042, 0.01250000000000000069, 0.04499999999999999833, 0.07749999999999999944, 0.1100000000000000006, 0.1424999999999999878, 0.1749999999999999889, 0.2074999999999999900, 0.2399999999999999911, 0.2725000000000000200, 0.3049999999999999933, 0.3375000000000000222, 0.3699999999999999956, 0.4025000000000000244, 0.4349999999999999978, 0.4675000000000000266, 0.5000000000000000000, 0.5324999999999999734, 0.5649999999999999467, 0.5975000000000000311, 0.6300000000000000044, 0.6624999999999999778, 0.6949999999999999512, 0.7275000000000000355, 0.7600000000000000089, 0.7924999999999999822, 0.8249999999999999556, 0.8575000000000000400, 0.8900000000000000133, 0.9224999999999999867, 0.9549999999999999600, 0.9875000000000000444, 1.020000000000000018 ),
 .UNSPECIFIED. ) ;
#54755=EDGE_CURVE ( 'NONE', #13712, #46203, #13339, .T. ) ;
#54756=CARTESIAN_POINT ( 'NONE',  ( -1.456085397364999867, -81.23900587363999648, -0.6271128268704999620 ) ) ;
#54758=DIRECTION ( 'NONE',  ( 0.000000000000000000, 1.000000000000000000, 0.000000000000000000 ) ) ;
#54846=CARTESIAN_POINT ( 'NONE',  ( 0.6196687357644999894, -82.42461323090898873, -1.586136063883000213 ) ) ;
#54853=DIRECTION ( 'NONE',  ( -1.000000000000000000, 0.000000000000000000, 0.000000000000000000 ) ) ;
#54859=ORIENTED_EDGE ( 'NONE', *, *, #46191, .F. ) ;
#54870=CIRCLE ( 'NONE', #5856, 1.250000000000000000 ) ;
#54886=CARTESIAN_POINT ( 'NONE',  ( -0.4639630351240068284, -78.24932064131154164, 1.464561517630637910 ) ) ;
#54904=CARTESIAN_POINT ( 'NONE',  ( -1.217840012802438698, -78.62105508162261458, -0.3270303979875727740 ) ) ;
#54909=CARTESIAN_POINT ( 'NONE',  ( -1.561527218546999940, -82.29871160559999055, -0.5804237711334999661 ) ) ;
#54925=VERTEX_POINT ( 'NONE', #57049 ) ;
#54966=CARTESIAN_POINT ( 'NONE',  ( 0.3877229342594999961, -77.85531778169000461, -1.580612325761999948 ) ) ;
#55007=CARTESIAN_POINT ( 'NONE',  ( -1.497546582071999977, -80.67509010745999376, 0.7298035716741000378 ) ) ;
#55008=CARTESIAN_POINT ( 'NONE',  ( 0.9487295532135000542, -78.33116200998999545, 0.9179270638336999300 ) ) ;
#55010=CARTESIAN_POINT ( 'NONE',  ( -1.388199995259592479, -81.78235798221467689, -0.5980877822880301675 ) ) ;
#55028=DIRECTION ( 'NONE',  ( 0.000000000000000000, 1.000000000000000000, 0.000000000000000000 ) ) ;
#55044=CARTESIAN_POINT ( 'NONE',  ( -0.5171309048475001280, -81.30216508874998738, -1.330821326197000110 ) ) ;
#55121=CARTESIAN_POINT ( 'NONE',  ( -0.1192998693168455110, -82.98315628367254249, 1.244397729618985871 ) ) ;
#55127=CARTESIAN_POINT ( 'NONE',  ( -1.065760231334440311, -79.78652098530383796, 1.072882827548660156 ) ) ;
#55166=CARTESIAN_POINT ( 'NONE',  ( -1.247931803916645821, -80.59581569326661565, 0.07626238930717134379 ) ) ;
#55177=CARTESIAN_POINT ( 'NONE',  ( -1.099011084613188860, -80.13991461626227419, -0.5953293180670605755 ) ) ;
#55178=CARTESIAN_POINT ( 'NONE',  ( 1.321783848197346511, -77.89322916679840603, -0.3543445508106254915 ) ) ;
#55182=CARTESIAN_POINT ( 'NONE',  ( -1.330154178996141967, -78.89180944238322013, -0.7730572632364612895 ) ) ;
#55198=CARTESIAN_POINT ( 'NONE',  ( -0.5525270872808000222, -82.61145401579800307, -1.233160589678000019 ) ) ;
#55206=CARTESIAN_POINT ( 'NONE',  ( 1.274651354540000003, -82.80309610059499903, -0.4485964608026000167 ) ) ;
#55225=EDGE_CURVE ( 'NONE', #25256, #10013, #15135, .T. ) ;
#55228=CARTESIAN_POINT ( 'NONE',  ( -0.8004101649314999678, -77.65262252499999818, -1.034513833287000084 ) ) ;
#55234=ORIENTED_EDGE ( 'NONE', *, *, #40266, .F. ) ;
#55257=CARTESIAN_POINT ( 'NONE',  ( 0.4102083068199999794, -78.41566823357999283, -1.574926093281000083 ) ) ;
#55259=CARTESIAN_POINT ( 'NONE',  ( -0.8591865374099513231, -79.16499716410996257, -0.9081973555077933469 ) ) ;
#55266=CARTESIAN_POINT ( 'NONE',  ( -0.5171309048475001280, -81.48884839998999041, -1.330821326197000110 ) ) ;
#55299=CARTESIAN_POINT ( 'NONE',  ( -0.9131908197385000259, -81.46327815847000409, -1.254418330386999791 ) ) ;
#55302=CARTESIAN_POINT ( 'NONE',  ( 1.270052417142802925, -81.95442635671317078, -0.8198608233724109517 ) ) ;
#55308=CARTESIAN_POINT ( 'NONE',  ( -0.4780979534308362200, -81.69389049006093728, -1.154869708129174111 ) ) ;
#55338=CARTESIAN_POINT ( 'NONE',  ( -0.7224186015757000368, -79.15443682768999167, -0.9790252285018000711 ) ) ;
#55372=CARTESIAN_POINT ( 'NONE',  ( -0.1636246173744673738, -82.61458333333330017, -1.249999999999999778 ) ) ;
#55391=CARTESIAN_POINT ( 'NONE',  ( 1.155591953334705657, -82.81890755821275718, -0.4764985287334481123 ) ) ;
#55404=CARTESIAN_POINT ( 'NONE',  ( 1.250000000000000000, -81.24999999999998579, 0.000000000000000000 ) ) ;
#55414=CARTESIAN_POINT ( 'NONE',  ( 1.030642090993115989, -82.89809790103859655, 0.7070660955623684352 ) ) ;
#55428=CARTESIAN_POINT ( 'NONE',  ( -1.249999999999999778, -80.51041666666664298, -0.1636246173744686228 ) ) ;
#55444=CARTESIAN_POINT ( 'NONE',  ( -0.7572724432162000197, -83.30137326488198823, 1.483977110291999857 ) ) ;
#55473=CARTESIAN_POINT ( 'NONE',  ( -1.063570462605010869, -80.14457819395771310, -0.6576264011075878546 ) ) ;
#55477=CARTESIAN_POINT ( 'NONE',  ( 1.095260562757544687, -78.16008608560689197, 1.039742534048890832 ) ) ;
#55482=DIRECTION ( 'NONE',  ( 0.000000000000000000, -1.000000000000000000, 0.000000000000000000 ) ) ;
#55492=CARTESIAN_POINT ( 'NONE',  ( -1.074445222347000017, -83.55884224245099290, -0.5709172427956999973 ) ) ;
#55495=CARTESIAN_POINT ( 'NONE',  ( -0.9995835529977281642, -78.94791666666662877, 0.7681833999686391579 ) ) ;
#55505=VERTEX_POINT ( 'NONE', #52989 ) ;
#55520=CARTESIAN_POINT ( 'NONE',  ( 1.045473607267330740, -81.39676167661833972, 0.6855302019354867493 ) ) ;
#55525=CARTESIAN_POINT ( 'NONE',  ( -0.5791533927176000240, -78.49152764148000472, 1.172759083288000159 ) ) ;
#55541=ORIENTED_EDGE ( 'NONE', *, *, #23548, .T. ) ;
#55551=CARTESIAN_POINT ( 'NONE',  ( 0.4192948356380000186, -79.53636913735000746, -1.440205485619000081 ) ) ;
#55561=CARTESIAN_POINT ( 'NONE',  ( -1.530783851654999861, -80.79393956010999034, 0.7460011833842999929 ) ) ;
#55592=CARTESIAN_POINT ( 'NONE',  ( -0.3164372427141999844, -79.66059977445999607, 1.635583079321000000 ) ) ;
#55593=CARTESIAN_POINT ( 'NONE',  ( 0.1413472186869999814, -77.88570945174998883, 1.208470106255999932 ) ) ;
#55600=CARTESIAN_POINT ( 'NONE',  ( 1.212634435040167658, -79.83097499881669989, -0.3047410518862661011 ) ) ;
#55601=CARTESIAN_POINT ( 'NONE',  ( 1.250000000000000000, -80.84999999999999432, 0.000000000000000000 ) ) ;
#55603=CARTESIAN_POINT ( 'NONE',  ( 0.004852466274130710043, -81.72588911470774065, -1.249646052481410141 ) ) ;
#55620=ORIENTED_EDGE ( 'NONE', *, *, #52709, .F. ) ;
#55629=CARTESIAN_POINT ( 'NONE',  ( 1.100531998921000065, -79.28075525790998768, -0.7842560430285000495 ) ) ;
#55634=CARTESIAN_POINT ( 'NONE',  ( 0.5368854727554398520, -79.59607745916922283, 1.411883060306194926 ) ) ;
#55635=VECTOR ( 'NONE', #12453, 1000.000000000000000 ) ;
#55689=CARTESIAN_POINT ( 'NONE',  ( 1.156359412676422282, -82.81903375624176533, -0.4746362260554010670 ) ) ;
#55692=CARTESIAN_POINT ( 'NONE',  ( -1.191119343893799920, -79.57605893021457177, 0.3784560293714495649 ) ) ;
#55693=CARTESIAN_POINT ( 'NONE',  ( 1.528777005363244568, -78.99356928323743432, -0.1184073789878865995 ) ) ;
#55694=CARTESIAN_POINT ( 'NONE',  ( -9.949999999959999286, -86.19999999995999929, -1.488372002482999864E-09 ) ) ;
#55701=CARTESIAN_POINT ( 'NONE',  ( 0.6295237254636258939, -81.16666666666665719, -1.092232985442821658 ) ) ;
#55715=CARTESIAN_POINT ( 'NONE',  ( -0.5008228193151907925, -83.00788715391320238, 1.145400540283604496 ) ) ;
#55721=EDGE_CURVE ( 'NONE', #16901, #45372, #47175, .T. ) ;
#55745=FACE_OUTER_BOUND ( 'NONE', #15958, .T. ) ;
#55749=EDGE_LOOP ( 'NONE', ( #4403, #49511, #46520, #48641 ) ) ;
#55761=CARTESIAN_POINT ( 'NONE',  ( 0.6783686788296603432, -80.42946718699170106, 1.049845246189362147 ) ) ;
#55772=CARTESIAN_POINT ( 'NONE',  ( -0.4778988054446937639, -80.19393997919249273, -1.154928669624085691 ) ) ;
#55776=CARTESIAN_POINT ( 'NONE',  ( -0.7609899864356860499, -79.26659457633572003, 1.304350159878486570 ) ) ;
#55790=EDGE_LOOP ( 'NONE', ( #46387, #32403, #33813, #28569 ) ) ;
#55794=CARTESIAN_POINT ( 'NONE',  ( -1.217465845835396188, -82.97916666666668561, 0.3271848554490955907 ) ) ;
#55800=CARTESIAN_POINT ( 'NONE',  ( -0.4497554808884999811, -81.98202630415998726, 1.274241432965000032 ) ) ;
#55803=CARTESIAN_POINT ( 'NONE',  ( 1.092232985442823212, -82.20833333333331439, -0.6295237254636224522 ) ) ;
#55818=CARTESIAN_POINT ( 'NONE',  ( 1.154165937183204926, -81.38156932103548513, 0.4796374930683212634 ) ) ;
#55823=CARTESIAN_POINT ( 'NONE',  ( -0.1495270637475999975, -79.02672845825999559, 1.413525301447999816 ) ) ;
#55829=ORIENTED_EDGE ( 'NONE', *, *, #7574, .F. ) ;
#55849=DIRECTION ( 'NONE',  ( -1.996944831318000060E-10, 1.000000000000000000, 5.653829486504999768E-11 ) ) ;
#55850=CARTESIAN_POINT ( 'NONE',  ( 0.000000000000000000, -76.75499999999999545, 0.000000000000000000 ) ) ;
#55851=CARTESIAN_POINT ( 'NONE',  ( -0.9536002873971000104, -79.31364285822999705, 1.318830682536000110 ) ) ;
#55874=ORIENTED_EDGE ( 'NONE', *, *, #51400, .F. ) ;
#55887=CARTESIAN_POINT ( 'NONE',  ( -0.8890245797214872958, -80.03847917517971666, 0.8782872498970755171 ) ) ;
#55891=CARTESIAN_POINT ( 'NONE',  ( 0.3417741717619000030, -78.10080061187998979, -1.393295110451999941 ) ) ;
#55893=CARTESIAN_POINT ( 'NONE',  ( 0.5361682633709462520, -81.90381801127249162, -1.413805704914858241 ) ) ;
#55897=CARTESIAN_POINT ( 'NONE',  ( 1.093259379017939681, -80.89232953274604654, 0.6295269788946473710 ) ) ;
#55899=CARTESIAN_POINT ( 'NONE',  ( -0.8383438467763877355, -81.66698421707488365, -0.9271207089584655447 ) ) ;
#55903=CARTESIAN_POINT ( 'NONE',  ( 0.000000000000000000, -76.75499999999999545, 0.000000000000000000 ) ) ;
#55908=DIRECTION ( 'NONE',  ( 1.000000000000000000, 0.000000000000000000, 0.000000000000000000 ) ) ;
#55912=DIRECTION ( 'NONE',  ( 1.000000000000000000, 0.000000000000000000, 0.000000000000000000 ) ) ;
#55929=CARTESIAN_POINT ( 'NONE',  ( -1.530783851654999861, -80.73388962642000877, 0.7460011833842999929 ) ) ;
#55933=CARTESIAN_POINT ( 'NONE',  ( -0.03127831795120067371, -79.37340073922844397, -1.510815432793727986 ) ) ;
#55948=CARTESIAN_POINT ( 'NONE',  ( 1.179985190145098173, -78.37701668321712134, 0.4119397061850897934 ) ) ;
#55970=CARTESIAN_POINT ( 'NONE',  ( 1.115616509574796078, -78.30837352953511754, -0.6527249703762391109 ) ) ;
#55982=ORIENTED_EDGE ( 'NONE', *, *, #52097, .F. ) ;
#55983=CARTESIAN_POINT ( 'NONE',  ( 0.3045730287770247458, -82.74492401537455066, -1.212283547811195739 ) ) ;
#55990=CARTESIAN_POINT ( 'NONE',  ( 1.507222751313145093, -77.98526986442249154, -0.2769236843535003434 ) ) ;
#55991=DIRECTION ( 'NONE',  ( -0.7071067811865969777, -0.7071067811864980568, 1.236220812569996176E-09 ) ) ;
#56007=CARTESIAN_POINT ( 'NONE',  ( 0.4362293792333048481, -82.94664917577976837, 1.171447771671162652 ) ) ;
#56019=( LENGTH_UNIT ( ) NAMED_UNIT ( * ) SI_UNIT ( .MILLI., .METRE. ) );
#56031=CARTESIAN_POINT ( 'NONE',  ( -1.462746796095000024, -81.40659681158000183, -0.3322225316158000097 ) ) ;
#56050=EDGE_LOOP ( 'NONE', ( #959, #11600, #21865, #52713, #30950 ) ) ;
#56051=CARTESIAN_POINT ( 'NONE',  ( -0.8920742119596244413, -80.53887022317101696, 0.8750902781345917258 ) ) ;
#56052=CARTESIAN_POINT ( 'NONE',  ( 1.250000000000000000, -82.24999999999998579, 0.000000000000000000 ) ) ;
#56069=CARTESIAN_POINT ( 'NONE',  ( 1.379693150491080988, -79.13274274277868869, 0.6107116112576068678 ) ) ;
#56081=CARTESIAN_POINT ( 'NONE',  ( -1.512396851278637433, -80.23374261172247657, 0.3224664540911364452 ) ) ;
#56083=CARTESIAN_POINT ( 'NONE',  ( 1.249999999999999778, -79.26041666666667140, 0.1636246173744711763 ) ) ;
#56084=CARTESIAN_POINT ( 'NONE',  ( -0.1636246173744726473, -82.88541666666664298, 1.249999999999999112 ) ) ;
#56096=CARTESIAN_POINT ( 'NONE',  ( -0.2199206942898871420, -79.39661240347331272, -1.482330506908097201 ) ) ;
#56110=CARTESIAN_POINT ( 'NONE',  ( 1.149808842311183410, -81.38230583544610397, 0.4899631106986611084 ) ) ;
#56112=CARTESIAN_POINT ( 'NONE',  ( -0.1639543601470098144, -82.21523505733837567, -1.249472255457048098 ) ) ;
#56114=CARTESIAN_POINT ( 'NONE',  ( -1.223460966046000076, -77.56523657536999394, 0.2343682768462999888 ) ) ;
#56143=CARTESIAN_POINT ( 'NONE',  ( 1.136899222205000060, -79.14306339479999508, 1.164526648744999893 ) ) ;
#56149=ORIENTED_EDGE ( 'NONE', *, *, #31266, .T. ) ;
#56151=CARTESIAN_POINT ( 'NONE',  ( 1.386886761648000066, -79.53075525790998768, -0.9883168548346998872 ) ) ;
#56159=CARTESIAN_POINT ( 'NONE',  ( 0.9801489377500960387, -81.29702506321740429, -0.7880733966296984416 ) ) ;
#56161=CARTESIAN_POINT ( 'NONE',  ( 0.000000000000000000, -76.75499999999999545, 0.000000000000000000 ) ) ;
#56171=CARTESIAN_POINT ( 'NONE',  ( -0.3865739120649937521, -79.45398714331572876, -1.459136857207182114 ) ) ;
#56175=CARTESIAN_POINT ( 'NONE',  ( 1.335937499394570516, -77.91406250010766144, 0.2110757592694599283 ) ) ;
#56177=CARTESIAN_POINT ( 'NONE',  ( -0.9344580297550504344, -80.04259503167067180, 0.8300580218378730279 ) ) ;
#56184=CARTESIAN_POINT ( 'NONE',  ( 0.9992560168720977520, -78.90234941287772585, 0.7679384024261605157 ) ) ;
#56186=CARTESIAN_POINT ( 'NONE',  ( 0.1761264049549336741, -82.21573302580067377, 1.536971449393705447 ) ) ;
#56187=CARTESIAN_POINT ( 'NONE',  ( -0.4741829603392039294, -79.69437006906809984, -1.156353086730761870 ) ) ;
#56201=CARTESIAN_POINT ( 'NONE',  ( 0.000000000000000000, -77.50000000000000000, 0.000000000000000000 ) ) ;
#56217=CARTESIAN_POINT ( 'NONE',  ( 0.5947595261268000533, -80.92336727174999567, -1.595643580583000043 ) ) ;
#56239=CARTESIAN_POINT ( 'NONE',  ( 1.233647025524779339, -78.36298610943158849, 0.2016259055441099179 ) ) ;
#56242=DIRECTION ( 'NONE',  ( -1.000000000000000000, 0.000000000000000000, 0.000000000000000000 ) ) ;
#56251=CARTESIAN_POINT ( 'NONE',  ( -1.494641324160000062, -79.36620647882999435, -0.7306109071898999607 ) ) ;
#56256=CARTESIAN_POINT ( 'NONE',  ( -1.250000000000000000, -78.50000000000000000, 0.000000000000000000 ) ) ;
#56273=CARTESIAN_POINT ( 'NONE',  ( 0.3307596944394597949, -82.74658640164716417, -1.205731917451906554 ) ) ;
#56278=CARTESIAN_POINT ( 'NONE',  ( -0.5546092031877057904, -79.51207562121919636, 1.122904892616682249 ) ) ;
#56279=CARTESIAN_POINT ( 'NONE',  ( -1.433156267533250983, -78.72468943822306642, 0.4708507765673180523 ) ) ;
#56287=CARTESIAN_POINT ( 'NONE',  ( -1.358260632703687021, -81.38578242155206510, -0.6678246071336888523 ) ) ;
#56295=CARTESIAN_POINT ( 'NONE',  ( 0.8976219970198608955, -82.91185551150395838, 0.8696104471699304117 ) ) ;
#56328=ORIENTED_EDGE ( 'NONE', *, *, #27821, .F. ) ;
#56331=DIRECTION ( 'NONE',  ( 0.000000000000000000, -1.000000000000000000, 0.000000000000000000 ) ) ;
#56337=CARTESIAN_POINT ( 'NONE',  ( 0.5131766215739365089, -80.44137981884804844, 1.140404433670309858 ) ) ;
#56366=CARTESIAN_POINT ( 'NONE',  ( 0.3271848554491016414, -78.64583333333330017, -1.217465845835393967 ) ) ;
#56368=CARTESIAN_POINT ( 'NONE',  ( 1.226384192711576837, -79.95033587725438906, -0.8842796768856556744 ) ) ;
#56397=CARTESIAN_POINT ( 'NONE',  ( 1.249556443808253592, -82.34024392821149263, -0.1639605875127234658 ) ) ;
#56421=DIRECTION ( 'NONE',  ( -0.7071067811865975328, -0.7071067811864976127, 2.062933177233993779E-09 ) ) ;
#56429=AXIS2_PLACEMENT_3D ( 'NONE', #30509, #12226, #56242 ) ;
#56431=CARTESIAN_POINT ( 'NONE',  ( 1.619712389308999967, -79.08738182501998892, 0.1587296492880999887 ) ) ;
#56466=CARTESIAN_POINT ( 'NONE',  ( -0.4841670057754499656, -80.00688952560039979, 1.152271897791588229 ) ) ;
#56471=CARTESIAN_POINT ( 'NONE',  ( 1.092501263137524159, -78.89193896525061689, 0.6295016473291589199 ) ) ;
#56472=CARTESIAN_POINT ( 'NONE',  ( -1.417317677626557471, -81.82097862065256777, 0.5276391229990249343 ) ) ;
#56473=CARTESIAN_POINT ( 'NONE',  ( -0.8507816195585579111, -79.66573003440132084, -0.9156227843767963392 ) ) ;
#56505=CARTESIAN_POINT ( 'NONE',  ( 1.653747448240000084, -80.03913826020999522, 0.4061235413877000155 ) ) ;
#56524=CARTESIAN_POINT ( 'NONE',  ( 0.3102673461446125436, -78.45508004528514334, 1.211442227934462323 ) ) ;
#56537=CARTESIAN_POINT ( 'NONE',  ( 0.1224622883215999852, -79.19916176948999009, 1.659079133038000142 ) ) ;
#56546=CARTESIAN_POINT ( 'NONE',  ( -0.7681833999686477066, -81.92708333333332860, 0.9995835529977223910 ) ) ;
#56551=VERTEX_POINT ( 'NONE', #51596 ) ;
#56561=CARTESIAN_POINT ( 'NONE',  ( 0.1647566600028030070, -79.46510844028065890, 1.241328820898986329 ) ) ;
#56562=CARTESIAN_POINT ( 'NONE',  ( -1.342108659710564034, -78.28775969006993307, -0.6887887724524024424 ) ) ;
#56572=CARTESIAN_POINT ( 'NONE',  ( -0.8903047578514302618, -81.27444143548434852, 1.221612336925710807 ) ) ;
#56593=EDGE_CURVE ( 'NONE', #41153, #8320, #33049, .T. ) ;
#56605=CARTESIAN_POINT ( 'NONE',  ( 1.579899301681999990, -82.16450739290000627, 0.5283722218587000308 ) ) ;
#56616=CARTESIAN_POINT ( 'NONE',  ( 0.1431601642728717039, -80.73480119803696198, -1.243017257267813758 ) ) ;
#56622=CARTESIAN_POINT ( 'NONE',  ( 0.07224473200327397038, -80.47101823697612133, 1.250019735964936540 ) ) ;
#56655=CARTESIAN_POINT ( 'NONE',  ( -0.6248080770815239715, -80.84104275701125175, -1.377230163493380788 ) ) ;
#56664=CARTESIAN_POINT ( 'NONE',  ( -1.376471765390000046, -82.17166142314999888, -0.5116381728330999801 ) ) ;
#56682=CARTESIAN_POINT ( 'NONE',  ( 1.102516846580866128, -81.38947583744716496, 0.5887672520915298024 ) ) ;
#56683=CARTESIAN_POINT ( 'NONE',  ( 1.617840321509000034, -80.09877138898998794, 0.3973055507782000118 ) ) ;
#56692=LINE ( 'NONE', #48136, #16774 ) ;
#56720=CARTESIAN_POINT ( 'NONE',  ( 0.1982664792347280658, -81.63720639545748270, -1.259862767458886257 ) ) ;
#56721=CARTESIAN_POINT ( 'NONE',  ( 0.1429208184976999974, -78.69761083655998846, 1.621183732314999792 ) ) ;
#56723=CARTESIAN_POINT ( 'NONE',  ( -1.249811141842820161, -79.10985391374313735, -0.1498213877793858617 ) ) ;
#56731=CARTESIAN_POINT ( 'NONE',  ( 0.8102226603197999477, -80.22566409777999752, 1.363061245571999924 ) ) ;
#56740=CARTESIAN_POINT ( 'NONE',  ( 0.4517135710334128085, -81.25462243997134237, -1.165398785623916522 ) ) ;
#56757=CARTESIAN_POINT ( 'NONE',  ( -1.197877150778747124, -80.07738762097918084, 0.3567682535721993786 ) ) ;
#56763=CARTESIAN_POINT ( 'NONE',  ( 1.218014849295945723, -78.87111806999728003, 0.3275086013355714143 ) ) ;
#56764=CARTESIAN_POINT ( 'NONE',  ( 0.8897706433943217696, -82.17524539450347731, 1.268930192044961380 ) ) ;
#56765=CARTESIAN_POINT ( 'NONE',  ( -0.6126584217143548061, -79.68445856097022784, -1.092851559434964814 ) ) ;
#56794=CARTESIAN_POINT ( 'NONE',  ( -1.666294527194000175, -79.78650139976998901, -0.3511123450079000063 ) ) ;
#56814=CARTESIAN_POINT ( 'NONE',  ( 1.248526980818341237, -78.35470678600303529, 0.07396862603816467541 ) ) ;
#56828=CARTESIAN_POINT ( 'NONE',  ( -1.085757491496805560, -82.05909138311299955, 0.6269543719623986711 ) ) ;
#56851=ORIENTED_EDGE ( 'NONE', *, *, #44468, .T. ) ;
#56853=CARTESIAN_POINT ( 'NONE',  ( -1.515185110494049470, -78.75829941884984464, -0.1588823915039442869 ) ) ;
#56873=CARTESIAN_POINT ( 'NONE',  ( 1.153972371676974751, -82.88143275804098664, 0.4803910728602110436 ) ) ;
#56913=CARTESIAN_POINT ( 'NONE',  ( -0.3222441879806262066, -80.49579513225657479, 1.208098981363385560 ) ) ;
#56927=CARTESIAN_POINT ( 'NONE',  ( -1.041898385056842402, -77.78530095164687452, 1.092208633748498636 ) ) ;
#56931=PLANE ( 'NONE',  #26657 ) ;
#56938=CARTESIAN_POINT ( 'NONE',  ( -1.090924692763506121, -80.81067774974684426, -1.044066399784976618 ) ) ;
#56947=CARTESIAN_POINT ( 'NONE',  ( -0.3643839585117999991, -81.47675258327998904, 1.301227969886000091 ) ) ;
#56961=DIRECTION ( 'NONE',  ( 1.000000000000000000, 0.000000000000000000, 0.000000000000000000 ) ) ;
#56965=CARTESIAN_POINT ( 'NONE',  ( 0.7545134501129999727, -80.72642064884999513, 1.485250302772000097 ) ) ;
#56972=CARTESIAN_POINT ( 'NONE',  ( -1.092232985442824100, -78.45833333333328596, 0.6295237254636200097 ) ) ;
#56978=VERTEX_POINT ( 'NONE', #46538 ) ;
#56985=DIRECTION ( 'NONE',  ( -0.7071067811865474617, 0.7071067811865474617, -2.768420520316182841E-09 ) ) ;
#56995=CARTESIAN_POINT ( 'NONE',  ( -1.092232985442822102, -83.04166666666664298, -0.6295237254636245616 ) ) ;
#57008=CARTESIAN_POINT ( 'NONE',  ( -1.631971144587999856, -81.85307101349999925, -0.4862994432698999892 ) ) ;
#57010=CARTESIAN_POINT ( 'NONE',  ( 1.561568621681000080, -79.65723116178999419, 0.2753811681071999806 ) ) ;
#57040=CARTESIAN_POINT ( 'NONE',  ( -1.025450104155645858, -80.05165854934456604, 0.7168883596936641567 ) ) ;
#57046=CARTESIAN_POINT ( 'NONE',  ( 0.6297746568761206643, -78.93358075575952171, 1.092604805766054010 ) ) ;
#57047=CARTESIAN_POINT ( 'NONE',  ( -0.2222643924572317575, -81.96268533019295432, -1.494766702788131507 ) ) ;
#57048=CARTESIAN_POINT ( 'NONE',  ( 0.04273675807453811148, -79.72806120046924150, -1.249183804664953268 ) ) ;
#57049=CARTESIAN_POINT ( 'NONE',  ( 2.299999999999999822, -77.50000000000000000, 0.000000000000000000 ) ) ;
#57066=ORIENTED_EDGE ( 'NONE', *, *, #17692, .F. ) ;
#57076=CARTESIAN_POINT ( 'NONE',  ( -0.4334656432294999862, -80.16545669043000544, 1.646792182271999971 ) ) ;
#57077=CARTESIAN_POINT ( 'NONE',  ( -1.249999999999999778, -81.01041666666665719, -0.1636246173744686228 ) ) ;
#57078=ORIENTED_EDGE ( 'NONE', *, *, #38361, .F. ) ;
#57108=CARTESIAN_POINT ( 'NONE',  ( 0.2234679122977781540, -81.96125120072602499, 1.229696476816594108 ) ) ;
#57109=ADVANCED_FACE ( 'NONE', ( #34656 ), #15831, .F. ) ;
#57114=FACE_OUTER_BOUND ( 'NONE', #3409, .T. ) ;
#57153=CARTESIAN_POINT ( 'NONE',  ( 1.153116094663966251, -82.88157216681773320, 0.4824474276636376846 ) ) ;
#57178=VERTEX_POINT ( 'NONE', #6870 ) ;
#57179=VECTOR ( 'NONE', #25444, 1000.000000000000000 ) ;
#57189=ORIENTED_EDGE ( 'NONE', *, *, #20043, .F. ) ;
#57222=CARTESIAN_POINT ( 'NONE',  ( 0.9056516610957285884, -81.07384114603890168, 1.208906470985191106 ) ) ;
#57232=CARTESIAN_POINT ( 'NONE',  ( -1.183213148269000259, -81.53991179838999415, 0.6526699808710000328 ) ) ;
#57244=CARTESIAN_POINT ( 'NONE',  ( -0.3862712429687000237, -78.00000000000000000, 1.188820645369000006 ) ) ;
#57246=DIRECTION ( 'NONE',  ( 0.000000000000000000, 1.000000000000000000, 0.000000000000000000 ) ) ;
#57248=DIRECTION ( 'NONE',  ( 0.000000000000000000, -1.000000000000000000, 0.000000000000000000 ) ) ;
#57250=CARTESIAN_POINT ( 'NONE',  ( 0.5818457612699999837, -80.98300040053000259, -1.560998038830999857 ) ) ;
#57265=CARTESIAN_POINT ( 'NONE',  ( 0.6885956969122000171, -77.97809706267000252, 1.243482171564999961 ) ) ;
#57290=CARTESIAN_POINT ( 'NONE',  ( -1.222545847381571127, -79.11929213067102751, -0.2981043881531356132 ) ) ;
#57300=CARTESIAN_POINT ( 'NONE',  ( -1.359874270581000077, -81.42584665852999137, 0.5545210745837000355 ) ) ;
#57304=CARTESIAN_POINT ( 'NONE',  ( 0.8286895765316001361, -81.54474391552000156, 1.445177540541999983 ) ) ;
#57325=CARTESIAN_POINT ( 'NONE',  ( 1.138160268254951646, -79.88425004917058914, 0.5165142851595377893 ) ) ;
#57331=CARTESIAN_POINT ( 'NONE',  ( -1.169763865275986525, -82.90402275785740471, -0.9575444884849958482 ) ) ;
#57333=CARTESIAN_POINT ( 'NONE',  ( -0.7154746835691508933, -79.67666239307115461, -1.026037770346891698 ) ) ;
#57347=AXIS2_PLACEMENT_3D ( 'NONE', #12418, #7411, #8272 ) ;
#57395=CYLINDRICAL_SURFACE ( 'NONE', #2798, 1.250000000000000000 ) ;
#57400=CARTESIAN_POINT ( 'NONE',  ( 0.8960442985632506296, -81.91201433914557128, 0.8711734550944890687 ) ) ;
#57401=CARTESIAN_POINT ( 'NONE',  ( -0.6945049390072000062, -78.92075392059999217, -1.511688483436000041 ) ) ;
#57411=CARTESIAN_POINT ( 'NONE',  ( 0.6295237254636211199, -81.83333333333334281, 1.092232985442824322 ) ) ;
#57421=ORIENTED_EDGE ( 'NONE', *, *, #13353, .F. ) ;
#57427=ORIENTED_EDGE ( 'NONE', *, *, #11235, .F. ) ;
#57435=DIRECTION ( 'NONE',  ( 0.000000000000000000, -1.000000000000000000, 0.000000000000000000 ) ) ;
#57482=ORIENTED_EDGE ( 'NONE', *, *, #21366, .F. ) ;
#57491=CARTESIAN_POINT ( 'NONE',  ( -1.344070316215177030, -77.81207131835833479, 0.6864365363003362974 ) ) ;
#57499=CARTESIAN_POINT ( 'NONE',  ( -0.6295237254636286695, -83.41666666666668561, 1.092232985442819881 ) ) ;
#57504=CARTESIAN_POINT ( 'NONE',  ( -1.217465845835394411, -78.52083333333332860, -0.3271848554491003647 ) ) ;
#57505=CARTESIAN_POINT ( 'NONE',  ( 1.238215446118554164, -80.15090966697889030, 0.9263567608796238195 ) ) ;
#57516=CARTESIAN_POINT ( 'NONE',  ( -1.477496145247999992, -82.67709261769098816, 0.5756751103899000466 ) ) ;
#57519=CARTESIAN_POINT ( 'NONE',  ( -1.217465845835394411, -82.02083333333330017, -0.3271848554491003647 ) ) ;
#57580=CARTESIAN_POINT ( 'NONE',  ( -0.4670233199325999895, -80.85741372253998804, 1.392241846115000126 ) ) ;
#57594=DIRECTION ( 'NONE',  ( 0.000000000000000000, -1.000000000000000000, 0.000000000000000000 ) ) ;
#57597=B_SPLINE_CURVE_WITH_KNOTS ( 'NONE', 3,
 ( #4410, #25960, #22413, #12677 ),
 .UNSPECIFIED., .F., .F.,
 ( 4, 4 ),
 ( 0.000000000000000000, 1.000000000000000000 ),
 .UNSPECIFIED. ) ;
#57603=ORIENTED_EDGE ( 'NONE', *, *, #22873, .T. ) ;
#57606=CARTESIAN_POINT ( 'NONE',  ( -0.001903571469574895196, -79.97561236326164646, 1.249706230131253593 ) ) ;
#57612=CARTESIAN_POINT ( 'NONE',  ( 0.04625940550791253492, -81.47683375462607103, -1.511023559015027162 ) ) ;
#57647=CARTESIAN_POINT ( 'NONE',  ( 1.092232985442823212, -78.20833333333332860, -0.6295237254636224522 ) ) ;
#57678=CARTESIAN_POINT ( 'NONE',  ( 1.223541343054339592, -81.86652669252035253, 0.2554005638053010174 ) ) ;
#57679=CARTESIAN_POINT ( 'NONE',  ( -0.8896911107955999265, -78.81702590002998932, 1.268128527205000022 ) ) ;
#57688=VERTEX_POINT ( 'NONE', #14342 ) ;
#57690=CARTESIAN_POINT ( 'NONE',  ( -0.6295237254636286695, -81.91666666666665719, 1.092232985442819881 ) ) ;
#57710=DIRECTION ( 'NONE',  ( 0.000000000000000000, 1.000000000000000000, 0.000000000000000000 ) ) ;
#57717=CARTESIAN_POINT ( 'NONE',  ( -1.251342548660999920, -81.04921328099999300, 0.5102646838515999539 ) ) ;
#57746=ADVANCED_FACE ( 'NONE', ( #35904 ), #53631, .T. ) ;
#57796=CARTESIAN_POINT ( 'NONE',  ( -0.2603338869383251541, -80.96066229293080596, -1.489115581560273460 ) ) ;
#57805=CARTESIAN_POINT ( 'NONE',  ( 1.385204701026000018, -82.86641278936299670, -0.4875042294149000144 ) ) ;
#57838=ORIENTED_EDGE ( 'NONE', *, *, #13535, .F. ) ;
#57845=CARTESIAN_POINT ( 'NONE',  ( 1.160010371456533518, -80.31977958019837160, -0.4654735999135473090 ) ) ;
#57849=B_SPLINE_CURVE_WITH_KNOTS ( 'NONE', 3,
 ( #38074, #6489, #37782, #55803, #15354, #33348, #51380, #8220, #48111, #26221, #20932, #30350, #40086, #53097, #4077, #57519, #3227, #25643 ),
 .UNSPECIFIED., .F., .F.,
 ( 4, 2, 2, 2, 2, 2, 2, 2, 4 ),
 ( 0.000000000000000000, 0.1250000000000000833, 0.2500000000000001110, 0.3750000000000000000, 0.4999999999999999445, 0.6249999999999998890, 0.7499999999999997780, 0.8749999999999998890, 1.000000000000000000 ),
 .UNSPECIFIED. ) ;
#57861=CIRCLE ( 'NONE', #53147, 9.950000000000001066 ) ;
#57866=ADVANCED_FACE ( 'NONE', ( #37363 ), #33516, .F. ) ;
#57870=CARTESIAN_POINT ( 'NONE',  ( -0.6663465976954637826, -83.01994639268885123, 1.061158757155598042 ) ) ;
#57873=CARTESIAN_POINT ( 'NONE',  ( 0.7887820451556000201, -81.72691005693999955, 1.375581554690999964 ) ) ;
#57874=CARTESIAN_POINT ( 'NONE',  ( 1.511505244404999893, -80.66777860354999063, 0.4793209935110999687 ) ) ;
#57878=CARTESIAN_POINT ( 'NONE',  ( 0.6304340365998000184, -82.55529135728299650, 1.542015542100000136 ) ) ;
#57891=CARTESIAN_POINT ( 'NONE',  ( -1.552248384014999871, -82.80004243524099650, 0.6048007385293000526 ) ) ;
#57896=CARTESIAN_POINT ( 'NONE',  ( 0.000000000000000000, -92.39999999999999147, 0.000000000000000000 ) ) ;
#57899=CARTESIAN_POINT ( 'NONE',  ( -0.01465444447223758842, -79.97640258770987032, 1.249640596461801145 ) ) ;
#57902=AXIS2_PLACEMENT_3D ( 'NONE', #52755, #21163, #33861 ) ;
#57912=VERTEX_POINT ( 'NONE', #23497 ) ;
#57922=CARTESIAN_POINT ( 'NONE',  ( -0.1638756991376206507, -82.48607747092580667, 1.249557844123856398 ) ) ;
#57926=CARTESIAN_POINT ( 'NONE',  ( -1.170441605159127318, -79.57192497548669508, 0.4385201796425973741 ) ) ;
#57928=ORIENTED_EDGE ( 'NONE', *, *, #47997, .F. ) ;
#57936=CARTESIAN_POINT ( 'NONE',  ( 0.4192948356380000186, -79.35872016573999588, -1.440205485619000081 ) ) ;
#57941=CARTESIAN_POINT ( 'NONE',  ( -0.3271848554490991434, -78.10416666666665719, -1.217465845835395299 ) ) ;
#57974=CARTESIAN_POINT ( 'NONE',  ( 1.154393885937252007, -81.88139355081031567, 0.4793241423197361351 ) ) ;
#57975=CARTESIAN_POINT ( 'NONE',  ( -0.6263700131298999274, -79.48520473737998771, -1.416660022192000046 ) ) ;
#57976=VECTOR ( 'NONE', #10612, 1000.000000000000000 ) ;
#57978=CARTESIAN_POINT ( 'NONE',  ( -1.500000000000000000, -83.24999999999998579, 0.000000000000000000 ) ) ;
#57983=CARTESIAN_POINT ( 'NONE',  ( 1.176643243505789638, -81.82277510417709721, -0.4220517775147419326 ) ) ;
#57987=CARTESIAN_POINT ( 'NONE',  ( 2.299999999264999762, -77.49999999927000260, 2.080610816276000257E-10 ) ) ;
#58037=FACE_OUTER_BOUND ( 'NONE', #25249, .T. ) ;
#58046=EDGE_CURVE ( 'NONE', #39544, #19092, #42049, .T. ) ;
#58083=CARTESIAN_POINT ( 'NONE',  ( 1.092232985442820992, -83.29166666666665719, 0.6295237254636267821 ) ) ;
#58091=CARTESIAN_POINT ( 'NONE',  ( 1.476627061896669924, -81.08212518682249481, -0.3264197646420510246 ) ) ;
#58116=DIRECTION ( 'NONE',  ( 0.7071067811865969777, -0.7071067811864980568, 6.518241473468980170E-10 ) ) ;
#58120=CARTESIAN_POINT ( 'NONE',  ( 0.9441861370063999725, -79.71587320708998448, 1.372505234203999835 ) ) ;
#58123=CARTESIAN_POINT ( 'NONE',  ( 1.250000000000000000, -78.35000000000000853, 0.000000000000000000 ) ) ;
#58135=CARTESIAN_POINT ( 'NONE',  ( 1.248120568784000017, -78.57661456821999479, 1.076606392262000167 ) ) ;
#58136=ORIENTED_EDGE ( 'NONE', *, *, #34300, .T. ) ;
#58140=CARTESIAN_POINT ( 'NONE',  ( 0.5435567983843210271, -80.26107177751177346, -1.125492201572247719 ) ) ;
#58141=CARTESIAN_POINT ( 'NONE',  ( 3.425937024882473377E-06, -77.82827182887865547, -1.422119424801547627 ) ) ;
#58164=EDGE_CURVE ( 'NONE', #57912, #31243, #25092, .T. ) ;
#58166=CARTESIAN_POINT ( 'NONE',  ( 0.6237791458550000501, -83.11657026302199824, -1.329415719495999904 ) ) ;
#58167=CARTESIAN_POINT ( 'NONE',  ( 0.4719577028681999908, -81.17336727174999567, -1.266186157272999768 ) ) ;
#58171=CARTESIAN_POINT ( 'NONE',  ( 1.531359430757999851, -82.48818925093098642, -0.6558942768039000004 ) ) ;
#58184=CARTESIAN_POINT ( 'NONE',  ( -1.458706046781999888, -81.73027866961000143, 0.8046341008317999810 ) ) ;
#58194=FACE_OUTER_BOUND ( 'NONE', #13107, .T. ) ;
#58200=CARTESIAN_POINT ( 'NONE',  ( 1.206033450961812248, -81.54768710939626430, -0.9139931269966713456 ) ) ;
#58205=EDGE_CURVE ( 'NONE', #57688, #7670, #44440, .T. ) ;
#58220=CARTESIAN_POINT ( 'NONE',  ( 0.7692036342426435969, -79.42240521102286266, 0.9862270034562748977 ) ) ;
#58271=CARTESIAN_POINT ( 'NONE',  ( 0.2845710395804645909, -81.95718609884063710, 1.217605880370489446 ) ) ;
#58272=CARTESIAN_POINT ( 'NONE',  ( 1.545390935813999889, -78.14884706267000070, 0.1070856457118000010 ) ) ;
#58274=CARTESIAN_POINT ( 'NONE',  ( -1.035861440536891553, -82.81476822920818393, -1.098648061763779937 ) ) ;
#58284=CARTESIAN_POINT ( 'NONE',  ( -0.6295237254636235624, -80.08333333333331439, -1.092232985442822990 ) ) ;
#58291=CARTESIAN_POINT ( 'NONE',  ( 1.102622140505636006, -80.38934177173996432, 0.5889613092908587699 ) ) ;
#58306=CARTESIAN_POINT ( 'NONE',  ( -1.499999999971000086, -77.75000000002998490, -1.761798912373000190E-09 ) ) ;
#58336=CARTESIAN_POINT ( 'NONE',  ( 0.000000000000000000, -87.20000000000000284, 0.000000000000000000 ) ) ;
#58343=CARTESIAN_POINT ( 'NONE',  ( 0.6295237254636211199, -82.33333333333335702, 1.092232985442824322 ) ) ;
#58388=CARTESIAN_POINT ( 'NONE',  ( -1.320768259162522273, -80.80883367555978225, 0.7383452188593548904 ) ) ;
#58399=CARTESIAN_POINT ( 'NONE',  ( 0.8470819118255000779, -81.60354343447998815, 1.477252506412999988 ) ) ;
ENDSEC;
END-ISO-10303-21;
